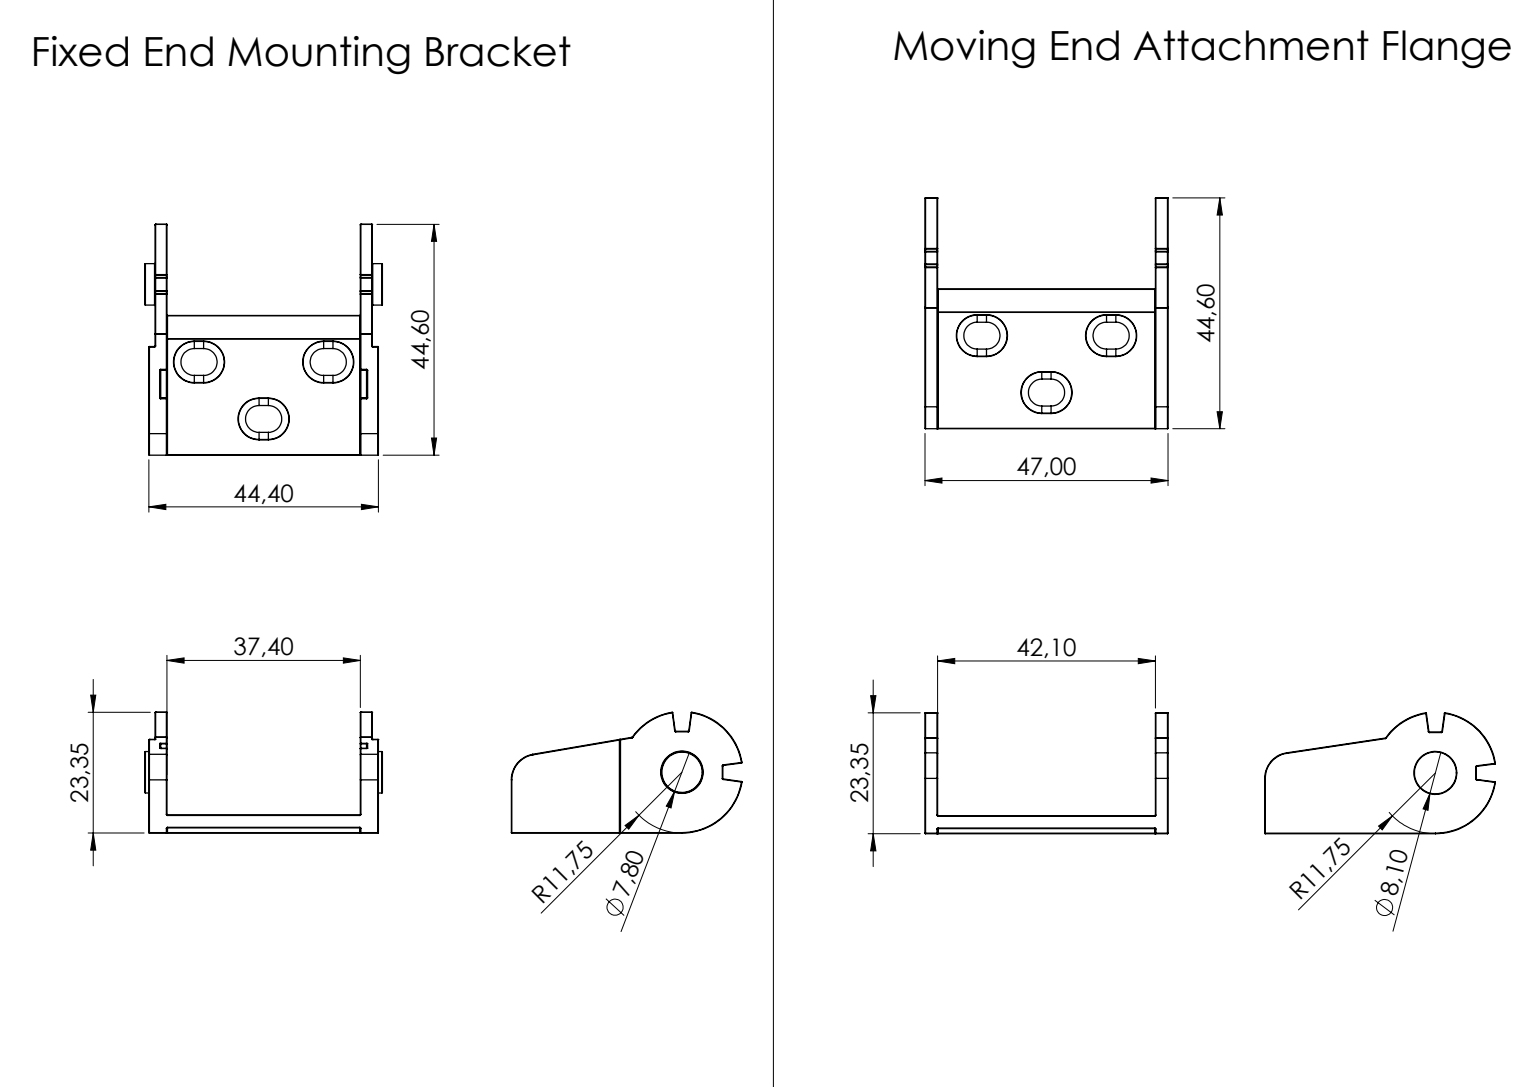
ISO-10303-21;
HEADER;
FILE_DESCRIPTION (('STEP AP214'),
    '1' );
FILE_NAME ('Moving End Attachment Flange.step',
    '2026-10-08T22:59:04',
    ( '' ),
    ( '' ),
    'SwSTEP 2.0',
    'SolidWorks 2020',
    '' );
FILE_SCHEMA (( 'AUTOMOTIVE_DESIGN' ));
ENDSEC;

DATA;
#58=DIRECTION ( 'NONE',  ( 1.000000000000000000, 0.000000000000000000, 0.000000000000000000 ) ) ;
#65=DIRECTION ( 'NONE',  ( -1.000000000000000000, 0.000000000000000000, 0.000000000000000000 ) ) ;
#86=AXIS2_PLACEMENT_3D ( 'NONE', #170578, #248783, #191400 ) ;
#130=ORIENTED_EDGE ( 'NONE', *, *, #78727, .F. ) ;
#161=CARTESIAN_POINT ( 'NONE',  ( 21.15000000000003055, 74.83745509109094485, -44.02310748452479316 ) ) ;
#188=FACE_OUTER_BOUND ( 'NONE', #64548, .T. ) ;
#229=AXIS2_PLACEMENT_3D ( 'NONE', #181398, #200936, #217905 ) ;
#283=DIRECTION ( 'NONE',  ( 1.000000000000000000, -0.000000000000000000, -0.000000000000000000 ) ) ;
#297=VERTEX_POINT ( 'NONE', #114542 ) ;
#298=DIRECTION ( 'NONE',  ( 0.000000000000000000, -0.9910827722268049644, -0.1332476588733589040 ) ) ;
#305=AXIS2_PLACEMENT_3D ( 'NONE', #200096, #237928, #219641 ) ;
#313=LINE ( 'NONE', #160718, #74675 ) ;
#317=ORIENTED_EDGE ( 'NONE', *, *, #114958, .T. ) ;
#423=CARTESIAN_POINT ( 'NONE',  ( 23.50000000000005684, 64.35000000001120668, -36.02310748452479316 ) ) ;
#432=ORIENTED_EDGE ( 'NONE', *, *, #190307, .F. ) ;
#508=AXIS2_PLACEMENT_3D ( 'NONE', #214942, #57126, #117135 ) ;
#514=VERTEX_POINT ( 'NONE', #110365 ) ;
#591=DIRECTION ( 'NONE',  ( 0.000000000000000000, -0.000000000000000000, 1.000000000000000000 ) ) ;
#608=DIRECTION ( 'NONE',  ( -1.000000000000000000, 0.000000000000000000, 0.000000000000000000 ) ) ;
#681=DIRECTION ( 'NONE',  ( 1.000000000000000000, -0.000000000000000000, -0.000000000000000000 ) ) ;
#684=DIRECTION ( 'NONE',  ( -1.000000000000000000, 0.000000000000000000, 0.000000000000000000 ) ) ;
#692=VECTOR ( 'NONE', #235400, 1000.000000000000114 ) ;
#719=EDGE_CURVE ( 'NONE', #17064, #33613, #92090, .T. ) ;
#745=FACE_OUTER_BOUND ( 'NONE', #98219, .T. ) ;
#767=ORIENTED_EDGE ( 'NONE', *, *, #253164, .T. ) ;
#781=CARTESIAN_POINT ( 'NONE',  ( 21.05000000000003979, 77.26165318615413469, -44.00978271863746016 ) ) ;
#784=CARTESIAN_POINT ( 'NONE',  ( 21.15000000000005187, 82.72707916847673459, -26.51159310135756897 ) ) ;
#789=CIRCLE ( 'NONE', #92397, 0.09999999999999939493 ) ;
#846=DIRECTION ( 'NONE',  ( 0.000000000000000000, 0.000000000000000000, 1.000000000000000000 ) ) ;
#874=DIRECTION ( 'NONE',  ( 0.000000000000000000, -1.000000000000000000, 0.000000000000000000 ) ) ;
#877=FACE_OUTER_BOUND ( 'NONE', #241147, .T. ) ;
#885=AXIS2_PLACEMENT_3D ( 'NONE', #13789, #95876, #252376 ) ;
#899=CARTESIAN_POINT ( 'NONE',  ( -23.49999999999994316, 74.83745509109094485, -44.02310748452479316 ) ) ;
#911=CARTESIAN_POINT ( 'NONE',  ( -23.39999999999994529, 84.00000000001119815, -37.18565239344504647 ) ) ;
#1008=AXIS2_PLACEMENT_3D ( 'NONE', #183384, #165097, #242056 ) ;
#1064=CARTESIAN_POINT ( 'NONE',  ( -23.49999999999994316, 83.80000000001119531, -34.86056257560453986 ) ) ;
#1099=DIRECTION ( 'NONE',  ( 0.000000000000000000, 0.000000000000000000, -1.000000000000000000 ) ) ;
#1101=DIRECTION ( 'NONE',  ( 0.000000000000000000, -0.9910827722268055195, 0.1332476588733540468 ) ) ;
#1121=EDGE_LOOP ( 'NONE', ( #113054, #182674, #33801, #198627 ) ) ;
#1192=CARTESIAN_POINT ( 'NONE',  ( 13.40000000000005898, 67.72071067812984779, -17.05239680640613997 ) ) ;
#1199=CARTESIAN_POINT ( 'NONE',  ( -20.94999999999994600, 65.25000000001119815, -51.02310748452479316 ) ) ;
#1262=EDGE_CURVE ( 'NONE', #252143, #114575, #242463, .T. ) ;
#1303=EDGE_LOOP ( 'NONE', ( #252309, #196137, #144068, #151074 ) ) ;
#1338=EDGE_CURVE ( 'NONE', #144177, #154033, #211118, .T. ) ;
#1363=CARTESIAN_POINT ( 'NONE',  ( 21.05000000000005400, 76.00000000001119815, -36.02310748452479316 ) ) ;
#1390=DIRECTION ( 'NONE',  ( -1.070660780358590712E-14, 0.9875102702516478370, -0.1575546449569727447 ) ) ;
#1441=EDGE_LOOP ( 'NONE', ( #100065, #27139, #58016, #75040 ) ) ;
#1472=LINE ( 'NONE', #118882, #221495 ) ;
#1480=DIRECTION ( 'NONE',  ( 1.000000000000000000, 0.000000000000000000, 0.000000000000000000 ) ) ;
#1489=ORIENTED_EDGE ( 'NONE', *, *, #175669, .F. ) ;
#1495=CARTESIAN_POINT ( 'NONE',  ( -20.94999999999994600, 66.25000000001114131, -51.02310748452476474 ) ) ;
#1569=VERTEX_POINT ( 'NONE', #161428 ) ;
#1588=LINE ( 'NONE', #141126, #111848 ) ;
#1647=DIRECTION ( 'NONE',  ( -0.000000000000000000, 1.000000000000000000, -0.000000000000000000 ) ) ;
#1657=VERTEX_POINT ( 'NONE', #70031 ) ;
#1673=EDGE_CURVE ( 'NONE', #28383, #222419, #249930, .T. ) ;
#1721=ORIENTED_EDGE ( 'NONE', *, *, #167214, .T. ) ;
#1726=AXIS2_PLACEMENT_3D ( 'NONE', #171029, #167159, #68024 ) ;
#1753=EDGE_CURVE ( 'NONE', #216962, #117682, #84575, .T. ) ;
#1769=EDGE_CURVE ( 'NONE', #179303, #61312, #15179, .T. ) ;
#1838=FACE_OUTER_BOUND ( 'NONE', #225196, .T. ) ;
#1881=CIRCLE ( 'NONE', #139248, 11.74999999999999645 ) ;
#1900=CYLINDRICAL_SURFACE ( 'NONE', #133191, 0.1000000000000028644 ) ;
#1940=ADVANCED_FACE ( 'NONE', ( #127099 ), #187100, .F. ) ;
#1952=ORIENTED_EDGE ( 'NONE', *, *, #205499, .F. ) ;
#2003=CARTESIAN_POINT ( 'NONE',  ( -23.49999999999994316, 64.35000000001120668, -29.92310748452479174 ) ) ;
#2010=ORIENTED_EDGE ( 'NONE', *, *, #13983, .T. ) ;
#2069=ORIENTED_EDGE ( 'NONE', *, *, #253484, .F. ) ;
#2123=DIRECTION ( 'NONE',  ( 0.000000000000000000, 0.000000000000000000, 1.000000000000000000 ) ) ;
#2254=EDGE_LOOP ( 'NONE', ( #136794, #52446, #245311, #24312 ) ) ;
#2289=EDGE_CURVE ( 'NONE', #178217, #49193, #223313, .T. ) ;
#2316=ORIENTED_EDGE ( 'NONE', *, *, #26990, .T. ) ;
#2337=ORIENTED_EDGE ( 'NONE', *, *, #212153, .F. ) ;
#2346=ORIENTED_EDGE ( 'NONE', *, *, #179917, .F. ) ;
#2425=AXIS2_PLACEMENT_3D ( 'NONE', #153513, #135160, #16531 ) ;
#2429=AXIS2_PLACEMENT_3D ( 'NONE', #151127, #230663, #191554 ) ;
#2432=CARTESIAN_POINT ( 'NONE',  ( -20.94999999999994600, 64.35000000001120668, -30.12310748452479103 ) ) ;
#2437=EDGE_CURVE ( 'NONE', #105984, #249805, #159645, .T. ) ;
#2510=CARTESIAN_POINT ( 'NONE',  ( -21.04999999999994387, 67.75000000001118394, -51.02310748452479316 ) ) ;
#2533=ORIENTED_EDGE ( 'NONE', *, *, #140585, .F. ) ;
#2552=DIRECTION ( 'NONE',  ( -1.000000000000000000, 0.000000000000000000, 0.000000000000000000 ) ) ;
#2571=DIRECTION ( 'NONE',  ( 0.000000000000000000, -1.000000000000000000, 0.000000000000000000 ) ) ;
#2592=ORIENTED_EDGE ( 'NONE', *, *, #199882, .F. ) ;
#2628=ADVANCED_FACE ( 'NONE', ( #243589 ), #18362, .F. ) ;
#2667=ORIENTED_EDGE ( 'NONE', *, *, #152205, .F. ) ;
#2698=ORIENTED_EDGE ( 'NONE', *, *, #100935, .F. ) ;
#2707=ORIENTED_EDGE ( 'NONE', *, *, #230430, .F. ) ;
#2770=ADVANCED_FACE ( 'NONE', ( #12709, #51783 ), #92205, .T. ) ;
#2806=PLANE ( 'NONE',  #25318 ) ;
#2812=EDGE_CURVE ( 'NONE', #113855, #9346, #20397, .T. ) ;
#2871=CARTESIAN_POINT ( 'NONE',  ( 21.05000000000005400, 74.16448838626246243, -47.52760213295649550 ) ) ;
#2911=AXIS2_PLACEMENT_3D ( 'NONE', #169962, #13421, #155523 ) ;
#2954=AXIS2_PLACEMENT_3D ( 'NONE', #224651, #164695, #167289 ) ;
#2988=AXIS2_PLACEMENT_3D ( 'NONE', #69678, #65800, #146600 ) ;
#3026=FACE_OUTER_BOUND ( 'NONE', #56842, .T. ) ;
#3089=EDGE_CURVE ( 'NONE', #24547, #60636, #101713, .T. ) ;
#3099=ORIENTED_EDGE ( 'NONE', *, *, #152190, .T. ) ;
#3110=LINE ( 'NONE', #183067, #153785 ) ;
#3143=DIRECTION ( 'NONE',  ( 0.000000000000000000, 0.000000000000000000, 1.000000000000000000 ) ) ;
#3193=CARTESIAN_POINT ( 'NONE',  ( -23.49999999999994316, 64.25000000001119815, -21.92310748452479174 ) ) ;
#3251=AXIS2_PLACEMENT_3D ( 'NONE', #102544, #214215, #195948 ) ;
#3256=DIRECTION ( 'NONE',  ( 1.000000000000000000, -0.000000000000000000, 0.000000000000000000 ) ) ;
#3259=VERTEX_POINT ( 'NONE', #80009 ) ;
#3263=CARTESIAN_POINT ( 'NONE',  ( -23.49999999999994316, 77.16254490893143725, -44.02310748452479316 ) ) ;
#3291=EDGE_LOOP ( 'NONE', ( #132921, #218359, #207662, #185863 ) ) ;
#3403=CARTESIAN_POINT ( 'NONE',  ( 21.15000000000005187, 83.90000000001120384, -37.27310748452479316 ) ) ;
#3418=ORIENTED_EDGE ( 'NONE', *, *, #5501, .T. ) ;
#3438=CARTESIAN_POINT ( 'NONE',  ( 6.000000000000061284, 64.65000000001120384, -22.12310748452479103 ) ) ;
#3443=EDGE_CURVE ( 'NONE', #226270, #123360, #243570, .T. ) ;
#3454=DIRECTION ( 'NONE',  ( 0.000000000000000000, 0.1332476588733589318, 0.9910827722268049644 ) ) ;
#3486=CIRCLE ( 'NONE', #149273, 0.1000000000000045852 ) ;
#3565=ORIENTED_EDGE ( 'NONE', *, *, #6376, .T. ) ;
#3574=EDGE_CURVE ( 'NONE', #35839, #131459, #32963, .T. ) ;
#3588=CARTESIAN_POINT ( 'NONE',  ( -23.49999999999994316, 82.84256550613280012, -26.34830530078816935 ) ) ;
#3592=VERTEX_POINT ( 'NONE', #115024 ) ;
#3598=CARTESIAN_POINT ( 'NONE',  ( 20.95000000000005258, 65.15000000001120384, -51.02310748452479316 ) ) ;
#3668=CARTESIAN_POINT ( 'NONE',  ( 5.551115123125782702E-14, 64.75000000001119815, -36.02310748452479316 ) ) ;
#3706=DIRECTION ( 'NONE',  ( 0.000000000000000000, -0.9910827722268055195, -0.1332476588733540468 ) ) ;
#3757=CARTESIAN_POINT ( 'NONE',  ( -20.94999999999994600, 65.15000000001120384, -3.123107484524795474 ) ) ;
#3786=CARTESIAN_POINT ( 'NONE',  ( 21.05000000000005400, 64.25000000001119815, -29.92310748452479174 ) ) ;
#3817=ORIENTED_EDGE ( 'NONE', *, *, #192515, .F. ) ;
#3832=CIRCLE ( 'NONE', #182907, 4.041421356237310469 ) ;
#3842=CIRCLE ( 'NONE', #241184, 0.09999999999999982514 ) ;
#3861=DIRECTION ( 'NONE',  ( 0.000000000000000000, 0.000000000000000000, -1.000000000000000000 ) ) ;
#3897=AXIS2_PLACEMENT_3D ( 'NONE', #95566, #57713, #237656 ) ;
#3941=ORIENTED_EDGE ( 'NONE', *, *, #226784, .F. ) ;
#4014=ADVANCED_FACE ( 'NONE', ( #179523 ), #139050, .T. ) ;
#4017=ORIENTED_EDGE ( 'NONE', *, *, #162333, .F. ) ;
#4045=CYLINDRICAL_SURFACE ( 'NONE', #163268, 0.09999999999999939493 ) ;
#4077=AXIS2_PLACEMENT_3D ( 'NONE', #31474, #53573, #110979 ) ;
#4093=DIRECTION ( 'NONE',  ( 0.000000000000000000, 0.000000000000000000, -1.000000000000000000 ) ) ;
#4096=AXIS2_PLACEMENT_3D ( 'NONE', #226436, #206904, #28301 ) ;
#4129=ORIENTED_EDGE ( 'NONE', *, *, #11231, .F. ) ;
#4148=CIRCLE ( 'NONE', #145598, 0.09999999999999939493 ) ;
#4156=CARTESIAN_POINT ( 'NONE',  ( 20.95000000000005613, 66.15000000001120384, -5.923107484524795296 ) ) ;
#4160=DIRECTION ( 'NONE',  ( 1.000000000000000000, 0.000000000000000000, 0.000000000000000000 ) ) ;
#4165=AXIS2_PLACEMENT_3D ( 'NONE', #175488, #100708, #155931 ) ;
#4169=DIRECTION ( 'NONE',  ( 0.000000000000000000, 0.000000000000000000, 1.000000000000000000 ) ) ;
#4170=DIRECTION ( 'NONE',  ( 0.000000000000000000, 0.000000000000000000, 1.000000000000000000 ) ) ;
#4173=ORIENTED_EDGE ( 'NONE', *, *, #60970, .F. ) ;
#4191=CIRCLE ( 'NONE', #204094, 0.09999999999999635569 ) ;
#4262=AXIS2_PLACEMENT_3D ( 'NONE', #181726, #124322, #42219 ) ;
#4289=CARTESIAN_POINT ( 'NONE',  ( -23.39999999999994529, 82.64476912853859858, -26.37791261425322986 ) ) ;
#4299=ORIENTED_EDGE ( 'NONE', *, *, #222834, .F. ) ;
#4303=EDGE_LOOP ( 'NONE', ( #202943, #2316, #5119, #203165, #34482, #231347, #128376, #168284, #195736, #122157, #112154, #131721, #69827, #42740, #256729, #184778, #204213, #171842 ) ) ;
#4333=DIRECTION ( 'NONE',  ( 0.000000000000000000, -0.1480365673253065117, 0.9889818879709274535 ) ) ;
#4335=CIRCLE ( 'NONE', #125175, 0.1999999999999987899 ) ;
#4427=LINE ( 'NONE', #245626, #204503 ) ;
#4449=EDGE_CURVE ( 'NONE', #168532, #177623, #63085, .T. ) ;
#4530=DIRECTION ( 'NONE',  ( 1.000000000000000000, 0.000000000000000000, 0.000000000000000000 ) ) ;
#4591=CARTESIAN_POINT ( 'NONE',  ( -21.14999999999994174, 76.00000000001119815, -36.02310748452479316 ) ) ;
#4593=DIRECTION ( 'NONE',  ( -1.000000000000000000, 0.000000000000000000, 0.000000000000000000 ) ) ;
#4675=AXIS2_PLACEMENT_3D ( 'NONE', #54422, #132692, #33632 ) ;
#4691=DIRECTION ( 'NONE',  ( -0.000000000000000000, -1.000000000000000000, 0.000000000000000000 ) ) ;
#4782=CIRCLE ( 'NONE', #221456, 0.09999999999999635569 ) ;
#4787=CARTESIAN_POINT ( 'NONE',  ( -21.14999999999994174, 83.90000000001120384, -34.77310748452479316 ) ) ;
#4835=CIRCLE ( 'NONE', #79679, 0.1000000000000021844 ) ;
#4914=CARTESIAN_POINT ( 'NONE',  ( -23.39999999999994529, 77.16254490893143725, -43.82310748452479743 ) ) ;
#5000=DIRECTION ( 'NONE',  ( 0.000000000000000000, 0.1480365673253065117, -0.9889818879709273425 ) ) ;
#5019=CARTESIAN_POINT ( 'NONE',  ( -21.14999999999994174, 87.51781941433023349, -37.75951082105083145 ) ) ;
#5026=DIRECTION ( 'NONE',  ( -0.000000000000000000, 0.000000000000000000, 1.000000000000000000 ) ) ;
#5035=DIRECTION ( 'NONE',  ( -1.284434275755705296E-16, 0.7071067811865471286, -0.7071067811865479058 ) ) ;
#5048=DIRECTION ( 'NONE',  ( 1.000000000000000000, 0.000000000000000000, 0.000000000000000000 ) ) ;
#5067=LINE ( 'NONE', #45514, #195066 ) ;
#5119=ORIENTED_EDGE ( 'NONE', *, *, #1753, .F. ) ;
#5137=DIRECTION ( 'NONE',  ( 1.000000000000000000, 0.000000000000000000, 0.000000000000000000 ) ) ;
#5177=DIRECTION ( 'NONE',  ( 0.000000000000000000, 0.000000000000000000, 1.000000000000000000 ) ) ;
#5205=AXIS2_PLACEMENT_3D ( 'NONE', #2510, #202017, #20831 ) ;
#5207=VERTEX_POINT ( 'NONE', #162901 ) ;
#5251=DIRECTION ( 'NONE',  ( 1.000000000000000000, 0.000000000000000000, 0.000000000000000000 ) ) ;
#5309=CARTESIAN_POINT ( 'NONE',  ( -13.39999999999994529, 64.35000000001120668, -18.32310748452479388 ) ) ;
#5311=DIRECTION ( 'NONE',  ( 0.000000000000000000, 1.000000000000000000, 0.000000000000000000 ) ) ;
#5356=ORIENTED_EDGE ( 'NONE', *, *, #92045, .T. ) ;
#5376=ORIENTED_EDGE ( 'NONE', *, *, #101397, .F. ) ;
#5436=ORIENTED_EDGE ( 'NONE', *, *, #13960, .T. ) ;
#5487=VECTOR ( 'NONE', #95802, 1000.000000000000000 ) ;
#5491=ORIENTED_EDGE ( 'NONE', *, *, #140323, .T. ) ;
#5501=EDGE_CURVE ( 'NONE', #118363, #143932, #44230, .T. ) ;
#5523=ORIENTED_EDGE ( 'NONE', *, *, #39101, .F. ) ;
#5527=ORIENTED_EDGE ( 'NONE', *, *, #208102, .F. ) ;
#5534=EDGE_CURVE ( 'NONE', #81245, #109039, #143949, .T. ) ;
#5588=AXIS2_PLACEMENT_3D ( 'NONE', #65713, #188233, #109969 ) ;
#5596=DIRECTION ( 'NONE',  ( 0.000000000000000000, 0.000000000000000000, 1.000000000000000000 ) ) ;
#5681=ORIENTED_EDGE ( 'NONE', *, *, #75557, .T. ) ;
#5698=ORIENTED_EDGE ( 'NONE', *, *, #205981, .F. ) ;
#5797=EDGE_LOOP ( 'NONE', ( #16794, #21298, #95358, #113360 ) ) ;
#5858=CIRCLE ( 'NONE', #30852, 0.09999999999999939493 ) ;
#5874=CARTESIAN_POINT ( 'NONE',  ( -5.899999999999938183, 64.65000000001120384, -22.12310748452479103 ) ) ;
#5887=VECTOR ( 'NONE', #138797, 1000.000000000000000 ) ;
#5945=ORIENTED_EDGE ( 'NONE', *, *, #220027, .F. ) ;
#5948=CARTESIAN_POINT ( 'NONE',  ( 11.60000000000006182, 66.35000000001119247, -18.42310748452479530 ) ) ;
#6019=ORIENTED_EDGE ( 'NONE', *, *, #64587, .T. ) ;
#6034=DIRECTION ( 'NONE',  ( 1.000000000000000000, 0.000000000000000000, 0.000000000000000000 ) ) ;
#6060=DIRECTION ( 'NONE',  ( 3.469446951953515108E-14, 0.000000000000000000, 1.000000000000000000 ) ) ;
#6077=AXIS2_PLACEMENT_3D ( 'NONE', #129564, #249515, #126983 ) ;
#6102=CARTESIAN_POINT ( 'NONE',  ( 20.95000000000005969, 61.72892516158560028, -36.56695479651062897 ) ) ;
#6134=EDGE_CURVE ( 'NONE', #166555, #204034, #173245, .T. ) ;
#6163=LINE ( 'NONE', #129650, #109600 ) ;
#6179=ORIENTED_EDGE ( 'NONE', *, *, #223678, .F. ) ;
#6253=EDGE_CURVE ( 'NONE', #109234, #200341, #151252, .T. ) ;
#6254=ORIENTED_EDGE ( 'NONE', *, *, #244093, .T. ) ;
#6284=CARTESIAN_POINT ( 'NONE',  ( -21.04999999999994387, 67.75000000001118394, -3.123107484524795474 ) ) ;
#6318=CARTESIAN_POINT ( 'NONE',  ( -23.49999999999994316, 83.90000000001120384, -34.77310748452479316 ) ) ;
#6339=CARTESIAN_POINT ( 'NONE',  ( -23.49999999999994316, 77.83551161375991967, -47.52760213295649550 ) ) ;
#6376=EDGE_CURVE ( 'NONE', #131459, #210784, #186243, .T. ) ;
#6397=FACE_OUTER_BOUND ( 'NONE', #98533, .T. ) ;
#6464=FACE_OUTER_BOUND ( 'NONE', #103057, .T. ) ;
#6487=VERTEX_POINT ( 'NONE', #119836 ) ;
#6491=EDGE_CURVE ( 'NONE', #88642, #28434, #23384, .T. ) ;
#6566=CIRCLE ( 'NONE', #102390, 0.1000000000000028644 ) ;
#6567=CARTESIAN_POINT ( 'NONE',  ( -23.49999999999994316, 87.50449464844290048, -37.85861909827351468 ) ) ;
#6577=ORIENTED_EDGE ( 'NONE', *, *, #18649, .T. ) ;
#6652=SPHERICAL_SURFACE ( 'NONE', #72367, 0.1000000000000000056 ) ;
#6663=CARTESIAN_POINT ( 'NONE',  ( -23.49999999999994316, 77.73640333653723644, -47.54092689884382850 ) ) ;
#6726=AXIS2_PLACEMENT_3D ( 'NONE', #63550, #141802, #183513 ) ;
#6800=VECTOR ( 'NONE', #177965, 1000.000000000000000 ) ;
#6839=ORIENTED_EDGE ( 'NONE', *, *, #254228, .F. ) ;
#6859=CARTESIAN_POINT ( 'NONE',  ( -13.39999999999994351, 64.25000000001119815, -23.72310748452479245 ) ) ;
#6881=LINE ( 'NONE', #186825, #76412 ) ;
#6904=CARTESIAN_POINT ( 'NONE',  ( 21.15000000000005187, 64.25000000001119815, -36.02310748452479316 ) ) ;
#6932=ORIENTED_EDGE ( 'NONE', *, *, #243618, .F. ) ;
#6944=ORIENTED_EDGE ( 'NONE', *, *, #59147, .T. ) ;
#6947=ORIENTED_EDGE ( 'NONE', *, *, #242302, .T. ) ;
#6953=VERTEX_POINT ( 'NONE', #104705 ) ;
#6987=DIRECTION ( 'NONE',  ( 0.000000000000000000, 1.000000000000000000, -1.224646799147352961E-16 ) ) ;
#7009=DIRECTION ( 'NONE',  ( 0.000000000000000000, 0.000000000000000000, 1.000000000000000000 ) ) ;
#7097=CARTESIAN_POINT ( 'NONE',  ( -23.49999999999994316, 89.48413628383013929, -38.12477508515532065 ) ) ;
#7122=AXIS2_PLACEMENT_3D ( 'NONE', #137369, #257277, #96934 ) ;
#7186=ADVANCED_FACE ( 'NONE', ( #238827 ), #58872, .T. ) ;
#7195=ADVANCED_FACE ( 'NONE', ( #120200 ), #15957, .T. ) ;
#7211=FACE_OUTER_BOUND ( 'NONE', #182132, .T. ) ;
#7234=CARTESIAN_POINT ( 'NONE',  ( 23.40000000000005542, 64.25000000001119815, -43.82310748452479743 ) ) ;
#7255=ORIENTED_EDGE ( 'NONE', *, *, #152151, .F. ) ;
#7370=LINE ( 'NONE', #204278, #172996 ) ;
#7377=ORIENTED_EDGE ( 'NONE', *, *, #142662, .F. ) ;
#7384=CIRCLE ( 'NONE', #153185, 0.09999999999999939493 ) ;
#7407=CARTESIAN_POINT ( 'NONE',  ( 21.05000000000005400, 79.78873604695631627, -7.297728304630792806 ) ) ;
#7463=ORIENTED_EDGE ( 'NONE', *, *, #65270, .T. ) ;
#7555=FACE_OUTER_BOUND ( 'NONE', #97491, .T. ) ;
#7567=ORIENTED_EDGE ( 'NONE', *, *, #44290, .T. ) ;
#7576=AXIS2_PLACEMENT_3D ( 'NONE', #228645, #26588, #203917 ) ;
#7626=DIRECTION ( 'NONE',  ( 0.000000000000000000, 0.1332476588733448597, 0.9910827722268067408 ) ) ;
#7661=AXIS2_PLACEMENT_3D ( 'NONE', #125665, #87803, #167395 ) ;
#7714=TOROIDAL_SURFACE ( 'NONE', #20182, 4.150000000000000355, 0.1000000000000000056 ) ;
#7804=CARTESIAN_POINT ( 'NONE',  ( -21.14999999999994174, 76.00000000001119815, -36.02310748452479316 ) ) ;
#7807=DIRECTION ( 'NONE',  ( -1.000000000000000000, 0.000000000000000000, 0.000000000000000000 ) ) ;
#7832=ORIENTED_EDGE ( 'NONE', *, *, #196051, .F. ) ;
#7836=ADVANCED_FACE ( 'NONE', ( #182412 ), #132225, .T. ) ;
#7879=ORIENTED_EDGE ( 'NONE', *, *, #155408, .F. ) ;
#7893=DIRECTION ( 'NONE',  ( -1.000000000000000000, -0.000000000000000000, -0.000000000000000000 ) ) ;
#7939=CARTESIAN_POINT ( 'NONE',  ( 5.900000000000059863, 64.65000000001120384, -25.92310748452479174 ) ) ;
#7988=VECTOR ( 'NONE', #37090, 1000.000000000000114 ) ;
#7990=ADVANCED_FACE ( 'NONE', ( #176985 ), #53150, .F. ) ;
#8064=CARTESIAN_POINT ( 'NONE',  ( 6.000000000000060396, 64.25000000001119815, -25.92310748452479174 ) ) ;
#8187=DIRECTION ( 'NONE',  ( 0.000000000000000000, 0.000000000000000000, -1.000000000000000000 ) ) ;
#8191=DIRECTION ( 'NONE',  ( 1.000000000000000000, -0.000000000000000000, -0.000000000000000000 ) ) ;
#8217=VERTEX_POINT ( 'NONE', #48989 ) ;
#8218=SHAPE_REPRESENTATION_RELATIONSHIP ( 'NONE' , 'NONE' ,  #133560, #200717 ) ;
#8249=ORIENTED_EDGE ( 'NONE', *, *, #204291, .F. ) ;
#8251=ORIENTED_EDGE ( 'NONE', *, *, #19825, .F. ) ;
#8336=CIRCLE ( 'NONE', #154110, 4.041421356237310469 ) ;
#8399=FACE_OUTER_BOUND ( 'NONE', #57955, .T. ) ;
#8423=ORIENTED_EDGE ( 'NONE', *, *, #165404, .T. ) ;
#8429=FACE_OUTER_BOUND ( 'NONE', #91879, .T. ) ;
#8441=ORIENTED_EDGE ( 'NONE', *, *, #6376, .F. ) ;
#8457=AXIS2_PLACEMENT_3D ( 'NONE', #82873, #102439, #24248 ) ;
#8462=EDGE_LOOP ( 'NONE', ( #194088, #90251, #198660, #143089 ) ) ;
#8469=ORIENTED_EDGE ( 'NONE', *, *, #62876, .F. ) ;
#8539=DIRECTION ( 'NONE',  ( 0.000000000000000000, 2.775557561562812086E-13, 1.000000000000000000 ) ) ;
#8561=CIRCLE ( 'NONE', #16952, 0.1000000000000021844 ) ;
#8569=DIRECTION ( 'NONE',  ( 0.000000000000000000, 0.000000000000000000, 1.000000000000000000 ) ) ;
#8584=CARTESIAN_POINT ( 'NONE',  ( 21.05000000000005400, 82.72707916847673459, -26.51159310135756897 ) ) ;
#8596=CARTESIAN_POINT ( 'NONE',  ( -23.49999999999994316, 77.85126707825561709, -47.62635315998165453 ) ) ;
#8652=CARTESIAN_POINT ( 'NONE',  ( -13.39999999999994529, 67.65000000001118963, -16.98168612828748181 ) ) ;
#8670=CARTESIAN_POINT ( 'NONE',  ( -21.04999999999994387, 87.50449464844290048, -34.18759587077607165 ) ) ;
#8675=DIRECTION ( 'NONE',  ( -1.000000000000000000, 0.000000000000000000, 0.000000000000000000 ) ) ;
#8676=ORIENTED_EDGE ( 'NONE', *, *, #190134, .F. ) ;
#8683=FACE_OUTER_BOUND ( 'NONE', #14893, .T. ) ;
#8784=ORIENTED_EDGE ( 'NONE', *, *, #137079, .T. ) ;
#8835=ORIENTED_EDGE ( 'NONE', *, *, #46738, .T. ) ;
#8920=AXIS2_PLACEMENT_3D ( 'NONE', #232601, #90481, #248284 ) ;
#8939=LINE ( 'NONE', #164169, #155031 ) ;
#8971=CARTESIAN_POINT ( 'NONE',  ( 21.05000000000005400, 67.65000000001118963, -25.06452884076209742 ) ) ;
#8988=ORIENTED_EDGE ( 'NONE', *, *, #141241, .T. ) ;
#9117=EDGE_LOOP ( 'NONE', ( #16086, #23583, #36112, #191588 ) ) ;
#9165=CARTESIAN_POINT ( 'NONE',  ( -5.999999999999938716, 64.75000000001119815, -25.92310748452479174 ) ) ;
#9189=CIRCLE ( 'NONE', #217443, 0.1000000000000028644 ) ;
#9211=AXIS2_PLACEMENT_3D ( 'NONE', #172868, #77537, #257425 ) ;
#9233=ORIENTED_EDGE ( 'NONE', *, *, #179815, .T. ) ;
#9244=SPHERICAL_SURFACE ( 'NONE', #225558, 0.1000000000000000056 ) ;
#9290=ORIENTED_EDGE ( 'NONE', *, *, #13159, .T. ) ;
#9297=FACE_OUTER_BOUND ( 'NONE', #214035, .T. ) ;
#9304=DIRECTION ( 'NONE',  ( -0.000000000000000000, 0.9910827722268037432, 0.1332476588733682299 ) ) ;
#9319=CYLINDRICAL_SURFACE ( 'NONE', #147477, 0.09999999999999982514 ) ;
#9334=ADVANCED_FACE ( 'NONE', ( #163857, #162586 ), #99990, .T. ) ;
#9346=VERTEX_POINT ( 'NONE', #183421 ) ;
#9371=CARTESIAN_POINT ( 'NONE',  ( -23.39999999999994529, 64.25000000001119815, -36.02310748452479316 ) ) ;
#9389=VERTEX_POINT ( 'NONE', #127292 ) ;
#9410=ORIENTED_EDGE ( 'NONE', *, *, #246327, .F. ) ;
#9439=DIRECTION ( 'NONE',  ( 0.000000000000000000, 0.9910827722268042983, 0.1332476588733650935 ) ) ;
#9468=AXIS2_PLACEMENT_3D ( 'NONE', #110669, #72861, #148520 ) ;
#9479=ORIENTED_EDGE ( 'NONE', *, *, #226367, .T. ) ;
#9491=DIRECTION ( 'NONE',  ( 1.000000000000000000, 0.000000000000000000, 0.000000000000000000 ) ) ;
#9494=CARTESIAN_POINT ( 'NONE',  ( -40.23850191057533010, 61.64150943397345372, -36.51839050339276582 ) ) ;
#9533=ORIENTED_EDGE ( 'NONE', *, *, #49799, .T. ) ;
#9552=CARTESIAN_POINT ( 'NONE',  ( 23.50000000000005684, 84.00000000001119815, -34.86056257560453986 ) ) ;
#9575=CARTESIAN_POINT ( 'NONE',  ( -23.49999999999994316, 76.00000000001119815, -36.02310748452479316 ) ) ;
#9586=ORIENTED_EDGE ( 'NONE', *, *, #186080, .F. ) ;
#9589=DIRECTION ( 'NONE',  ( 0.000000000000000000, 0.9875102702516471709, 0.1575546449569757979 ) ) ;
#9621=CARTESIAN_POINT ( 'NONE',  ( 21.05000000000005400, 84.00000000001119815, -34.86056257560453986 ) ) ;
#9633=ORIENTED_EDGE ( 'NONE', *, *, #3443, .T. ) ;
#9637=EDGE_CURVE ( 'NONE', #143490, #186471, #124962, .T. ) ;
#9798=ORIENTED_EDGE ( 'NONE', *, *, #74787, .T. ) ;
#9836=TOROIDAL_SURFACE ( 'NONE', #147213, 0.2000000000000000111, 0.1000000000000000056 ) ;
#9838=ORIENTED_EDGE ( 'NONE', *, *, #147461, .F. ) ;
#9898=ORIENTED_EDGE ( 'NONE', *, *, #85489, .T. ) ;
#9937=CARTESIAN_POINT ( 'NONE',  ( -21.14999999999994174, 74.63923853664559260, -43.99645795275012006 ) ) ;
#10006=DIRECTION ( 'NONE',  ( 0.000000000000000000, 0.000000000000000000, -1.000000000000000000 ) ) ;
#10047=VERTEX_POINT ( 'NONE', #118902 ) ;
#10142=FACE_OUTER_BOUND ( 'NONE', #252352, .T. ) ;
#10157=VECTOR ( 'NONE', #85979, 1000.000000000000000 ) ;
#10224=CARTESIAN_POINT ( 'NONE',  ( -5.999999999999938716, 64.65000000001120384, -25.92310748452479174 ) ) ;
#10230=ORIENTED_EDGE ( 'NONE', *, *, #225434, .T. ) ;
#10234=CIRCLE ( 'NONE', #218863, 0.1000000000000032391 ) ;
#10258=CARTESIAN_POINT ( 'NONE',  ( 21.15000000000005542, 64.35000000001120668, -3.023107484524792277 ) ) ;
#10259=CARTESIAN_POINT ( 'NONE',  ( -21.14999999999994174, 77.25000000001119815, -43.92310748452479885 ) ) ;
#10282=VECTOR ( 'NONE', #105529, 1000.000000000000000 ) ;
#10351=CARTESIAN_POINT ( 'NONE',  ( -23.39999999999994529, 79.78873604695631627, -7.297728304630792806 ) ) ;
#10391=FACE_OUTER_BOUND ( 'NONE', #232579, .T. ) ;
#10448=ORIENTED_EDGE ( 'NONE', *, *, #61513, .F. ) ;
#10581=EDGE_CURVE ( 'NONE', #216036, #53024, #100773, .T. ) ;
#10605=VERTEX_POINT ( 'NONE', #5019 ) ;
#10610=EDGE_LOOP ( 'NONE', ( #69076, #190839, #236443, #253146 ) ) ;
#10848=DIRECTION ( 'NONE',  ( 0.000000000000000000, 0.000000000000000000, 1.000000000000000000 ) ) ;
#10888=PLANE ( 'NONE',  #186697 ) ;
#10915=CARTESIAN_POINT ( 'NONE',  ( -23.39999999999994529, 76.00000000001119815, -36.02310748452479316 ) ) ;
#10936=CARTESIAN_POINT ( 'NONE',  ( 21.15000000000005542, 83.97335046823651794, -37.38386894789040582 ) ) ;
#10948=DIRECTION ( 'NONE',  ( 0.000000000000000000, 0.000000000000000000, -1.000000000000000000 ) ) ;
#10959=ORIENTED_EDGE ( 'NONE', *, *, #249561, .F. ) ;
#10977=VECTOR ( 'NONE', #23732, 999.9999999999998863 ) ;
#11001=ADVANCED_FACE ( 'NONE', ( #85519 ), #245924, .T. ) ;
#11052=DIRECTION ( 'NONE',  ( 1.734723475976817823E-14, 1.000000000000000000, -0.000000000000000000 ) ) ;
#11068=ADVANCED_FACE ( 'NONE', ( #202934 ), #127255, .T. ) ;
#11093=ORIENTED_EDGE ( 'NONE', *, *, #257916, .T. ) ;
#11100=CYLINDRICAL_SURFACE ( 'NONE', #203103, 0.09999999999999939493 ) ;
#11109=VECTOR ( 'NONE', #240581, 1000.000000000000114 ) ;
#11165=DIRECTION ( 'NONE',  ( -3.469446951953515108E-14, 0.000000000000000000, -1.000000000000000000 ) ) ;
#11178=LINE ( 'NONE', #69885, #101275 ) ;
#11227=CARTESIAN_POINT ( 'NONE',  ( 21.05000000000005400, 76.00000000001119815, -36.02310748452479316 ) ) ;
#11231=EDGE_CURVE ( 'NONE', #49193, #147247, #254837, .T. ) ;
#11253=DIRECTION ( 'NONE',  ( -1.000000000000000000, 0.000000000000000000, -0.000000000000000000 ) ) ;
#11296=CARTESIAN_POINT ( 'NONE',  ( -40.23850191057533010, 67.65000000001118963, -25.49719488170504533 ) ) ;
#11488=CARTESIAN_POINT ( 'NONE',  ( 23.40000000000005542, 87.50449464844290048, -37.85861909827351468 ) ) ;
#11531=ORIENTED_EDGE ( 'NONE', *, *, #94855, .T. ) ;
#11539=DIRECTION ( 'NONE',  ( -0.000000000000000000, 0.1480365673253065117, -0.9889818879709273425 ) ) ;
#11638=CARTESIAN_POINT ( 'NONE',  ( -5.899999999999938183, 64.65000000001120384, -26.02310748452479316 ) ) ;
#11704=ORIENTED_EDGE ( 'NONE', *, *, #140585, .T. ) ;
#11710=DIRECTION ( 'NONE',  ( 0.000000000000000000, 1.000000000000000000, 0.000000000000000000 ) ) ;
#11717=ORIENTED_EDGE ( 'NONE', *, *, #152190, .F. ) ;
#11762=ADVANCED_FACE ( 'NONE', ( #45498 ), #46767, .T. ) ;
#11779=CIRCLE ( 'NONE', #174110, 2.699999999999999289 ) ;
#11786=ORIENTED_EDGE ( 'NONE', *, *, #250558, .T. ) ;
#11792=AXIS2_PLACEMENT_3D ( 'NONE', #47207, #146317, #126764 ) ;
#11824=AXIS2_PLACEMENT_3D ( 'NONE', #82317, #241436, #4093 ) ;
#11841=ORIENTED_EDGE ( 'NONE', *, *, #33972, .F. ) ;
#11846=DIRECTION ( 'NONE',  ( 0.000000000000000000, 2.775557561562812086E-13, 1.000000000000000000 ) ) ;
#11891=CIRCLE ( 'NONE', #207517, 0.09999999999999939493 ) ;
#11916=LINE ( 'NONE', #169724, #118260 ) ;
#11972=VERTEX_POINT ( 'NONE', #174491 ) ;
#11987=EDGE_LOOP ( 'NONE', ( #236841, #230235, #218852, #15222 ) ) ;
#11995=AXIS2_PLACEMENT_3D ( 'NONE', #94146, #254481, #172453 ) ;
#12025=EDGE_LOOP ( 'NONE', ( #138536, #106594, #133117, #116553 ) ) ;
#12036=ORIENTED_EDGE ( 'NONE', *, *, #42241, .F. ) ;
#12057=CARTESIAN_POINT ( 'NONE',  ( 21.05000000000005400, 87.75000000001119815, -43.82310748452479743 ) ) ;
#12090=CIRCLE ( 'NONE', #150118, 0.1000000000000028644 ) ;
#12117=CIRCLE ( 'NONE', #45402, 4.049999999999998046 ) ;
#12135=DIRECTION ( 'NONE',  ( 0.000000000000000000, 0.000000000000000000, -1.000000000000000000 ) ) ;
#12138=DIRECTION ( 'NONE',  ( 0.000000000000000000, 0.000000000000000000, 1.000000000000000000 ) ) ;
#12172=CARTESIAN_POINT ( 'NONE',  ( -23.49999999999994316, 76.00000000001119815, -31.87310748452479459 ) ) ;
#12178=DIRECTION ( 'NONE',  ( 1.000000000000000000, -0.000000000000000000, -0.000000000000000000 ) ) ;
#12197=VERTEX_POINT ( 'NONE', #88129 ) ;
#12214=VERTEX_POINT ( 'NONE', #105117 ) ;
#12239=EDGE_CURVE ( 'NONE', #35839, #74847, #89074, .T. ) ;
#12240=AXIS2_PLACEMENT_3D ( 'NONE', #105737, #223138, #44522 ) ;
#12281=PLANE ( 'NONE',  #68683 ) ;
#12282=DIRECTION ( 'NONE',  ( 0.000000000000000000, 0.000000000000000000, -1.000000000000000000 ) ) ;
#12360=EDGE_LOOP ( 'NONE', ( #119536, #155518, #179823 ) ) ;
#12388=DIRECTION ( 'NONE',  ( -1.000000000000000000, 0.000000000000000000, 0.000000000000000000 ) ) ;
#12524=CIRCLE ( 'NONE', #245736, 0.09999999999999939493 ) ;
#12539=VERTEX_POINT ( 'NONE', #87836 ) ;
#12634=ORIENTED_EDGE ( 'NONE', *, *, #33176, .T. ) ;
#12659=EDGE_CURVE ( 'NONE', #17064, #88829, #105988, .T. ) ;
#12665=ORIENTED_EDGE ( 'NONE', *, *, #236566, .F. ) ;
#12679=ORIENTED_EDGE ( 'NONE', *, *, #224280, .T. ) ;
#12682=ORIENTED_EDGE ( 'NONE', *, *, #24841, .T. ) ;
#12695=ADVANCED_FACE ( 'NONE', ( #248225 ), #229940, .T. ) ;
#12709=FACE_BOUND ( 'NONE', #159419, .T. ) ;
#12741=CARTESIAN_POINT ( 'NONE',  ( -20.94999999999994600, 64.35000000001120668, -30.02310748452479316 ) ) ;
#12755=LINE ( 'NONE', #210930, #212322 ) ;
#12764=CIRCLE ( 'NONE', #183430, 0.1000000000000028644 ) ;
#12771=CARTESIAN_POINT ( 'NONE',  ( 5.900000000000060751, 64.35000000001120668, -22.02310748452479316 ) ) ;
#12772=ORIENTED_EDGE ( 'NONE', *, *, #257916, .F. ) ;
#12805=DIRECTION ( 'NONE',  ( 0.000000000000000000, 1.000000000000000000, 0.000000000000000000 ) ) ;
#12851=AXIS2_PLACEMENT_3D ( 'NONE', #70539, #127920, #228307 ) ;
#12912=DIRECTION ( 'NONE',  ( 4.336808689942017736E-16, -0.000000000000000000, 1.000000000000000000 ) ) ;
#12936=AXIS2_PLACEMENT_3D ( 'NONE', #190065, #90955, #170556 ) ;
#12981=CARTESIAN_POINT ( 'NONE',  ( -20.94999999999994245, 67.85000000001119247, -51.02310748452479316 ) ) ;
#13015=DIRECTION ( 'NONE',  ( 0.000000000000000000, -0.1332476588733448597, -0.9910827722268067408 ) ) ;
#13048=DIRECTION ( 'NONE',  ( -0.000000000000000000, 1.000000000000000000, -0.000000000000000000 ) ) ;
#13087=DIRECTION ( 'NONE',  ( -1.000000000000000000, 0.000000000000000000, 0.000000000000000000 ) ) ;
#13122=ADVANCED_FACE ( 'NONE', ( #9297 ), #50966, .T. ) ;
#13148=CYLINDRICAL_SURFACE ( 'NONE', #232670, 0.09999999999999939493 ) ;
#13159=EDGE_CURVE ( 'NONE', #205114, #30110, #88858, .T. ) ;
#13224=CARTESIAN_POINT ( 'NONE',  ( -13.39999999999994351, 66.35000000001119247, -23.62310748452479103 ) ) ;
#13230=DIRECTION ( 'NONE',  ( -1.000000000000000000, 0.000000000000000000, 0.000000000000000000 ) ) ;
#13239=CARTESIAN_POINT ( 'NONE',  ( 21.15000000000005187, 82.84256550613280012, -26.34830530078816935 ) ) ;
#13264=ORIENTED_EDGE ( 'NONE', *, *, #147746, .F. ) ;
#13355=ORIENTED_EDGE ( 'NONE', *, *, #50686, .F. ) ;
#13376=CARTESIAN_POINT ( 'NONE',  ( -21.14999999999994174, 83.97335046823651794, -37.38386894789040582 ) ) ;
#13421=DIRECTION ( 'NONE',  ( 1.000000000000000000, -0.000000000000000000, -0.000000000000000000 ) ) ;
#13543=AXIS2_PLACEMENT_3D ( 'NONE', #96349, #152532, #175939 ) ;
#13662=DIRECTION ( 'NONE',  ( 0.000000000000000000, 0.000000000000000000, 1.000000000000000000 ) ) ;
#13672=CARTESIAN_POINT ( 'NONE',  ( 13.40000000000005898, 64.35000000001120668, -21.02310748452479316 ) ) ;
#13705=ORIENTED_EDGE ( 'NONE', *, *, #155750, .T. ) ;
#13752=DIRECTION ( 'NONE',  ( 1.000000000000000000, 0.000000000000000000, 0.000000000000000000 ) ) ;
#13756=VECTOR ( 'NONE', #184747, 1000.000000000000000 ) ;
#13774=CARTESIAN_POINT ( 'NONE',  ( 13.40000000000005720, 64.25000000001119815, -18.32310748452480098 ) ) ;
#13789=CARTESIAN_POINT ( 'NONE',  ( 13.40000000000005898, 64.35000000001120668, -21.02310748452479316 ) ) ;
#13796=ORIENTED_EDGE ( 'NONE', *, *, #138506, .T. ) ;
#13811=CIRCLE ( 'NONE', #109841, 0.09999999999999939493 ) ;
#13830=DIRECTION ( 'NONE',  ( 0.000000000000000000, 0.9910827722268055195, 0.1332476588733540468 ) ) ;
#13870=AXIS2_PLACEMENT_3D ( 'NONE', #130521, #117070, #90100 ) ;
#13905=AXIS2_PLACEMENT_3D ( 'NONE', #122932, #88592, #202463 ) ;
#13909=DIRECTION ( 'NONE',  ( 0.000000000000000000, 0.000000000000000000, -1.000000000000000000 ) ) ;
#13960=EDGE_CURVE ( 'NONE', #224235, #92271, #196928, .T. ) ;
#13983=EDGE_CURVE ( 'NONE', #248236, #192885, #135201, .T. ) ;
#14023=CARTESIAN_POINT ( 'NONE',  ( -21.14999999999994174, 74.94272479589878344, -3.023107484524792277 ) ) ;
#14046=ORIENTED_EDGE ( 'NONE', *, *, #174401, .F. ) ;
#14054=ORIENTED_EDGE ( 'NONE', *, *, #75636, .F. ) ;
#14055=AXIS2_PLACEMENT_3D ( 'NONE', #134334, #135623, #211329 ) ;
#14081=CARTESIAN_POINT ( 'NONE',  ( -13.39999999999994529, 67.75000000001118394, -16.98168612828748181 ) ) ;
#14126=DIRECTION ( 'NONE',  ( 0.000000000000000000, -0.9910827722268055195, -0.1332476588733540468 ) ) ;
#14135=ORIENTED_EDGE ( 'NONE', *, *, #253187, .T. ) ;
#14155=LINE ( 'NONE', #254007, #53938 ) ;
#14257=ORIENTED_EDGE ( 'NONE', *, *, #42522, .T. ) ;
#14293=CYLINDRICAL_SURFACE ( 'NONE', #69639, 0.09999999999999982514 ) ;
#14315=CYLINDRICAL_SURFACE ( 'NONE', #2954, 0.09999999999999939493 ) ;
#14340=ORIENTED_EDGE ( 'NONE', *, *, #213756, .T. ) ;
#14416=AXIS2_PLACEMENT_3D ( 'NONE', #205276, #127041, #103597 ) ;
#14472=CARTESIAN_POINT ( 'NONE',  ( -23.39999999999994529, 74.83745509109094485, -43.92310748452479885 ) ) ;
#14536=ORIENTED_EDGE ( 'NONE', *, *, #142536, .T. ) ;
#14572=ORIENTED_EDGE ( 'NONE', *, *, #71480, .F. ) ;
#14593=EDGE_LOOP ( 'NONE', ( #37242, #15404, #132835, #91312 ) ) ;
#14601=EDGE_LOOP ( 'NONE', ( #47038, #174680, #215860, #23375 ) ) ;
#14679=EDGE_CURVE ( 'NONE', #45216, #17064, #85007, .T. ) ;
#14693=DIRECTION ( 'NONE',  ( 1.000000000000000000, 0.000000000000000000, -0.000000000000000000 ) ) ;
#14715=CARTESIAN_POINT ( 'NONE',  ( 0.9000000000000547562, 64.35000000001120668, -10.02310748452479139 ) ) ;
#14764=CARTESIAN_POINT ( 'NONE',  ( -21.04999999999994387, 64.35000000001120668, -30.12310748452479103 ) ) ;
#14802=FACE_OUTER_BOUND ( 'NONE', #142238, .T. ) ;
#14806=DIRECTION ( 'NONE',  ( -1.000000000000000000, -0.000000000000000000, 0.000000000000000000 ) ) ;
#14829=VERTEX_POINT ( 'NONE', #30214 ) ;
#14843=DIRECTION ( 'NONE',  ( 0.000000000000000000, 0.000000000000000000, 1.000000000000000000 ) ) ;
#14876=LINE ( 'NONE', #249622, #248009 ) ;
#14882=DIRECTION ( 'NONE',  ( -0.000000000000000000, 0.9910827722268049644, -0.1332476588733589318 ) ) ;
#14893=EDGE_LOOP ( 'NONE', ( #61675, #142377, #175182, #100694 ) ) ;
#14962=FACE_OUTER_BOUND ( 'NONE', #146804, .T. ) ;
#15078=ORIENTED_EDGE ( 'NONE', *, *, #206989, .T. ) ;
#15110=DIRECTION ( 'NONE',  ( 0.000000000000000000, 1.000000000000000000, -0.000000000000000000 ) ) ;
#15130=CIRCLE ( 'NONE', #194209, 0.09999999999999939493 ) ;
#15171=VERTEX_POINT ( 'NONE', #65159 ) ;
#15179=LINE ( 'NONE', #94692, #34577 ) ;
#15198=AXIS2_PLACEMENT_3D ( 'NONE', #103703, #47593, #163713 ) ;
#15219=EDGE_CURVE ( 'NONE', #144016, #202492, #144115, .T. ) ;
#15222=ORIENTED_EDGE ( 'NONE', *, *, #146087, .F. ) ;
#15224=CARTESIAN_POINT ( 'NONE',  ( 6.100000000000060929, 64.35000000001120668, -25.92310748452479174 ) ) ;
#15261=VERTEX_POINT ( 'NONE', #11638 ) ;
#15297=ORIENTED_EDGE ( 'NONE', *, *, #18649, .F. ) ;
#15387=ORIENTED_EDGE ( 'NONE', *, *, #11231, .T. ) ;
#15404=ORIENTED_EDGE ( 'NONE', *, *, #36383, .T. ) ;
#15434=CARTESIAN_POINT ( 'NONE',  ( 21.05000000000005400, 65.19115966511134275, -30.12310748452479103 ) ) ;
#15464=VECTOR ( 'NONE', #82545, 1000.000000000000000 ) ;
#15498=CARTESIAN_POINT ( 'NONE',  ( -23.39999999999994529, 77.36076146337680370, -43.99645795275012006 ) ) ;
#15540=EDGE_CURVE ( 'NONE', #6487, #209133, #150809, .T. ) ;
#15549=FACE_OUTER_BOUND ( 'NONE', #231038, .T. ) ;
#15572=DIRECTION ( 'NONE',  ( -1.000000000000000000, 0.000000000000000000, -0.000000000000000000 ) ) ;
#15581=ORIENTED_EDGE ( 'NONE', *, *, #5501, .F. ) ;
#15633=CYLINDRICAL_SURFACE ( 'NONE', #29487, 2.599999999999998312 ) ;
#15639=ADVANCED_FACE ( 'NONE', ( #16463 ), #231834, .T. ) ;
#15649=DIRECTION ( 'NONE',  ( 0.000000000000000000, 0.000000000000000000, 1.000000000000000000 ) ) ;
#15695=DIRECTION ( 'NONE',  ( 1.000000000000000000, 0.000000000000000000, 0.000000000000000000 ) ) ;
#15726=DIRECTION ( 'NONE',  ( 0.000000000000000000, 0.000000000000000000, -1.000000000000000000 ) ) ;
#15731=FACE_OUTER_BOUND ( 'NONE', #128574, .T. ) ;
#15765=LINE ( 'NONE', #31475, #32410 ) ;
#15809=DIRECTION ( 'NONE',  ( 0.000000000000000000, 0.000000000000000000, -1.000000000000000000 ) ) ;
#15825=DIRECTION ( 'NONE',  ( 1.000000000000000000, -0.000000000000000000, -0.000000000000000000 ) ) ;
#15865=TOROIDAL_SURFACE ( 'NONE', #157325, 11.65000000000000036, 0.1000000000000000056 ) ;
#15890=CARTESIAN_POINT ( 'NONE',  ( -40.23850191057533010, 65.25000000001119815, -4.423107484524790856 ) ) ;
#15908=VERTEX_POINT ( 'NONE', #128383 ) ;
#15912=ORIENTED_EDGE ( 'NONE', *, *, #64587, .F. ) ;
#15945=CARTESIAN_POINT ( 'NONE',  ( -21.04999999999994387, 83.90000000001120384, -34.86056257560453986 ) ) ;
#15957=CYLINDRICAL_SURFACE ( 'NONE', #156846, 0.09999999999999939493 ) ;
#16042=FACE_OUTER_BOUND ( 'NONE', #47930, .T. ) ;
#16063=ORIENTED_EDGE ( 'NONE', *, *, #117310, .F. ) ;
#16086=ORIENTED_EDGE ( 'NONE', *, *, #242478, .F. ) ;
#16113=EDGE_LOOP ( 'NONE', ( #98849, #63173, #1952, #28126 ) ) ;
#16268=FACE_OUTER_BOUND ( 'NONE', #93488, .T. ) ;
#16389=CARTESIAN_POINT ( 'NONE',  ( 13.40000000000005898, 67.65000000001118963, -21.02310748452479316 ) ) ;
#16409=EDGE_CURVE ( 'NONE', #90507, #19078, #153113, .T. ) ;
#16410=DIRECTION ( 'NONE',  ( 0.000000000000000000, 0.1575546449569621699, -0.9875102702516493913 ) ) ;
#16419=ORIENTED_EDGE ( 'NONE', *, *, #200332, .F. ) ;
#16426=CIRCLE ( 'NONE', #116375, 11.65000000000000036 ) ;
#16463=FACE_OUTER_BOUND ( 'NONE', #53296, .T. ) ;
#16475=CARTESIAN_POINT ( 'NONE',  ( 21.05000000000005400, 66.15000000001120384, -5.923107484524795296 ) ) ;
#16528=ORIENTED_EDGE ( 'NONE', *, *, #197824, .F. ) ;
#16530=ORIENTED_EDGE ( 'NONE', *, *, #155408, .T. ) ;
#16531=DIRECTION ( 'NONE',  ( 1.000000000000000000, 0.000000000000000000, 0.000000000000000000 ) ) ;
#16560=VECTOR ( 'NONE', #235069, 1000.000000000000000 ) ;
#16574=DIRECTION ( 'NONE',  ( 0.000000000000000000, -0.7071067811865477948, -0.7071067811865473507 ) ) ;
#16645=FACE_OUTER_BOUND ( 'NONE', #105945, .T. ) ;
#16704=CARTESIAN_POINT ( 'NONE',  ( 21.15000000000005187, 74.94272479589878344, -8.023107484524793165 ) ) ;
#16794=ORIENTED_EDGE ( 'NONE', *, *, #193020, .T. ) ;
#16826=VECTOR ( 'NONE', #73349, 1000.000000000000000 ) ;
#16834=FACE_OUTER_BOUND ( 'NONE', #48777, .T. ) ;
#16843=AXIS2_PLACEMENT_3D ( 'NONE', #145443, #144149, #67203 ) ;
#16872=CARTESIAN_POINT ( 'NONE',  ( 23.50000000000005684, 77.16254490893143725, -44.02310748452479316 ) ) ;
#16873=AXIS2_PLACEMENT_3D ( 'NONE', #123439, #81698, #80414 ) ;
#16881=DIRECTION ( 'NONE',  ( 0.000000000000000000, -0.7071067811865472397, -0.7071067811865479058 ) ) ;
#16931=CARTESIAN_POINT ( 'NONE',  ( 23.50000000000005684, 79.78873604695631627, -7.297728304630792806 ) ) ;
#16937=AXIS2_PLACEMENT_3D ( 'NONE', #184020, #142322, #22409 ) ;
#16942=LINE ( 'NONE', #1192, #182692 ) ;
#16952=AXIS2_PLACEMENT_3D ( 'NONE', #11488, #230533, #7626 ) ;
#17048=ADVANCED_FACE ( 'NONE', ( #144955 ), #27633, .T. ) ;
#17064=VERTEX_POINT ( 'NONE', #142400 ) ;
#17074=FACE_OUTER_BOUND ( 'NONE', #125058, .T. ) ;
#17084=ORIENTED_EDGE ( 'NONE', *, *, #248568, .F. ) ;
#17117=VECTOR ( 'NONE', #115455, 1000.000000000000114 ) ;
#17164=LINE ( 'NONE', #15890, #244964 ) ;
#17175=FACE_OUTER_BOUND ( 'NONE', #219417, .T. ) ;
#17202=AXIS2_PLACEMENT_3D ( 'NONE', #156318, #255324, #139256 ) ;
#17306=ADVANCED_FACE ( 'NONE', ( #30345, #105986 ), #186852, .T. ) ;
#17333=DIRECTION ( 'NONE',  ( 0.000000000000000000, 0.000000000000000000, 1.000000000000000000 ) ) ;
#17336=CARTESIAN_POINT ( 'NONE',  ( 20.95000000000005613, 67.82483145523551116, -25.59432346794077162 ) ) ;
#17341=DIRECTION ( 'NONE',  ( -0.000000000000000000, 0.9910827722268049644, 0.1332476588733589318 ) ) ;
#17344=DIRECTION ( 'NONE',  ( 0.000000000000000000, 1.000000000000000000, 0.000000000000000000 ) ) ;
#17355=EDGE_CURVE ( 'NONE', #103163, #211446, #27797, .T. ) ;
#17368=EDGE_CURVE ( 'NONE', #179805, #116279, #148787, .T. ) ;
#17380=DIRECTION ( 'NONE',  ( 1.000000000000000000, -0.000000000000000000, -0.000000000000000000 ) ) ;
#17389=EDGE_CURVE ( 'NONE', #15908, #137320, #95437, .T. ) ;
#17466=EDGE_CURVE ( 'NONE', #243985, #248236, #228468, .T. ) ;
#17470=CARTESIAN_POINT ( 'NONE',  ( -23.39999999999994529, 83.80000000001119531, -34.86056257560453986 ) ) ;
#17509=CARTESIAN_POINT ( 'NONE',  ( -21.04999999999994387, 76.00000000001119815, -36.02310748452479316 ) ) ;
#17543=AXIS2_PLACEMENT_3D ( 'NONE', #4914, #84432, #127463 ) ;
#17614=CARTESIAN_POINT ( 'NONE',  ( -23.49999999999994316, 87.60324567546805952, -34.17184040628037422 ) ) ;
#17702=DIRECTION ( 'NONE',  ( 1.000000000000000000, 0.000000000000000000, 0.000000000000000000 ) ) ;
#17728=DIRECTION ( 'NONE',  ( 1.000000000000000000, 0.000000000000000000, 0.000000000000000000 ) ) ;
#17729=EDGE_LOOP ( 'NONE', ( #60761, #191038, #130573, #103437 ) ) ;
#17759=AXIS2_PLACEMENT_3D ( 'NONE', #120350, #21243, #218103 ) ;
#17787=DIRECTION ( 'NONE',  ( 0.000000000000000000, 0.000000000000000000, -1.000000000000000000 ) ) ;
#17795=CARTESIAN_POINT ( 'NONE',  ( -21.04999999999994387, 67.75000000001118394, -51.02310748452479316 ) ) ;
#17812=DIRECTION ( 'NONE',  ( 0.000000000000000000, 1.000000000000000000, 0.000000000000000000 ) ) ;
#17858=ADVANCED_FACE ( 'NONE', ( #59830 ), #90683, .T. ) ;
#17859=CARTESIAN_POINT ( 'NONE',  ( -23.49999999999994316, 74.94272479589878344, -8.023107484524793165 ) ) ;
#17871=EDGE_CURVE ( 'NONE', #221278, #135540, #122405, .T. ) ;
#17899=VECTOR ( 'NONE', #107798, 1000.000000000000000 ) ;
#17919=EDGE_LOOP ( 'NONE', ( #151768, #99821, #143837, #92593 ) ) ;
#17923=ORIENTED_EDGE ( 'NONE', *, *, #227971, .T. ) ;
#17931=CIRCLE ( 'NONE', #34717, 4.150000000000001243 ) ;
#18034=CIRCLE ( 'NONE', #172213, 2.599999999999998312 ) ;
#18052=CYLINDRICAL_SURFACE ( 'NONE', #123069, 0.1000000000000002554 ) ;
#18072=ADVANCED_FACE ( 'NONE', ( #127535 ), #94783, .T. ) ;
#18076=EDGE_CURVE ( 'NONE', #177623, #116279, #107974, .T. ) ;
#18100=VERTEX_POINT ( 'NONE', #36151 ) ;
#18131=ORIENTED_EDGE ( 'NONE', *, *, #73558, .T. ) ;
#18162=DIRECTION ( 'NONE',  ( 0.000000000000000000, 0.000000000000000000, 1.000000000000000000 ) ) ;
#18170=DIRECTION ( 'NONE',  ( 0.000000000000000000, -0.7071067811865477948, 0.7071067811865473507 ) ) ;
#18179=DIRECTION ( 'NONE',  ( 0.000000000000000000, 0.000000000000000000, 1.000000000000000000 ) ) ;
#18223=VECTOR ( 'NONE', #52357, 999.9999999999998863 ) ;
#18243=ORIENTED_EDGE ( 'NONE', *, *, #174401, .T. ) ;
#18304=LINE ( 'NONE', #241222, #253231 ) ;
#18351=DIRECTION ( 'NONE',  ( -1.000000000000000000, 0.000000000000000000, 0.000000000000000000 ) ) ;
#18358=CARTESIAN_POINT ( 'NONE',  ( 23.50000000000005684, 76.00000000001119815, -36.02310748452479316 ) ) ;
#18362=CONICAL_SURFACE ( 'NONE', #168242, 4.000000000000000000, 0.7853981633974489451 ) ;
#18365=AXIS2_PLACEMENT_3D ( 'NONE', #113308, #57159, #74224 ) ;
#18448=DIRECTION ( 'NONE',  ( 0.000000000000000000, 0.000000000000000000, 1.000000000000000000 ) ) ;
#18464=DIRECTION ( 'NONE',  ( -1.000000000000000000, 0.000000000000000000, 0.000000000000000000 ) ) ;
#18526=EDGE_LOOP ( 'NONE', ( #317, #193214, #126025 ) ) ;
#18533=DIRECTION ( 'NONE',  ( -0.000000000000000000, 1.000000000000000000, 0.000000000000000000 ) ) ;
#18578=DIRECTION ( 'NONE',  ( 1.661467591126378393E-14, -0.9910827722268042983, -0.1332476588733650935 ) ) ;
#18622=DIRECTION ( 'NONE',  ( -1.000000000000000000, 0.000000000000000000, 0.000000000000000000 ) ) ;
#18649=EDGE_CURVE ( 'NONE', #85681, #169497, #44813, .T. ) ;
#18655=ORIENTED_EDGE ( 'NONE', *, *, #253164, .F. ) ;
#18690=EDGE_LOOP ( 'NONE', ( #210591, #80799, #13796, #153418 ) ) ;
#18701=ADVANCED_FACE ( 'NONE', ( #91339 ), #249297, .T. ) ;
#18753=DIRECTION ( 'NONE',  ( 0.000000000000000000, -0.000000000000000000, 1.000000000000000000 ) ) ;
#18837=ORIENTED_EDGE ( 'NONE', *, *, #146318, .T. ) ;
#18983=EDGE_LOOP ( 'NONE', ( #71893, #80288, #157638, #182612 ) ) ;
#19055=CARTESIAN_POINT ( 'NONE',  ( 21.15000000000005187, 74.16448838626247664, -47.52760213295649550 ) ) ;
#19078=VERTEX_POINT ( 'NONE', #56988 ) ;
#19190=DIRECTION ( 'NONE',  ( -1.000000000000000000, 0.000000000000000000, 0.000000000000000000 ) ) ;
#19213=SPHERICAL_SURFACE ( 'NONE', #199670, 0.1000000000000000056 ) ;
#19235=DIRECTION ( 'NONE',  ( -1.000000000000000000, 0.000000000000000000, 0.000000000000000000 ) ) ;
#19237=LINE ( 'NONE', #180889, #148011 ) ;
#19238=DIRECTION ( 'NONE',  ( 0.000000000000000000, 1.000000000000000000, 0.000000000000000000 ) ) ;
#19244=EDGE_CURVE ( 'NONE', #39283, #104351, #242066, .T. ) ;
#19257=ORIENTED_EDGE ( 'NONE', *, *, #61404, .F. ) ;
#19307=ADVANCED_FACE ( 'NONE', ( #236943 ), #58284, .T. ) ;
#19328=EDGE_CURVE ( 'NONE', #63115, #100189, #62164, .T. ) ;
#19367=CARTESIAN_POINT ( 'NONE',  ( -5.999999999999938716, 64.65000000001120384, -26.02310748452479316 ) ) ;
#19424=CARTESIAN_POINT ( 'NONE',  ( 21.05000000000005400, 67.75000000001118394, -51.02310748452479316 ) ) ;
#19438=DIRECTION ( 'NONE',  ( 0.000000000000000000, -0.7071067811865479058, 0.7071067811865472397 ) ) ;
#19470=CARTESIAN_POINT ( 'NONE',  ( -21.14999999999994174, 64.25000000001119815, -30.12310748452479103 ) ) ;
#19480=ORIENTED_EDGE ( 'NONE', *, *, #214676, .T. ) ;
#19487=DIRECTION ( 'NONE',  ( 0.000000000000000000, 1.000000000000000000, 0.000000000000000000 ) ) ;
#19504=EDGE_LOOP ( 'NONE', ( #5356, #154089, #3817, #31451 ) ) ;
#19646=DIRECTION ( 'NONE',  ( 0.000000000000000000, 0.000000000000000000, -1.000000000000000000 ) ) ;
#19654=ADVANCED_FACE ( 'NONE', ( #157116 ), #138772, .T. ) ;
#19676=DIRECTION ( 'NONE',  ( 0.000000000000000000, -1.000000000000000000, 0.000000000000000000 ) ) ;
#19740=ORIENTED_EDGE ( 'NONE', *, *, #217306, .F. ) ;
#19822=AXIS2_PLACEMENT_3D ( 'NONE', #3757, #183691, #84527 ) ;
#19825=EDGE_CURVE ( 'NONE', #186900, #60596, #4427, .T. ) ;
#19854=ORIENTED_EDGE ( 'NONE', *, *, #226448, .T. ) ;
#19869=ADVANCED_FACE ( 'NONE', ( #94244 ), #242097, .T. ) ;
#19891=ORIENTED_EDGE ( 'NONE', *, *, #214755, .T. ) ;
#19913=ORIENTED_EDGE ( 'NONE', *, *, #249561, .T. ) ;
#19937=VECTOR ( 'NONE', #186848, 1000.000000000000000 ) ;
#19951=AXIS2_PLACEMENT_3D ( 'NONE', #192834, #71613, #136683 ) ;
#19958=CARTESIAN_POINT ( 'NONE',  ( 5.900000000000059863, 64.75000000001119815, -26.02310748452479316 ) ) ;
#19985=FACE_OUTER_BOUND ( 'NONE', #153828, .T. ) ;
#20003=ORIENTED_EDGE ( 'NONE', *, *, #96953, .T. ) ;
#20012=AXIS2_PLACEMENT_3D ( 'NONE', #140289, #22963, #144140 ) ;
#20063=CARTESIAN_POINT ( 'NONE',  ( -40.23850191057533010, 66.15000000001120384, -5.923107484524795296 ) ) ;
#20084=CARTESIAN_POINT ( 'NONE',  ( 20.95000000000005258, 65.25000000001119815, -3.123107484524795474 ) ) ;
#20182=AXIS2_PLACEMENT_3D ( 'NONE', #128209, #91646, #12135 ) ;
#20197=FACE_OUTER_BOUND ( 'NONE', #49165, .T. ) ;
#20203=FACE_OUTER_BOUND ( 'NONE', #121989, .T. ) ;
#20297=ORIENTED_EDGE ( 'NONE', *, *, #153269, .F. ) ;
#20346=CARTESIAN_POINT ( 'NONE',  ( -21.04999999999994387, 67.75000000001118394, -43.82310748452479743 ) ) ;
#20353=CARTESIAN_POINT ( 'NONE',  ( 13.40000000000005898, 64.25000000001119815, -23.72310748452479601 ) ) ;
#20383=ORIENTED_EDGE ( 'NONE', *, *, #13159, .F. ) ;
#20395=ORIENTED_EDGE ( 'NONE', *, *, #94412, .T. ) ;
#20397=LINE ( 'NONE', #22977, #51836 ) ;
#20423=ORIENTED_EDGE ( 'NONE', *, *, #157087, .T. ) ;
#20456=DIRECTION ( 'NONE',  ( 1.000000000000000000, -0.000000000000000000, 0.000000000000000000 ) ) ;
#20477=SPHERICAL_SURFACE ( 'NONE', #33287, 0.1000000000000000056 ) ;
#20495=FACE_OUTER_BOUND ( 'NONE', #60586, .T. ) ;
#20544=VERTEX_POINT ( 'NONE', #141197 ) ;
#20678=DIRECTION ( 'NONE',  ( -0.000000000000000000, 1.000000000000000000, -0.000000000000000000 ) ) ;
#20731=CARTESIAN_POINT ( 'NONE',  ( -21.14999999999994174, 77.36076146337680370, -43.99645795275012006 ) ) ;
#20749=EDGE_CURVE ( 'NONE', #3592, #189995, #111710, .T. ) ;
#20764=ORIENTED_EDGE ( 'NONE', *, *, #52047, .F. ) ;
#20775=EDGE_CURVE ( 'NONE', #161116, #137320, #195125, .T. ) ;
#20815=EDGE_LOOP ( 'NONE', ( #234589, #87668, #63025, #43144 ) ) ;
#20826=SHAPE_DEFINITION_REPRESENTATION ( #193165, #133560 ) ;
#20831=DIRECTION ( 'NONE',  ( 0.000000000000000000, 0.000000000000000000, -1.000000000000000000 ) ) ;
#20832=CONICAL_SURFACE ( 'NONE', #166577, 4.000000000000000000, 0.7853981633974489451 ) ;
#20843=DIRECTION ( 'NONE',  ( -0.000000000000000000, 0.000000000000000000, -1.000000000000000000 ) ) ;
#20937=VECTOR ( 'NONE', #176294, 1000.000000000000000 ) ;
#20951=CARTESIAN_POINT ( 'NONE',  ( 23.40000000000005187, 76.00000000001119815, -40.17310748452479174 ) ) ;
#20978=AXIS2_PLACEMENT_3D ( 'NONE', #39979, #236855, #180749 ) ;
#21018=VERTEX_POINT ( 'NONE', #33497 ) ;
#21048=DIRECTION ( 'NONE',  ( 1.000000000000000000, 0.000000000000000000, 0.000000000000000000 ) ) ;
#21166=ORIENTED_EDGE ( 'NONE', *, *, #205775, .F. ) ;
#21187=VERTEX_POINT ( 'NONE', #38590 ) ;
#21231=CIRCLE ( 'NONE', #83692, 0.09999999999999939493 ) ;
#21243=DIRECTION ( 'NONE',  ( -0.000000000000000000, 1.000000000000000000, -0.000000000000000000 ) ) ;
#21285=CIRCLE ( 'NONE', #162937, 0.1000000000000028644 ) ;
#21288=ORIENTED_EDGE ( 'NONE', *, *, #250244, .F. ) ;
#21298=ORIENTED_EDGE ( 'NONE', *, *, #188316, .T. ) ;
#21305=EDGE_LOOP ( 'NONE', ( #221693, #97604, #248495, #83671 ) ) ;
#21313=ORIENTED_EDGE ( 'NONE', *, *, #5534, .T. ) ;
#21325=ORIENTED_EDGE ( 'NONE', *, *, #125578, .T. ) ;
#21341=VECTOR ( 'NONE', #165771, 1000.000000000000000 ) ;
#21361=CYLINDRICAL_SURFACE ( 'NONE', #257189, 0.1000000000000002554 ) ;
#21419=CIRCLE ( 'NONE', #200461, 0.09999999999999635569 ) ;
#21451=ORIENTED_EDGE ( 'NONE', *, *, #72982, .T. ) ;
#21452=AXIS2_PLACEMENT_3D ( 'NONE', #5874, #46289, #4593 ) ;
#21481=AXIS2_PLACEMENT_3D ( 'NONE', #52757, #12388, #132304 ) ;
#21517=VECTOR ( 'NONE', #221217, 1000.000000000000000 ) ;
#21531=ORIENTED_EDGE ( 'NONE', *, *, #66157, .F. ) ;
#21627=ORIENTED_EDGE ( 'NONE', *, *, #196634, .T. ) ;
#21649=ORIENTED_EDGE ( 'NONE', *, *, #84168, .F. ) ;
#21755=CIRCLE ( 'NONE', #55037, 0.1999999999999987899 ) ;
#21815=AXIS2_PLACEMENT_3D ( 'NONE', #112857, #209385, #248511 ) ;
#21878=VERTEX_POINT ( 'NONE', #39290 ) ;
#21887=EDGE_CURVE ( 'NONE', #179805, #77787, #140942, .T. ) ;
#21965=CARTESIAN_POINT ( 'NONE',  ( 6.000000000000060396, 64.65000000001120384, -25.92310748452479174 ) ) ;
#21985=EDGE_CURVE ( 'NONE', #135971, #37851, #207579, .T. ) ;
#22102=ORIENTED_EDGE ( 'NONE', *, *, #239506, .F. ) ;
#22153=FACE_OUTER_BOUND ( 'NONE', #67532, .T. ) ;
#22195=ORIENTED_EDGE ( 'NONE', *, *, #186650, .T. ) ;
#22228=CARTESIAN_POINT ( 'NONE',  ( -23.49999999999994316, 77.16254490893143725, -44.02310748452479316 ) ) ;
#22275=DIRECTION ( 'NONE',  ( 0.000000000000000000, 0.1575546449569757979, 0.9875102702516471709 ) ) ;
#22285=DIRECTION ( 'NONE',  ( -0.000000000000000000, 1.000000000000000000, 0.000000000000000000 ) ) ;
#22296=ADVANCED_FACE ( 'NONE', ( #167097 ), #83628, .T. ) ;
#22308=CYLINDRICAL_SURFACE ( 'NONE', #135538, 0.09999999999999530098 ) ;
#22339=DIRECTION ( 'NONE',  ( -1.000000000000000000, 0.000000000000000000, 0.000000000000000000 ) ) ;
#22385=TOROIDAL_SURFACE ( 'NONE', #55631, 4.900000000000000355, 0.1000000000000000056 ) ;
#22403=DIRECTION ( 'NONE',  ( -0.000000000000000000, 0.000000000000000000, -1.000000000000000000 ) ) ;
#22409=DIRECTION ( 'NONE',  ( 0.000000000000000000, 0.000000000000000000, 1.000000000000000000 ) ) ;
#22425=EDGE_LOOP ( 'NONE', ( #100536, #82314, #126085, #42443 ) ) ;
#22429=VECTOR ( 'NONE', #24406, 1000.000000000000000 ) ;
#22441=DIRECTION ( 'NONE',  ( 1.000000000000000000, -0.000000000000000000, 0.000000000000000000 ) ) ;
#22448=CARTESIAN_POINT ( 'NONE',  ( -23.49999999999994316, 64.35000000001120668, -3.123107484524795474 ) ) ;
#22457=VERTEX_POINT ( 'NONE', #190501 ) ;
#22602=ORIENTED_EDGE ( 'NONE', *, *, #36412, .F. ) ;
#22615=ORIENTED_EDGE ( 'NONE', *, *, #224280, .F. ) ;
#22748=ORIENTED_EDGE ( 'NONE', *, *, #252772, .T. ) ;
#22750=CARTESIAN_POINT ( 'NONE',  ( 11.60000000000006004, 67.75000000001118394, -21.02310748452479316 ) ) ;
#22870=FACE_OUTER_BOUND ( 'NONE', #236129, .T. ) ;
#22926=AXIS2_PLACEMENT_3D ( 'NONE', #96248, #175822, #114549 ) ;
#22963=DIRECTION ( 'NONE',  ( 1.000000000000000000, 0.000000000000000000, 0.000000000000000000 ) ) ;
#22977=CARTESIAN_POINT ( 'NONE',  ( 11.60000000000006004, 67.75000000001118394, -18.42310748452479530 ) ) ;
#23019=DIRECTION ( 'NONE',  ( -1.000000000000000000, 0.000000000000000000, 0.000000000000000000 ) ) ;
#23050=DIRECTION ( 'NONE',  ( 1.000000000000000000, 0.000000000000000000, -0.000000000000000000 ) ) ;
#23060=FACE_OUTER_BOUND ( 'NONE', #23623, .T. ) ;
#23071=CARTESIAN_POINT ( 'NONE',  ( 20.95000000000005969, 65.27857539272349641, -29.97167177764265844 ) ) ;
#23074=CARTESIAN_POINT ( 'NONE',  ( -0.8999999999999437339, 66.35000000001119247, -7.423107484524793520 ) ) ;
#23080=VECTOR ( 'NONE', #51913, 1000.000000000000000 ) ;
#23100=DIRECTION ( 'NONE',  ( 0.000000000000000000, 1.000000000000000000, -0.000000000000000000 ) ) ;
#23129=CIRCLE ( 'NONE', #85603, 0.09999999999999939493 ) ;
#23140=DIRECTION ( 'NONE',  ( 0.000000000000000000, 0.000000000000000000, -1.000000000000000000 ) ) ;
#23158=CARTESIAN_POINT ( 'NONE',  ( 21.05000000000005400, 89.48413628383013929, -38.12477508515532065 ) ) ;
#23181=VERTEX_POINT ( 'NONE', #107745 ) ;
#23192=ORIENTED_EDGE ( 'NONE', *, *, #126282, .T. ) ;
#23235=AXIS2_PLACEMENT_3D ( 'NONE', #189486, #51218, #10848 ) ;
#23264=CARTESIAN_POINT ( 'NONE',  ( -21.04999999999994387, 74.83745509109094485, -43.82310748452479743 ) ) ;
#23265=AXIS2_PLACEMENT_3D ( 'NONE', #911, #178333, #120930 ) ;
#23302=FACE_OUTER_BOUND ( 'NONE', #81284, .T. ) ;
#23353=VERTEX_POINT ( 'NONE', #115445 ) ;
#23375=ORIENTED_EDGE ( 'NONE', *, *, #122302, .T. ) ;
#23384=CIRCLE ( 'NONE', #148239, 0.09999999999999530098 ) ;
#23405=CARTESIAN_POINT ( 'NONE',  ( -21.14999999999994174, 77.85126707825561709, -47.62635315998165453 ) ) ;
#23427=AXIS2_PLACEMENT_3D ( 'NONE', #103781, #120841, #165068 ) ;
#23439=DIRECTION ( 'NONE',  ( 0.000000000000000000, 1.000000000000000000, 0.000000000000000000 ) ) ;
#23531=FACE_OUTER_BOUND ( 'NONE', #188053, .T. ) ;
#23583=ORIENTED_EDGE ( 'NONE', *, *, #142070, .T. ) ;
#23590=ORIENTED_EDGE ( 'NONE', *, *, #40458, .T. ) ;
#23600=ORIENTED_EDGE ( 'NONE', *, *, #255632, .F. ) ;
#23604=CARTESIAN_POINT ( 'NONE',  ( -23.49999999999994316, 87.51781941433023349, -37.75951082105083145 ) ) ;
#23611=VERTEX_POINT ( 'NONE', #14472 ) ;
#23623=EDGE_LOOP ( 'NONE', ( #183859, #88486, #168353, #61897 ) ) ;
#23626=VERTEX_POINT ( 'NONE', #176112 ) ;
#23643=ORIENTED_EDGE ( 'NONE', *, *, #106886, .F. ) ;
#23717=CIRCLE ( 'NONE', #240175, 0.1000000000000028644 ) ;
#23722=EDGE_CURVE ( 'NONE', #204034, #146220, #150228, .T. ) ;
#23732=DIRECTION ( 'NONE',  ( -1.284434275755705789E-16, 0.7071067811865472397, -0.7071067811865479058 ) ) ;
#23747=CARTESIAN_POINT ( 'NONE',  ( 21.05000000000005400, 76.00000000001119815, -36.02310748452479316 ) ) ;
#23762=EDGE_LOOP ( 'NONE', ( #37477, #40612, #63650 ) ) ;
#23786=CARTESIAN_POINT ( 'NONE',  ( 21.05000000000005400, 67.85000000001119247, -3.023107484524792277 ) ) ;
#23803=DIRECTION ( 'NONE',  ( -0.000000000000000000, 1.000000000000000000, -0.000000000000000000 ) ) ;
#23866=ORIENTED_EDGE ( 'NONE', *, *, #30190, .F. ) ;
#23917=CYLINDRICAL_SURFACE ( 'NONE', #26188, 0.09999999999999939493 ) ;
#23924=DIRECTION ( 'NONE',  ( 0.000000000000000000, 0.000000000000000000, -1.000000000000000000 ) ) ;
#23932=ORIENTED_EDGE ( 'NONE', *, *, #106728, .T. ) ;
#23976=ORIENTED_EDGE ( 'NONE', *, *, #81123, .F. ) ;
#24002=CARTESIAN_POINT ( 'NONE',  ( -23.49999999999994316, 87.60324567546805952, -34.17184040628037422 ) ) ;
#24030=DIRECTION ( 'NONE',  ( 1.000000000000000000, 0.000000000000000000, 0.000000000000000000 ) ) ;
#24114=CYLINDRICAL_SURFACE ( 'NONE', #14416, 4.049999999999998046 ) ;
#24123=CARTESIAN_POINT ( 'NONE',  ( 21.05000000000005400, 65.15000000001120384, -3.123107484524795474 ) ) ;
#24132=CARTESIAN_POINT ( 'NONE',  ( 23.50000000000005684, 82.84256550613280012, -26.34830530078816935 ) ) ;
#24135=ORIENTED_EDGE ( 'NONE', *, *, #3089, .T. ) ;
#24145=CARTESIAN_POINT ( 'NONE',  ( 21.15000000000005187, 64.25000000001119815, -6.023107484524794941 ) ) ;
#24177=AXIS2_PLACEMENT_3D ( 'NONE', #156436, #58558, #39035 ) ;
#24188=DIRECTION ( 'NONE',  ( -1.000000000000000000, -0.000000000000000000, -0.000000000000000000 ) ) ;
#24207=ORIENTED_EDGE ( 'NONE', *, *, #161533, .F. ) ;
#24211=EDGE_CURVE ( 'NONE', #58156, #111921, #129559, .T. ) ;
#24218=DIRECTION ( 'NONE',  ( 1.000000000000000000, 0.000000000000000000, 0.000000000000000000 ) ) ;
#24248=DIRECTION ( 'NONE',  ( 0.000000000000000000, 0.000000000000000000, -1.000000000000000000 ) ) ;
#24311=DIRECTION ( 'NONE',  ( 0.000000000000000000, 0.000000000000000000, -1.000000000000000000 ) ) ;
#24312=ORIENTED_EDGE ( 'NONE', *, *, #118295, .F. ) ;
#24374=DIRECTION ( 'NONE',  ( -1.000000000000000000, 0.000000000000000000, 0.000000000000000000 ) ) ;
#24406=DIRECTION ( 'NONE',  ( -0.000000000000000000, 0.000000000000000000, -1.000000000000000000 ) ) ;
#24407=ORIENTED_EDGE ( 'NONE', *, *, #103123, .T. ) ;
#24489=DIRECTION ( 'NONE',  ( -0.000000000000000000, -0.1332476588733589318, -0.9910827722268049644 ) ) ;
#24505=EDGE_CURVE ( 'NONE', #33031, #213499, #21419, .T. ) ;
#24523=ORIENTED_EDGE ( 'NONE', *, *, #9637, .F. ) ;
#24543=ORIENTED_EDGE ( 'NONE', *, *, #55293, .F. ) ;
#24547=VERTEX_POINT ( 'NONE', #115856 ) ;
#24550=FACE_OUTER_BOUND ( 'NONE', #217626, .T. ) ;
#24570=ORIENTED_EDGE ( 'NONE', *, *, #33437, .F. ) ;
#24675=DIRECTION ( 'NONE',  ( -1.000000000000000000, 0.000000000000000000, 0.000000000000000000 ) ) ;
#24752=DIRECTION ( 'NONE',  ( 1.000000000000000000, 0.000000000000000000, 0.000000000000000000 ) ) ;
#24777=VECTOR ( 'NONE', #26316, 1000.000000000000000 ) ;
#24780=LINE ( 'NONE', #246366, #117588 ) ;
#24805=DIRECTION ( 'NONE',  ( 0.000000000000000000, -0.9889818879709272315, -0.1480365673253073999 ) ) ;
#24833=EDGE_LOOP ( 'NONE', ( #6944, #251897, #2346, #234155 ) ) ;
#24841=EDGE_CURVE ( 'NONE', #250992, #129355, #30526, .T. ) ;
#24842=ORIENTED_EDGE ( 'NONE', *, *, #161503, .T. ) ;
#24890=VERTEX_POINT ( 'NONE', #225192 ) ;
#24911=ORIENTED_EDGE ( 'NONE', *, *, #12659, .T. ) ;
#24929=CIRCLE ( 'NONE', #203780, 0.1000000000000028644 ) ;
#24991=EDGE_CURVE ( 'NONE', #216036, #44045, #55411, .T. ) ;
#25012=EDGE_CURVE ( 'NONE', #153832, #15171, #52987, .T. ) ;
#25030=LINE ( 'NONE', #122839, #226011 ) ;
#25049=FACE_OUTER_BOUND ( 'NONE', #170476, .T. ) ;
#25119=DIRECTION ( 'NONE',  ( 0.000000000000000000, 0.000000000000000000, -1.000000000000000000 ) ) ;
#25266=DIRECTION ( 'NONE',  ( 0.000000000000000000, -1.000000000000000000, 0.000000000000000000 ) ) ;
#25299=CARTESIAN_POINT ( 'NONE',  ( 21.15000000000005542, 74.16448838626246243, -47.52760213295649550 ) ) ;
#25303=AXIS2_PLACEMENT_3D ( 'NONE', #139157, #58338, #178342 ) ;
#25310=CIRCLE ( 'NONE', #129534, 0.1000000000000028644 ) ;
#25318=AXIS2_PLACEMENT_3D ( 'NONE', #124070, #104462, #26253 ) ;
#25411=DIRECTION ( 'NONE',  ( 0.000000000000000000, 0.000000000000000000, 1.000000000000000000 ) ) ;
#25457=EDGE_CURVE ( 'NONE', #14829, #153040, #66099, .T. ) ;
#25459=AXIS2_PLACEMENT_3D ( 'NONE', #137951, #217485, #42716 ) ;
#25467=FACE_OUTER_BOUND ( 'NONE', #116091, .T. ) ;
#25471=DIRECTION ( 'NONE',  ( 1.000000000000000000, 0.000000000000000000, 0.000000000000000000 ) ) ;
#25495=CARTESIAN_POINT ( 'NONE',  ( -21.14999999999994174, 77.75000000001119815, -47.64205752314703801 ) ) ;
#25532=ORIENTED_EDGE ( 'NONE', *, *, #200332, .T. ) ;
#25552=ORIENTED_EDGE ( 'NONE', *, *, #128540, .F. ) ;
#25598=ADVANCED_FACE ( 'NONE', ( #131202 ), #133772, .F. ) ;
#25627=CARTESIAN_POINT ( 'NONE',  ( -23.49999999999994316, 87.75000000001119815, -51.02310748452479316 ) ) ;
#25630=CARTESIAN_POINT ( 'NONE',  ( -23.49999999999994316, 74.16448838626247664, -47.52760213295649550 ) ) ;
#25780=CARTESIAN_POINT ( 'NONE',  ( -21.04999999999994387, 64.35000000001120668, -3.123107484524795474 ) ) ;
#25793=CARTESIAN_POINT ( 'NONE',  ( -21.14999999999994174, 74.83745509109094485, -43.82310748452479743 ) ) ;
#25812=DIRECTION ( 'NONE',  ( 1.000000000000000000, 0.000000000000000000, 0.000000000000000000 ) ) ;
#25826=ORIENTED_EDGE ( 'NONE', *, *, #138172, .T. ) ;
#25835=CARTESIAN_POINT ( 'NONE',  ( -11.59999999999994458, 67.75000000001118394, -21.02310748452479316 ) ) ;
#25838=ORIENTED_EDGE ( 'NONE', *, *, #68350, .T. ) ;
#25851=CIRCLE ( 'NONE', #129872, 0.1999999999999987899 ) ;
#25901=ORIENTED_EDGE ( 'NONE', *, *, #144006, .F. ) ;
#25928=ORIENTED_EDGE ( 'NONE', *, *, #31723, .T. ) ;
#25935=VECTOR ( 'NONE', #75727, 1000.000000000000000 ) ;
#25967=CARTESIAN_POINT ( 'NONE',  ( -11.59999999999994458, 64.35000000001120668, -18.32310748452479388 ) ) ;
#26045=DIRECTION ( 'NONE',  ( 0.000000000000000000, -0.000000000000000000, -1.000000000000000000 ) ) ;
#26051=VERTEX_POINT ( 'NONE', #224441 ) ;
#26124=ORIENTED_EDGE ( 'NONE', *, *, #153269, .T. ) ;
#26188=AXIS2_PLACEMENT_3D ( 'NONE', #39635, #179141, #198668 ) ;
#26247=VERTEX_POINT ( 'NONE', #199126 ) ;
#26253=DIRECTION ( 'NONE',  ( 0.000000000000000000, 0.1332476588733589318, -0.9910827722268049644 ) ) ;
#26266=ORIENTED_EDGE ( 'NONE', *, *, #202074, .F. ) ;
#26285=CARTESIAN_POINT ( 'NONE',  ( 21.15000000000005187, 77.83551161375991967, -47.52760213295649550 ) ) ;
#26316=DIRECTION ( 'NONE',  ( 0.000000000000000000, -1.000000000000000000, 0.000000000000000000 ) ) ;
#26344=ORIENTED_EDGE ( 'NONE', *, *, #224199, .F. ) ;
#26363=AXIS2_PLACEMENT_3D ( 'NONE', #94406, #35753, #90549 ) ;
#26400=CIRCLE ( 'NONE', #88906, 0.1000000000000002554 ) ;
#26416=VERTEX_POINT ( 'NONE', #201686 ) ;
#26452=DIRECTION ( 'NONE',  ( 0.000000000000000000, 0.9889818879709272315, 0.1480365673253073999 ) ) ;
#26548=DIRECTION ( 'NONE',  ( -1.000000000000000000, 0.000000000000000000, -0.000000000000000000 ) ) ;
#26588=DIRECTION ( 'NONE',  ( 0.000000000000000000, 1.000000000000000000, 0.000000000000000000 ) ) ;
#26603=DIRECTION ( 'NONE',  ( -1.000000000000000000, 0.000000000000000000, -0.000000000000000000 ) ) ;
#26610=EDGE_CURVE ( 'NONE', #110468, #43374, #257443, .T. ) ;
#26622=VECTOR ( 'NONE', #26790, 1000.000000000000114 ) ;
#26702=AXIS2_PLACEMENT_3D ( 'NONE', #89209, #70973, #147922 ) ;
#26713=TOROIDAL_SURFACE ( 'NONE', #35107, 0.2000000000000000111, 0.1000000000000000056 ) ;
#26714=ORIENTED_EDGE ( 'NONE', *, *, #40228, .T. ) ;
#26757=ORIENTED_EDGE ( 'NONE', *, *, #236881, .T. ) ;
#26761=AXIS2_PLACEMENT_3D ( 'NONE', #36043, #33507, #94709 ) ;
#26790=DIRECTION ( 'NONE',  ( -0.000000000000000000, -0.1332476588733589318, 0.9910827722268049644 ) ) ;
#26819=CARTESIAN_POINT ( 'NONE',  ( -20.94999999999994245, 67.65000000001118963, -3.023107484524792277 ) ) ;
#26916=EDGE_CURVE ( 'NONE', #40901, #11972, #139154, .T. ) ;
#26990=EDGE_CURVE ( 'NONE', #99338, #117682, #178995, .T. ) ;
#27019=DIRECTION ( 'NONE',  ( -0.000000000000000000, 0.9910827722268049644, -0.1332476588733589318 ) ) ;
#27034=MECHANICAL_DESIGN_GEOMETRIC_PRESENTATION_REPRESENTATION('',(#43754),#131232);
#27044=DIRECTION ( 'NONE',  ( -1.000000000000000000, 0.000000000000000000, 0.000000000000000000 ) ) ;
#27060=DIRECTION ( 'NONE',  ( -0.000000000000000000, -0.000000000000000000, 1.000000000000000000 ) ) ;
#27061=AXIS2_PLACEMENT_3D ( 'NONE', #157512, #160063, #60922 ) ;
#27066=DIRECTION ( 'NONE',  ( 0.000000000000000000, 0.000000000000000000, 1.000000000000000000 ) ) ;
#27079=ORIENTED_EDGE ( 'NONE', *, *, #98305, .F. ) ;
#27111=DIRECTION ( 'NONE',  ( 0.000000000000000000, 0.000000000000000000, 1.000000000000000000 ) ) ;
#27125=ORIENTED_EDGE ( 'NONE', *, *, #64526, .F. ) ;
#27139=ORIENTED_EDGE ( 'NONE', *, *, #105775, .T. ) ;
#27144=VECTOR ( 'NONE', #37852, 1000.000000000000114 ) ;
#27155=DIRECTION ( 'NONE',  ( 0.000000000000000000, 0.000000000000000000, -1.000000000000000000 ) ) ;
#27187=CIRCLE ( 'NONE', #23265, 0.1000000000000028644 ) ;
#27217=DIRECTION ( 'NONE',  ( 1.000000000000000000, 0.000000000000000000, -0.000000000000000000 ) ) ;
#27224=CARTESIAN_POINT ( 'NONE',  ( -21.14999999999994174, 87.50449464844290048, -37.85861909827351468 ) ) ;
#27242=DIRECTION ( 'NONE',  ( 0.000000000000000000, 0.000000000000000000, 1.000000000000000000 ) ) ;
#27258=DIRECTION ( 'NONE',  ( 0.000000000000000000, 0.000000000000000000, 1.000000000000000000 ) ) ;
#27331=DIRECTION ( 'NONE',  ( 0.000000000000000000, 0.000000000000000000, 1.000000000000000000 ) ) ;
#27350=ORIENTED_EDGE ( 'NONE', *, *, #253920, .F. ) ;
#27461=DIRECTION ( 'NONE',  ( 0.000000000000000000, 0.000000000000000000, -1.000000000000000000 ) ) ;
#27508=ADVANCED_FACE ( 'NONE', ( #172913 ), #252378, .T. ) ;
#27561=ORIENTED_EDGE ( 'NONE', *, *, #72035, .F. ) ;
#27615=AXIS2_PLACEMENT_3D ( 'NONE', #111673, #66127, #145651 ) ;
#27624=EDGE_CURVE ( 'NONE', #222419, #64966, #164682, .T. ) ;
#27633=CYLINDRICAL_SURFACE ( 'NONE', #190890, 0.09999999999999939493 ) ;
#27638=CIRCLE ( 'NONE', #156804, 0.1000000000000032391 ) ;
#27786=LINE ( 'NONE', #249383, #68062 ) ;
#27797=LINE ( 'NONE', #146397, #91083 ) ;
#27845=AXIS2_PLACEMENT_3D ( 'NONE', #38076, #97999, #134563 ) ;
#27931=CIRCLE ( 'NONE', #173698, 0.1000000000000028644 ) ;
#27975=DIRECTION ( 'NONE',  ( 0.000000000000000000, 0.000000000000000000, 1.000000000000000000 ) ) ;
#27983=CARTESIAN_POINT ( 'NONE',  ( 23.50000000000005684, 78.05591623545335267, -49.16694968567509250 ) ) ;
#28051=DIRECTION ( 'NONE',  ( 1.000000000000000000, 0.000000000000000000, 0.000000000000000000 ) ) ;
#28126=ORIENTED_EDGE ( 'NONE', *, *, #209683, .T. ) ;
#28143=AXIS2_PLACEMENT_3D ( 'NONE', #199475, #20843, #80766 ) ;
#28221=CIRCLE ( 'NONE', #20012, 0.09999999999999939493 ) ;
#28239=CARTESIAN_POINT ( 'NONE',  ( 23.40000000000005542, 82.72707916847673459, -26.51159310135756897 ) ) ;
#28273=AXIS2_PLACEMENT_3D ( 'NONE', #17336, #57718, #156867 ) ;
#28301=DIRECTION ( 'NONE',  ( 1.000000000000000000, 0.000000000000000000, 0.000000000000000000 ) ) ;
#28383=VERTEX_POINT ( 'NONE', #92705 ) ;
#28434=VERTEX_POINT ( 'NONE', #232253 ) ;
#28486=DIRECTION ( 'NONE',  ( 1.000000000000000000, -0.000000000000000000, -0.000000000000000000 ) ) ;
#28507=DIRECTION ( 'NONE',  ( 0.000000000000000000, 0.000000000000000000, 1.000000000000000000 ) ) ;
#28545=VECTOR ( 'NONE', #22285, 1000.000000000000000 ) ;
#28575=AXIS2_PLACEMENT_3D ( 'NONE', #124355, #25266, #205145 ) ;
#28595=EDGE_CURVE ( 'NONE', #6953, #15908, #102461, .T. ) ;
#28608=CIRCLE ( 'NONE', #61306, 0.09999999999999530098 ) ;
#28655=CARTESIAN_POINT ( 'NONE',  ( -5.999999999999938716, 64.75000000001119815, -22.02310748452479316 ) ) ;
#28690=DIRECTION ( 'NONE',  ( 1.000000000000000000, 0.000000000000000000, 0.000000000000000000 ) ) ;
#28785=CIRCLE ( 'NONE', #203523, 0.1000000000000032391 ) ;
#28843=AXIS2_PLACEMENT_3D ( 'NONE', #196713, #216272, #199299 ) ;
#28872=EDGE_LOOP ( 'NONE', ( #44899, #120045, #167856, #246607 ) ) ;
#28897=EDGE_CURVE ( 'NONE', #234836, #191279, #141476, .T. ) ;
#28919=ORIENTED_EDGE ( 'NONE', *, *, #155742, .F. ) ;
#28922=DIRECTION ( 'NONE',  ( 0.000000000000000000, -0.1332476588733448597, 0.9910827722268067408 ) ) ;
#28959=DIRECTION ( 'NONE',  ( 0.000000000000000000, 0.000000000000000000, -1.000000000000000000 ) ) ;
#28960=CARTESIAN_POINT ( 'NONE',  ( 13.40000000000005898, 66.35000000001119247, -21.02310748452479316 ) ) ;
#29069=TOROIDAL_SURFACE ( 'NONE', #83144, 11.65000000000000036, 0.1000000000000000056 ) ;
#29073=FACE_OUTER_BOUND ( 'NONE', #35595, .T. ) ;
#29091=DIRECTION ( 'NONE',  ( 0.000000000000000000, 0.000000000000000000, -1.000000000000000000 ) ) ;
#29093=EDGE_CURVE ( 'NONE', #253828, #145505, #165429, .T. ) ;
#29123=DIRECTION ( 'NONE',  ( 1.000000000000000000, 0.000000000000000000, 0.000000000000000000 ) ) ;
#29127=CARTESIAN_POINT ( 'NONE',  ( 20.95000000000005258, 66.25000000001119815, -6.023107484524794941 ) ) ;
#29139=DIRECTION ( 'NONE',  ( 0.000000000000000000, -0.9910827722268055195, 0.1332476588733540468 ) ) ;
#29162=DIRECTION ( 'NONE',  ( 0.000000000000000000, 0.000000000000000000, -1.000000000000000000 ) ) ;
#29193=CIRCLE ( 'NONE', #158362, 0.09999999999999939493 ) ;
#29198=EDGE_CURVE ( 'NONE', #88017, #178217, #98729, .T. ) ;
#29258=DIRECTION ( 'NONE',  ( 1.000000000000000000, 0.000000000000000000, 0.000000000000000000 ) ) ;
#29267=CIRCLE ( 'NONE', #245698, 4.049999999999998046 ) ;
#29269=AXIS2_PLACEMENT_3D ( 'NONE', #186584, #13087, #229558 ) ;
#29288=ORIENTED_EDGE ( 'NONE', *, *, #55209, .F. ) ;
#29300=DIRECTION ( 'NONE',  ( 0.000000000000000000, 0.000000000000000000, 1.000000000000000000 ) ) ;
#29307=EDGE_CURVE ( 'NONE', #175937, #15261, #61356, .T. ) ;
#29320=CARTESIAN_POINT ( 'NONE',  ( -40.23850191057533010, 87.75000000001119815, -4.523107484524794053 ) ) ;
#29322=VERTEX_POINT ( 'NONE', #227123 ) ;
#29335=DIRECTION ( 'NONE',  ( 1.000000000000000000, 0.000000000000000000, 0.000000000000000000 ) ) ;
#29369=DIRECTION ( 'NONE',  ( 0.000000000000000000, -0.1480365673253065117, 0.9889818879709274535 ) ) ;
#29406=EDGE_LOOP ( 'NONE', ( #26714, #104894 ) ) ;
#29463=CARTESIAN_POINT ( 'NONE',  ( -11.59999999999994458, 64.35000000001120668, -23.62310748452479103 ) ) ;
#29487=AXIS2_PLACEMENT_3D ( 'NONE', #208975, #256722, #18162 ) ;
#29502=EDGE_CURVE ( 'NONE', #150745, #20544, #147488, .T. ) ;
#29525=CARTESIAN_POINT ( 'NONE',  ( -23.39999999999994529, 76.00000000001119815, -40.07310748452479032 ) ) ;
#29554=ADVANCED_FACE ( 'NONE', ( #73233 ), #56182, .T. ) ;
#29578=CARTESIAN_POINT ( 'NONE',  ( -23.49999999999994316, 87.60324567546805952, -37.87437456276921210 ) ) ;
#29585=AXIS2_PLACEMENT_3D ( 'NONE', #238854, #139730, #120231 ) ;
#29630=DIRECTION ( 'NONE',  ( -1.000000000000000000, -0.000000000000000000, -0.000000000000000000 ) ) ;
#29631=ADVANCED_FACE ( 'NONE', ( #135725 ), #101664, .F. ) ;
#29728=CARTESIAN_POINT ( 'NONE',  ( 23.40000000000005542, 74.16448838626247664, -47.52760213295649550 ) ) ;
#29740=AXIS2_PLACEMENT_3D ( 'NONE', #74087, #151034, #93616 ) ;
#29860=ORIENTED_EDGE ( 'NONE', *, *, #176621, .T. ) ;
#29901=ORIENTED_EDGE ( 'NONE', *, *, #88526, .T. ) ;
#29995=DIRECTION ( 'NONE',  ( -1.000000000000000000, 0.000000000000000000, 0.000000000000000000 ) ) ;
#30001=SPHERICAL_SURFACE ( 'NONE', #156225, 0.1000000000000000056 ) ;
#30027=EDGE_CURVE ( 'NONE', #150828, #24890, #143107, .T. ) ;
#30080=EDGE_CURVE ( 'NONE', #1569, #119358, #240949, .T. ) ;
#30110=VERTEX_POINT ( 'NONE', #126109 ) ;
#30121=ORIENTED_EDGE ( 'NONE', *, *, #157124, .F. ) ;
#30166=VECTOR ( 'NONE', #14806, 1000.000000000000000 ) ;
#30190=EDGE_CURVE ( 'NONE', #153040, #53024, #93497, .T. ) ;
#30197=ORIENTED_EDGE ( 'NONE', *, *, #48637, .F. ) ;
#30200=ORIENTED_EDGE ( 'NONE', *, *, #131741, .F. ) ;
#30206=CARTESIAN_POINT ( 'NONE',  ( 23.40000000000004476, 77.16254490893143725, -44.02310748452479316 ) ) ;
#30214=CARTESIAN_POINT ( 'NONE',  ( 21.15000000000005187, 87.60324567546805952, -37.87437456276921210 ) ) ;
#30228=EDGE_CURVE ( 'NONE', #167941, #141859, #156078, .T. ) ;
#30250=VERTEX_POINT ( 'NONE', #94694 ) ;
#30307=CARTESIAN_POINT ( 'NONE',  ( -13.39999999999994529, 64.25000000001119815, -23.72310748452479245 ) ) ;
#30313=VERTEX_POINT ( 'NONE', #16475 ) ;
#30345=FACE_BOUND ( 'NONE', #90075, .T. ) ;
#30352=( NAMED_UNIT ( * ) SI_UNIT ( $, .STERADIAN. ) SOLID_ANGLE_UNIT ( ) );
#30358=EDGE_LOOP ( 'NONE', ( #103076, #100172, #84483, #32103 ) ) ;
#30372=ORIENTED_EDGE ( 'NONE', *, *, #81123, .T. ) ;
#30416=AXIS2_PLACEMENT_3D ( 'NONE', #182361, #222738, #44127 ) ;
#30427=VERTEX_POINT ( 'NONE', #221055 ) ;
#30437=CYLINDRICAL_SURFACE ( 'NONE', #184229, 0.09999999999999982514 ) ;
#30526=CIRCLE ( 'NONE', #226105, 11.65000000000000036 ) ;
#30527=CIRCLE ( 'NONE', #242696, 0.1000000000000002554 ) ;
#30541=SPHERICAL_SURFACE ( 'NONE', #8920, 0.1000000000000000056 ) ;
#30573=CARTESIAN_POINT ( 'NONE',  ( -23.39999999999994529, 83.90000000001120384, -34.77310748452479316 ) ) ;
#30704=EDGE_LOOP ( 'NONE', ( #65613, #54999, #195544, #31991 ) ) ;
#30760=ORIENTED_EDGE ( 'NONE', *, *, #78503, .T. ) ;
#30770=CARTESIAN_POINT ( 'NONE',  ( 21.05000000000005400, 74.83745509109094485, -44.02310748452479316 ) ) ;
#30848=CARTESIAN_POINT ( 'NONE',  ( 23.40000000000005187, 87.60324567546805952, -37.87437456276921210 ) ) ;
#30852=AXIS2_PLACEMENT_3D ( 'NONE', #25967, #185026, #166785 ) ;
#30888=CARTESIAN_POINT ( 'NONE',  ( 23.40000000000005187, 74.94272479589878344, -8.023107484524793165 ) ) ;
#30957=AXIS2_PLACEMENT_3D ( 'NONE', #28960, #90141, #108448 ) ;
#31001=CARTESIAN_POINT ( 'NONE',  ( -21.14999999999994174, 64.35000000001120668, -3.023107484524792277 ) ) ;
#31021=CARTESIAN_POINT ( 'NONE',  ( 5.551115123125782702E-14, 67.65000000001118963, -3.023107484524792277 ) ) ;
#31047=LINE ( 'NONE', #147086, #83279 ) ;
#31049=AXIS2_PLACEMENT_3D ( 'NONE', #193404, #153011, #33076 ) ;
#31055=DIRECTION ( 'NONE',  ( 0.000000000000000000, -0.9910827722268049644, 0.1332476588733589318 ) ) ;
#31119=AXIS2_PLACEMENT_3D ( 'NONE', #147910, #227425, #118396 ) ;
#31198=DIRECTION ( 'NONE',  ( -1.284434275755705296E-16, 0.7071067811865471286, -0.7071067811865479058 ) ) ;
#31254=CARTESIAN_POINT ( 'NONE',  ( -20.94999999999994600, 65.15000000001120384, -51.02310748452479316 ) ) ;
#31302=CARTESIAN_POINT ( 'NONE',  ( 21.15000000000005542, 76.00000000001119815, -3.123107484524795474 ) ) ;
#31368=CYLINDRICAL_SURFACE ( 'NONE', #188182, 0.09999999999999939493 ) ;
#31370=ORIENTED_EDGE ( 'NONE', *, *, #107579, .F. ) ;
#31387=CYLINDRICAL_SURFACE ( 'NONE', #29269, 0.1000000000000028644 ) ;
#31451=ORIENTED_EDGE ( 'NONE', *, *, #85489, .F. ) ;
#31474=CARTESIAN_POINT ( 'NONE',  ( 23.50000000000005684, 76.00000000001119815, -36.02310748452479316 ) ) ;
#31475=CARTESIAN_POINT ( 'NONE',  ( -23.49999999999994316, 74.26359666348515987, -47.54092689884382850 ) ) ;
#31542=VECTOR ( 'NONE', #120140, 1000.000000000000000 ) ;
#31566=ORIENTED_EDGE ( 'NONE', *, *, #25457, .F. ) ;
#31619=AXIS2_PLACEMENT_3D ( 'NONE', #32297, #109225, #188769 ) ;
#31622=ORIENTED_EDGE ( 'NONE', *, *, #150792, .F. ) ;
#31694=ORIENTED_EDGE ( 'NONE', *, *, #17871, .T. ) ;
#31723=EDGE_CURVE ( 'NONE', #42311, #77787, #85257, .T. ) ;
#31736=CARTESIAN_POINT ( 'NONE',  ( -21.04999999999994387, 76.00000000001119815, -36.02310748452479316 ) ) ;
#31741=CARTESIAN_POINT ( 'NONE',  ( 21.15000000000005542, 76.00000000001119815, -3.123107484524795474 ) ) ;
#31767=AXIS2_PLACEMENT_3D ( 'NONE', #87931, #228769, #110082 ) ;
#31793=LINE ( 'NONE', #111301, #215456 ) ;
#31796=DIRECTION ( 'NONE',  ( -1.000000000000000000, 0.000000000000000000, 0.000000000000000000 ) ) ;
#31849=ORIENTED_EDGE ( 'NONE', *, *, #241026, .F. ) ;
#31921=CARTESIAN_POINT ( 'NONE',  ( -21.14999999999994174, 74.83745509109094485, -43.92310748452479885 ) ) ;
#31939=ADVANCED_FACE ( 'NONE', ( #14802 ), #185442, .T. ) ;
#31942=DIRECTION ( 'NONE',  ( 1.000000000000000000, 0.000000000000000000, 0.000000000000000000 ) ) ;
#31951=DIRECTION ( 'NONE',  ( 0.000000000000000000, 0.000000000000000000, -1.000000000000000000 ) ) ;
#31991=ORIENTED_EDGE ( 'NONE', *, *, #44106, .F. ) ;
#32046=DIRECTION ( 'NONE',  ( 0.000000000000000000, 0.000000000000000000, 1.000000000000000000 ) ) ;
#32072=CIRCLE ( 'NONE', #223557, 0.09999999999999530098 ) ;
#32103=ORIENTED_EDGE ( 'NONE', *, *, #35005, .F. ) ;
#32164=DIRECTION ( 'NONE',  ( -1.000000000000000000, 0.000000000000000000, 0.000000000000000000 ) ) ;
#32252=EDGE_LOOP ( 'NONE', ( #77552, #66453, #184306, #12634, #12682, #110240, #39806, #206284, #110789, #205045, #112973, #74274, #100981, #7567, #45989, #206010, #178838, #230447, #767, #166948, #45451, #173025, #254600 ) ) ;
#32296=ORIENTED_EDGE ( 'NONE', *, *, #40549, .T. ) ;
#32297=CARTESIAN_POINT ( 'NONE',  ( 21.15000000000005187, 64.35000000001120668, -51.02310748452479316 ) ) ;
#32338=ORIENTED_EDGE ( 'NONE', *, *, #80584, .F. ) ;
#32348=DIRECTION ( 'NONE',  ( 0.000000000000000000, 0.000000000000000000, 1.000000000000000000 ) ) ;
#32410=VECTOR ( 'NONE', #112280, 1000.000000000000000 ) ;
#32474=AXIS2_PLACEMENT_3D ( 'NONE', #2432, #199391, #40337 ) ;
#32508=EDGE_LOOP ( 'NONE', ( #229177, #61659, #83499 ) ) ;
#32543=EDGE_LOOP ( 'NONE', ( #163790, #202314, #210711, #164596 ) ) ;
#32566=ORIENTED_EDGE ( 'NONE', *, *, #239328, .T. ) ;
#32575=ORIENTED_EDGE ( 'NONE', *, *, #97664, .F. ) ;
#32636=AXIS2_PLACEMENT_3D ( 'NONE', #56262, #177553, #159255 ) ;
#32708=VERTEX_POINT ( 'NONE', #54555 ) ;
#32751=ADVANCED_FACE ( 'NONE', ( #216183 ), #117109, .F. ) ;
#32796=DIRECTION ( 'NONE',  ( 0.000000000000000000, -0.000000000000000000, -1.000000000000000000 ) ) ;
#32820=DIRECTION ( 'NONE',  ( -0.000000000000000000, -0.1480365673253065117, 0.9889818879709273425 ) ) ;
#32823=DIRECTION ( 'NONE',  ( 1.000000000000000000, -0.000000000000000000, -0.000000000000000000 ) ) ;
#32827=VECTOR ( 'NONE', #177854, 1000.000000000000000 ) ;
#32906=EDGE_CURVE ( 'NONE', #179303, #143490, #35966, .T. ) ;
#32943=DIRECTION ( 'NONE',  ( 1.000000000000000000, 0.000000000000000000, 0.000000000000000000 ) ) ;
#32949=EDGE_CURVE ( 'NONE', #107789, #1569, #227473, .T. ) ;
#32963=LINE ( 'NONE', #111175, #43856 ) ;
#32967=DIRECTION ( 'NONE',  ( 0.000000000000000000, -0.4856429311786307768, -0.8741572761215385956 ) ) ;
#33018=CARTESIAN_POINT ( 'NONE',  ( -21.14999999999994174, 67.85000000001119247, -3.123107484524795474 ) ) ;
#33031=VERTEX_POINT ( 'NONE', #7407 ) ;
#33054=ADVANCED_FACE ( 'NONE', ( #144331 ), #146907, .T. ) ;
#33076=DIRECTION ( 'NONE',  ( 0.000000000000000000, -0.1332476588733448597, 0.9910827722268067408 ) ) ;
#33086=VERTEX_POINT ( 'NONE', #149523 ) ;
#33153=CIRCLE ( 'NONE', #4077, 4.150000000000001243 ) ;
#33161=ORIENTED_EDGE ( 'NONE', *, *, #44961, .F. ) ;
#33176=EDGE_CURVE ( 'NONE', #243985, #250992, #232914, .T. ) ;
#33217=VECTOR ( 'NONE', #79735, 1000.000000000000000 ) ;
#33244=AXIS2_PLACEMENT_3D ( 'NONE', #131879, #32823, #229702 ) ;
#33246=CARTESIAN_POINT ( 'NONE',  ( -5.899999999999938183, 64.65000000001120384, -22.12310748452479103 ) ) ;
#33262=DIRECTION ( 'NONE',  ( -1.000000000000000000, 0.000000000000000000, 0.000000000000000000 ) ) ;
#33263=CARTESIAN_POINT ( 'NONE',  ( 20.95000000000005258, 87.75000000001119815, -4.623107484524796362 ) ) ;
#33283=DIRECTION ( 'NONE',  ( 0.000000000000000000, 0.9910827722268049644, -0.1332476588733589318 ) ) ;
#33287=AXIS2_PLACEMENT_3D ( 'NONE', #41331, #219938, #96124 ) ;
#33334=DIRECTION ( 'NONE',  ( -1.000000000000000000, 5.467925025959462129E-15, 3.427148797533442008E-14 ) ) ;
#33353=CIRCLE ( 'NONE', #58232, 0.1000000000000021844 ) ;
#33358=SPHERICAL_SURFACE ( 'NONE', #54474, 0.1000000000000000056 ) ;
#33403=DIRECTION ( 'NONE',  ( 0.000000000000000000, 0.000000000000000000, 1.000000000000000000 ) ) ;
#33428=DIRECTION ( 'NONE',  ( -0.000000000000000000, 1.000000000000000000, -0.000000000000000000 ) ) ;
#33437=EDGE_CURVE ( 'NONE', #176509, #73651, #32072, .T. ) ;
#33444=ADVANCED_FACE ( 'NONE', ( #163630 ), #144039, .F. ) ;
#33479=DIRECTION ( 'NONE',  ( 0.000000000000000000, 0.1332476588733636502, -0.9910827722268044093 ) ) ;
#33497=CARTESIAN_POINT ( 'NONE',  ( -21.04999999999994387, 74.63923853664559260, -43.99645795275012006 ) ) ;
#33507=DIRECTION ( 'NONE',  ( 1.000000000000000000, 0.000000000000000000, 0.000000000000000000 ) ) ;
#33512=VERTEX_POINT ( 'NONE', #79589 ) ;
#33546=CARTESIAN_POINT ( 'NONE',  ( -13.39999999999994351, 64.35000000001120668, -18.42310748452479174 ) ) ;
#33561=ORIENTED_EDGE ( 'NONE', *, *, #200124, .T. ) ;
#33593=PLANE ( 'NONE',  #168187 ) ;
#33613=VERTEX_POINT ( 'NONE', #103008 ) ;
#33632=DIRECTION ( 'NONE',  ( 0.000000000000000000, 0.000000000000000000, -1.000000000000000000 ) ) ;
#33653=ADVANCED_FACE ( 'NONE', ( #139564 ), #202916, .T. ) ;
#33665=ORIENTED_EDGE ( 'NONE', *, *, #2437, .F. ) ;
#33715=CARTESIAN_POINT ( 'NONE',  ( 21.15000000000005542, 77.36076146337680370, -43.99645795275012006 ) ) ;
#33719=VECTOR ( 'NONE', #98133, 1000.000000000000000 ) ;
#33759=CARTESIAN_POINT ( 'NONE',  ( -0.8999999999999437339, 67.75000000001118394, -10.02310748452479139 ) ) ;
#33801=ORIENTED_EDGE ( 'NONE', *, *, #3089, .F. ) ;
#33821=CARTESIAN_POINT ( 'NONE',  ( 11.60000000000006004, 67.75000000001118394, -21.02310748452479316 ) ) ;
#33860=CARTESIAN_POINT ( 'NONE',  ( -40.23850191057533010, 87.75000000001122658, -30.02310748452481448 ) ) ;
#33972=EDGE_CURVE ( 'NONE', #230960, #161116, #140543, .T. ) ;
#34000=ORIENTED_EDGE ( 'NONE', *, *, #17355, .F. ) ;
#34081=CIRCLE ( 'NONE', #179799, 0.09999999999999939493 ) ;
#34097=ORIENTED_EDGE ( 'NONE', *, *, #15219, .T. ) ;
#34162=EDGE_CURVE ( 'NONE', #131851, #191399, #11779, .T. ) ;
#34318=LINE ( 'NONE', #78538, #71779 ) ;
#34334=TOROIDAL_SURFACE ( 'NONE', #225804, 0.2000000000000000111, 0.1000000000000000056 ) ;
#34352=VERTEX_POINT ( 'NONE', #155982 ) ;
#34360=ORIENTED_EDGE ( 'NONE', *, *, #180033, .F. ) ;
#34437=VECTOR ( 'NONE', #52758, 1000.000000000000000 ) ;
#34473=ORIENTED_EDGE ( 'NONE', *, *, #134741, .T. ) ;
#34482=ORIENTED_EDGE ( 'NONE', *, *, #186650, .F. ) ;
#34533=DIRECTION ( 'NONE',  ( 0.000000000000000000, 0.000000000000000000, 1.000000000000000000 ) ) ;
#34545=ORIENTED_EDGE ( 'NONE', *, *, #175702, .F. ) ;
#34576=ORIENTED_EDGE ( 'NONE', *, *, #229330, .T. ) ;
#34577=VECTOR ( 'NONE', #115540, 1000.000000000000000 ) ;
#34580=CARTESIAN_POINT ( 'NONE',  ( -5.999999999999938716, 64.35000000001120668, -22.02310748452479316 ) ) ;
#34584=ORIENTED_EDGE ( 'NONE', *, *, #157293, .F. ) ;
#34585=AXIS2_PLACEMENT_3D ( 'NONE', #30888, #110382, #10006 ) ;
#34689=CARTESIAN_POINT ( 'NONE',  ( 21.15000000000005542, 87.50449464844290048, -34.18759587077607165 ) ) ;
#34717=AXIS2_PLACEMENT_3D ( 'NONE', #94664, #174257, #38554 ) ;
#34718=AXIS2_PLACEMENT_3D ( 'NONE', #108093, #88489, #148502 ) ;
#34730=EDGE_CURVE ( 'NONE', #46490, #88642, #106277, .T. ) ;
#34751=ORIENTED_EDGE ( 'NONE', *, *, #94673, .F. ) ;
#34769=CYLINDRICAL_SURFACE ( 'NONE', #190139, 0.09999999999999939493 ) ;
#34928=DIRECTION ( 'NONE',  ( 0.000000000000000000, 0.000000000000000000, 1.000000000000000000 ) ) ;
#34933=VERTEX_POINT ( 'NONE', #252220 ) ;
#34973=DIRECTION ( 'NONE',  ( 0.000000000000000000, 0.000000000000000000, -1.000000000000000000 ) ) ;
#35004=EDGE_CURVE ( 'NONE', #182432, #114575, #73628, .T. ) ;
#35005=EDGE_CURVE ( 'NONE', #252143, #19078, #256026, .T. ) ;
#35042=EDGE_CURVE ( 'NONE', #80585, #216962, #245169, .T. ) ;
#35094=CARTESIAN_POINT ( 'NONE',  ( 23.40000000000005187, 87.50449464844290048, -34.18759587077607165 ) ) ;
#35107=AXIS2_PLACEMENT_3D ( 'NONE', #119620, #175751, #98713 ) ;
#35117=ORIENTED_EDGE ( 'NONE', *, *, #32949, .F. ) ;
#35134=TOROIDAL_SURFACE ( 'NONE', #147527, 0.2000000000000000111, 0.1000000000000000056 ) ;
#35194=CARTESIAN_POINT ( 'NONE',  ( 0.9000000000000547562, 67.75000000001118394, -12.62310748452478926 ) ) ;
#35250=DIRECTION ( 'NONE',  ( -1.000000000000000000, 0.000000000000000000, 0.000000000000000000 ) ) ;
#35308=DIRECTION ( 'NONE',  ( 0.000000000000000000, -0.8741572761215280485, 0.4856429311786498171 ) ) ;
#35309=CARTESIAN_POINT ( 'NONE',  ( -23.49999999999994316, 87.60324567546805952, -37.87437456276921210 ) ) ;
#35334=VECTOR ( 'NONE', #64360, 1000.000000000000000 ) ;
#35372=FACE_OUTER_BOUND ( 'NONE', #182739, .T. ) ;
#35375=DIRECTION ( 'NONE',  ( 1.000000000000000000, 0.000000000000000000, 0.000000000000000000 ) ) ;
#35528=CARTESIAN_POINT ( 'NONE',  ( -40.23850191057533010, 65.19115966511134275, -29.92310748452479174 ) ) ;
#35563=EDGE_CURVE ( 'NONE', #107789, #3259, #41366, .T. ) ;
#35595=EDGE_LOOP ( 'NONE', ( #24911, #27079, #5698, #56755 ) ) ;
#35611=LINE ( 'NONE', #98079, #84610 ) ;
#35639=DIRECTION ( 'NONE',  ( -1.000000000000000000, 0.000000000000000000, 0.000000000000000000 ) ) ;
#35664=ADVANCED_FACE ( 'NONE', ( #193910 ), #37250, .T. ) ;
#35753=DIRECTION ( 'NONE',  ( 0.000000000000000000, -0.7071067811865479058, -0.7071067811865472397 ) ) ;
#35800=FACE_OUTER_BOUND ( 'NONE', #202502, .T. ) ;
#35823=ORIENTED_EDGE ( 'NONE', *, *, #114958, .F. ) ;
#35839=VERTEX_POINT ( 'NONE', #96062 ) ;
#35841=DIRECTION ( 'NONE',  ( 0.000000000000000000, 0.000000000000000000, -1.000000000000000000 ) ) ;
#35896=EDGE_LOOP ( 'NONE', ( #157198, #161187, #192107, #181373 ) ) ;
#35960=FACE_OUTER_BOUND ( 'NONE', #206442, .T. ) ;
#35966=CIRCLE ( 'NONE', #206641, 0.09999999999999982514 ) ;
#36008=EDGE_LOOP ( 'NONE', ( #88239, #140014, #60653, #116586 ) ) ;
#36010=VECTOR ( 'NONE', #169131, 1000.000000000000000 ) ;
#36043=CARTESIAN_POINT ( 'NONE',  ( -21.14999999999994174, 84.00000000001119815, -34.86056257560453986 ) ) ;
#36051=DIRECTION ( 'NONE',  ( 0.000000000000000000, -0.000000000000000000, 1.000000000000000000 ) ) ;
#36069=DIRECTION ( 'NONE',  ( 0.000000000000000000, 0.1575546449569757979, 0.9875102702516471709 ) ) ;
#36112=ORIENTED_EDGE ( 'NONE', *, *, #161700, .F. ) ;
#36128=CARTESIAN_POINT ( 'NONE',  ( -23.49999999999994316, 83.90000000001120384, -34.77310748452479316 ) ) ;
#36151=CARTESIAN_POINT ( 'NONE',  ( 11.60000000000006004, 64.25000000001119815, -23.72310748452479601 ) ) ;
#36155=FACE_OUTER_BOUND ( 'NONE', #178887, .T. ) ;
#36158=VERTEX_POINT ( 'NONE', #116617 ) ;
#36173=DIRECTION ( 'NONE',  ( 0.000000000000000000, 0.000000000000000000, -1.000000000000000000 ) ) ;
#36187=EDGE_LOOP ( 'NONE', ( #238784, #147611, #59854, #21313 ) ) ;
#36219=ORIENTED_EDGE ( 'NONE', *, *, #83120, .F. ) ;
#36221=DIRECTION ( 'NONE',  ( 1.000000000000000000, -3.427148797533456523E-14, 5.467925025959484217E-15 ) ) ;
#36383=EDGE_CURVE ( 'NONE', #113855, #97476, #95301, .T. ) ;
#36386=DIRECTION ( 'NONE',  ( 0.000000000000000000, 0.1575546449569757979, -0.9875102702516471709 ) ) ;
#36407=DIRECTION ( 'NONE',  ( 0.000000000000000000, -0.9875102702516471709, 0.1575546449569757979 ) ) ;
#36412=EDGE_CURVE ( 'NONE', #30313, #23353, #99929, .T. ) ;
#36461=CARTESIAN_POINT ( 'NONE',  ( 11.60000000000006004, 67.72071067812984779, -17.05239680640613997 ) ) ;
#36484=ORIENTED_EDGE ( 'NONE', *, *, #222834, .T. ) ;
#36516=TOROIDAL_SURFACE ( 'NONE', #73922, 4.150000000000000355, 0.1000000000000000056 ) ;
#36533=DIRECTION ( 'NONE',  ( 0.000000000000000000, 0.000000000000000000, -1.000000000000000000 ) ) ;
#36637=ORIENTED_EDGE ( 'NONE', *, *, #199609, .T. ) ;
#36743=ORIENTED_EDGE ( 'NONE', *, *, #198891, .F. ) ;
#36763=EDGE_LOOP ( 'NONE', ( #129007, #38564, #67896, #80029 ) ) ;
#36774=DIRECTION ( 'NONE',  ( 1.000000000000000000, -0.000000000000000000, 0.000000000000000000 ) ) ;
#36787=ORIENTED_EDGE ( 'NONE', *, *, #171652, .T. ) ;
#36809=DIRECTION ( 'NONE',  ( 1.000000000000000000, 0.000000000000000000, -0.000000000000000000 ) ) ;
#36836=CIRCLE ( 'NONE', #182566, 0.1000000000000002554 ) ;
#36879=CIRCLE ( 'NONE', #182605, 0.09999999999999939493 ) ;
#36884=TOROIDAL_SURFACE ( 'NONE', #182608, 0.2000000000000000111, 0.1000000000000000056 ) ;
#36896=LINE ( 'NONE', #61561, #16560 ) ;
#36933=CARTESIAN_POINT ( 'NONE',  ( 21.15000000000005187, 83.90000000001120384, -34.77310748452479316 ) ) ;
#36941=DIRECTION ( 'NONE',  ( 1.000000000000000000, 0.000000000000000000, 0.000000000000000000 ) ) ;
#36988=AXIS2_PLACEMENT_3D ( 'NONE', #78228, #161655, #62533 ) ;
#37090=DIRECTION ( 'NONE',  ( 0.000000000000000000, -0.9910827722268049644, 0.1332476588733589318 ) ) ;
#37111=ADVANCED_FACE ( 'NONE', ( #160304 ), #83143, .T. ) ;
#37130=CARTESIAN_POINT ( 'NONE',  ( -23.39999999999994529, 74.83745509109094485, -43.82310748452479743 ) ) ;
#37242=ORIENTED_EDGE ( 'NONE', *, *, #2812, .F. ) ;
#37248=DIRECTION ( 'NONE',  ( -1.000000000000000000, 0.000000000000000000, 0.000000000000000000 ) ) ;
#37250=TOROIDAL_SURFACE ( 'NONE', #182997, 0.2000000000000000111, 0.1000000000000000056 ) ;
#37270=ORIENTED_EDGE ( 'NONE', *, *, #72035, .T. ) ;
#37314=CARTESIAN_POINT ( 'NONE',  ( -23.49999999999994316, 84.00000000001119815, -34.86056257560453986 ) ) ;
#37315=DIRECTION ( 'NONE',  ( -1.000000000000000000, 0.000000000000000000, 0.000000000000000000 ) ) ;
#37338=CARTESIAN_POINT ( 'NONE',  ( -21.14999999999994174, 74.73834681386826162, -44.00978271863746016 ) ) ;
#37349=ORIENTED_EDGE ( 'NONE', *, *, #13983, .F. ) ;
#37375=CARTESIAN_POINT ( 'NONE',  ( -13.39999999999994529, 67.72071067812984779, -24.99381816264344991 ) ) ;
#37435=VECTOR ( 'NONE', #134079, 1000.000000000000000 ) ;
#37477=ORIENTED_EDGE ( 'NONE', *, *, #117834, .F. ) ;
#37479=FACE_OUTER_BOUND ( 'NONE', #48186, .T. ) ;
#37494=DIRECTION ( 'NONE',  ( 0.000000000000000000, 0.000000000000000000, 1.000000000000000000 ) ) ;
#37497=DIRECTION ( 'NONE',  ( 0.000000000000000000, 0.9889818879709272315, 0.1480365673253073999 ) ) ;
#37510=DIRECTION ( 'NONE',  ( 1.000000000000000000, 0.000000000000000000, 0.000000000000000000 ) ) ;
#37556=ADVANCED_FACE ( 'NONE', ( #241742 ), #61833, .T. ) ;
#37603=ORIENTED_EDGE ( 'NONE', *, *, #101397, .T. ) ;
#37663=DIRECTION ( 'NONE',  ( 0.000000000000000000, 0.000000000000000000, -1.000000000000000000 ) ) ;
#37681=DIRECTION ( 'NONE',  ( 0.000000000000000000, -1.000000000000000000, 0.000000000000000000 ) ) ;
#37752=DIRECTION ( 'NONE',  ( 1.000000000000000000, 0.000000000000000000, 0.000000000000000000 ) ) ;
#37770=DIRECTION ( 'NONE',  ( -4.282643121434362058E-15, 0.9875102702516478370, 0.1575546449569727447 ) ) ;
#37809=DIRECTION ( 'NONE',  ( -1.000000000000000000, -0.000000000000000000, -0.000000000000000000 ) ) ;
#37851=VERTEX_POINT ( 'NONE', #137199 ) ;
#37852=DIRECTION ( 'NONE',  ( 0.000000000000000000, 0.1332476588733589040, 0.9910827722268048534 ) ) ;
#37894=LINE ( 'NONE', #100382, #25935 ) ;
#37950=CIRCLE ( 'NONE', #25459, 0.09999999999999939493 ) ;
#37956=LINE ( 'NONE', #134439, #122531 ) ;
#37992=ADVANCED_FACE ( 'NONE', ( #126625 ), #96200, .T. ) ;
#37998=DIRECTION ( 'NONE',  ( 0.000000000000000000, 0.000000000000000000, -1.000000000000000000 ) ) ;
#38019=ORIENTED_EDGE ( 'NONE', *, *, #83120, .T. ) ;
#38065=DIRECTION ( 'NONE',  ( -1.000000000000000000, -0.000000000000000000, 0.000000000000000000 ) ) ;
#38073=LINE ( 'NONE', #41928, #138905 ) ;
#38076=CARTESIAN_POINT ( 'NONE',  ( -21.14999999999994174, 74.16448838626247664, -47.52760213295649550 ) ) ;
#38078=LINE ( 'NONE', #154201, #48164 ) ;
#38115=DIRECTION ( 'NONE',  ( 0.000000000000000000, -0.000000000000000000, 1.000000000000000000 ) ) ;
#38153=DIRECTION ( 'NONE',  ( 0.000000000000000000, 0.000000000000000000, -1.000000000000000000 ) ) ;
#38183=EDGE_CURVE ( 'NONE', #123360, #26051, #50391, .T. ) ;
#38189=EDGE_CURVE ( 'NONE', #74170, #117682, #154514, .T. ) ;
#38235=CARTESIAN_POINT ( 'NONE',  ( -0.8999999999999437339, 64.35000000001120668, -12.72310748452478890 ) ) ;
#38311=EDGE_CURVE ( 'NONE', #167673, #148669, #51042, .T. ) ;
#38317=ORIENTED_EDGE ( 'NONE', *, *, #235973, .F. ) ;
#38320=ADVANCED_FACE ( 'NONE', ( #116879 ), #79004, .T. ) ;
#38403=DIRECTION ( 'NONE',  ( 0.000000000000000000, 0.000000000000000000, -1.000000000000000000 ) ) ;
#38450=DIRECTION ( 'NONE',  ( -1.000000000000000000, -0.000000000000000000, 0.000000000000000000 ) ) ;
#38554=DIRECTION ( 'NONE',  ( 0.000000000000000000, 0.000000000000000000, -1.000000000000000000 ) ) ;
#38564=ORIENTED_EDGE ( 'NONE', *, *, #61929, .T. ) ;
#38569=AXIS2_PLACEMENT_3D ( 'NONE', #6339, #106718, #227973 ) ;
#38570=CARTESIAN_POINT ( 'NONE',  ( -21.14999999999994174, 84.00000000001119815, -37.18565239344504647 ) ) ;
#38590=CARTESIAN_POINT ( 'NONE',  ( -21.04999999999994387, 67.85000000001119247, -25.49719488170504533 ) ) ;
#38613=AXIS2_PLACEMENT_3D ( 'NONE', #80642, #83199, #1101 ) ;
#38614=VERTEX_POINT ( 'NONE', #222170 ) ;
#38633=DIRECTION ( 'NONE',  ( -1.444674012291107001E-15, 0.1332476588733650935, -0.9910827722268042983 ) ) ;
#38724=EDGE_LOOP ( 'NONE', ( #108239, #195940, #130204, #179754 ) ) ;
#38735=EDGE_CURVE ( 'NONE', #167673, #191399, #63736, .T. ) ;
#38749=AXIS2_PLACEMENT_3D ( 'NONE', #232529, #107412, #149132 ) ;
#38752=ORIENTED_EDGE ( 'NONE', *, *, #97664, .T. ) ;
#38832=AXIS2_PLACEMENT_3D ( 'NONE', #142800, #223631, #28051 ) ;
#38912=EDGE_LOOP ( 'NONE', ( #214633, #11531, #107837, #231440 ) ) ;
#38981=ORIENTED_EDGE ( 'NONE', *, *, #1338, .F. ) ;
#39035=DIRECTION ( 'NONE',  ( 0.000000000000000000, 0.000000000000000000, -1.000000000000000000 ) ) ;
#39093=LINE ( 'NONE', #1199, #172546 ) ;
#39101=EDGE_CURVE ( 'NONE', #33613, #252227, #77238, .T. ) ;
#39118=ORIENTED_EDGE ( 'NONE', *, *, #56475, .T. ) ;
#39172=ORIENTED_EDGE ( 'NONE', *, *, #78192, .F. ) ;
#39177=SPHERICAL_SURFACE ( 'NONE', #210730, 0.1000000000000000056 ) ;
#39179=ORIENTED_EDGE ( 'NONE', *, *, #215818, .T. ) ;
#39183=CIRCLE ( 'NONE', #93305, 4.049999999999998046 ) ;
#39197=EDGE_LOOP ( 'NONE', ( #151826, #230246, #159815, #242471 ) ) ;
#39222=DIRECTION ( 'NONE',  ( 0.000000000000000000, 0.000000000000000000, -1.000000000000000000 ) ) ;
#39273=EDGE_CURVE ( 'NONE', #143932, #64265, #84725, .T. ) ;
#39282=CARTESIAN_POINT ( 'NONE',  ( -23.39999999999994529, 74.16448838626247664, -47.52760213295649550 ) ) ;
#39283=VERTEX_POINT ( 'NONE', #113508 ) ;
#39290=CARTESIAN_POINT ( 'NONE',  ( -11.59999999999994458, 67.72071067812984779, -24.99381816264344991 ) ) ;
#39332=CARTESIAN_POINT ( 'NONE',  ( 6.000000000000060396, 64.35000000001120668, -26.02310748452479316 ) ) ;
#39338=VECTOR ( 'NONE', #234611, 999.9999999999998863 ) ;
#39348=ADVANCED_FACE ( 'NONE', ( #249180 ), #159784, .T. ) ;
#39368=CARTESIAN_POINT ( 'NONE',  ( 0.9000000000000547562, 64.35000000001120668, -12.62310748452478926 ) ) ;
#39369=ORIENTED_EDGE ( 'NONE', *, *, #1753, .T. ) ;
#39413=CARTESIAN_POINT ( 'NONE',  ( 23.50000000000005684, 74.94272479589878344, -3.123107484524795474 ) ) ;
#39444=DIRECTION ( 'NONE',  ( -0.000000000000000000, -0.9875102702516493913, 0.1575546449569621699 ) ) ;
#39446=AXIS2_PLACEMENT_3D ( 'NONE', #215036, #135480, #13015 ) ;
#39606=EDGE_LOOP ( 'NONE', ( #103083, #210435, #250986, #96131, #140529, #199645, #250132 ) ) ;
#39622=AXIS2_PLACEMENT_3D ( 'NONE', #170132, #249638, #190961 ) ;
#39628=ORIENTED_EDGE ( 'NONE', *, *, #68638, .T. ) ;
#39635=CARTESIAN_POINT ( 'NONE',  ( -5.999999999999938716, 64.65000000001120384, -22.12310748452479103 ) ) ;
#39761=DIRECTION ( 'NONE',  ( 0.000000000000000000, 0.9875102702516498354, 0.1575546449569600882 ) ) ;
#39793=EDGE_LOOP ( 'NONE', ( #225587, #63086, #247735, #76844 ) ) ;
#39806=ORIENTED_EDGE ( 'NONE', *, *, #253484, .T. ) ;
#39902=ORIENTED_EDGE ( 'NONE', *, *, #149215, .T. ) ;
#39907=CIRCLE ( 'NONE', #139827, 0.1000000000000002554 ) ;
#39979=CARTESIAN_POINT ( 'NONE',  ( 23.40000000000005187, 76.00000000001119815, -36.02310748452479316 ) ) ;
#40027=DIRECTION ( 'NONE',  ( 0.000000000000000000, 0.1332476588733589318, -0.9910827722268049644 ) ) ;
#40031=ORIENTED_EDGE ( 'NONE', *, *, #152151, .T. ) ;
#40053=AXIS2_PLACEMENT_3D ( 'NONE', #132468, #149485, #33403 ) ;
#40076=EDGE_CURVE ( 'NONE', #187747, #165490, #215659, .T. ) ;
#40090=LINE ( 'NONE', #180860, #163421 ) ;
#40093=FACE_OUTER_BOUND ( 'NONE', #185412, .T. ) ;
#40105=LINE ( 'NONE', #43918, #53051 ) ;
#40109=DIRECTION ( 'NONE',  ( 1.000000000000000000, 0.000000000000000000, 0.000000000000000000 ) ) ;
#40114=CARTESIAN_POINT ( 'NONE',  ( 21.05000000000005400, 66.15000000001120384, -4.523107484524794053 ) ) ;
#40157=VERTEX_POINT ( 'NONE', #201094 ) ;
#40167=ORIENTED_EDGE ( 'NONE', *, *, #233329, .F. ) ;
#40218=DIRECTION ( 'NONE',  ( -1.000000000000000000, 0.000000000000000000, 0.000000000000000000 ) ) ;
#40228=EDGE_CURVE ( 'NONE', #187434, #112788, #44990, .T. ) ;
#40315=DIRECTION ( 'NONE',  ( 0.000000000000000000, 0.000000000000000000, -1.000000000000000000 ) ) ;
#40325=CIRCLE ( 'NONE', #223422, 0.1999999999999987899 ) ;
#40337=DIRECTION ( 'NONE',  ( 0.000000000000000000, 0.000000000000000000, -1.000000000000000000 ) ) ;
#40365=SPHERICAL_SURFACE ( 'NONE', #129462, 0.1000000000000000056 ) ;
#40389=DIRECTION ( 'NONE',  ( 3.469446951953620500E-14, 0.000000000000000000, 1.000000000000000000 ) ) ;
#40421=DIRECTION ( 'NONE',  ( 0.000000000000000000, 0.000000000000000000, -1.000000000000000000 ) ) ;
#40439=CARTESIAN_POINT ( 'NONE',  ( -13.39999999999994529, 67.75000000001118394, -18.42310748452479174 ) ) ;
#40458=EDGE_CURVE ( 'NONE', #194487, #45940, #199304, .T. ) ;
#40474=ORIENTED_EDGE ( 'NONE', *, *, #197713, .T. ) ;
#40531=DIRECTION ( 'NONE',  ( 0.000000000000000000, -0.1332476588733589040, -0.9910827722268049644 ) ) ;
#40544=EDGE_CURVE ( 'NONE', #23353, #238821, #36836, .T. ) ;
#40549=EDGE_CURVE ( 'NONE', #136469, #118259, #215836, .T. ) ;
#40555=DIRECTION ( 'NONE',  ( 0.000000000000000000, 0.000000000000000000, 1.000000000000000000 ) ) ;
#40557=VERTEX_POINT ( 'NONE', #97803 ) ;
#40584=ORIENTED_EDGE ( 'NONE', *, *, #60970, .T. ) ;
#40589=ORIENTED_EDGE ( 'NONE', *, *, #212153, .T. ) ;
#40612=ORIENTED_EDGE ( 'NONE', *, *, #12239, .T. ) ;
#40617=ORIENTED_EDGE ( 'NONE', *, *, #61009, .F. ) ;
#40643=AXIS2_PLACEMENT_3D ( 'NONE', #222337, #42444, #25471 ) ;
#40695=VECTOR ( 'NONE', #67076, 1000.000000000000114 ) ;
#40761=ORIENTED_EDGE ( 'NONE', *, *, #159184, .F. ) ;
#40765=EDGE_LOOP ( 'NONE', ( #174649, #139018, #130584, #202846 ) ) ;
#40795=AXIS2_PLACEMENT_3D ( 'NONE', #210736, #227718, #67375 ) ;
#40829=AXIS2_PLACEMENT_3D ( 'NONE', #73664, #208030, #13662 ) ;
#40901=VERTEX_POINT ( 'NONE', #233213 ) ;
#40979=VERTEX_POINT ( 'NONE', #119670 ) ;
#41022=CARTESIAN_POINT ( 'NONE',  ( 0.9000000000000547562, 64.35000000001120668, -12.72310748452478890 ) ) ;
#41062=CARTESIAN_POINT ( 'NONE',  ( -21.04999999999994387, 83.80000000001119531, -34.86056257560453986 ) ) ;
#41075=DIRECTION ( 'NONE',  ( -1.000000000000000000, 0.000000000000000000, 0.000000000000000000 ) ) ;
#41109=CARTESIAN_POINT ( 'NONE',  ( 13.40000000000005898, 67.75000000001118394, -21.02310748452479316 ) ) ;
#41167=EDGE_LOOP ( 'NONE', ( #205966, #53786, #24570, #111384 ) ) ;
#41180=DIRECTION ( 'NONE',  ( 0.000000000000000000, -0.000000000000000000, 1.000000000000000000 ) ) ;
#41224=VECTOR ( 'NONE', #14882, 1000.000000000000114 ) ;
#41280=ORIENTED_EDGE ( 'NONE', *, *, #148987, .T. ) ;
#41318=CARTESIAN_POINT ( 'NONE',  ( -21.04999999999994387, 65.15000000001120384, -4.423107484524790856 ) ) ;
#41331=CARTESIAN_POINT ( 'NONE',  ( 21.15000000000005542, 74.16448838626247664, -47.52760213295649550 ) ) ;
#41333=DIRECTION ( 'NONE',  ( -0.000000000000000000, 0.9910827722268039652, 0.1332476588733670919 ) ) ;
#41366=CIRCLE ( 'NONE', #49714, 0.1000000000000028644 ) ;
#41417=CYLINDRICAL_SURFACE ( 'NONE', #183518, 0.1000000000000028644 ) ;
#41465=CIRCLE ( 'NONE', #203941, 0.1000000000000028644 ) ;
#41478=ORIENTED_EDGE ( 'NONE', *, *, #192409, .T. ) ;
#41493=DIRECTION ( 'NONE',  ( -4.336808689942017736E-16, 0.000000000000000000, -1.000000000000000000 ) ) ;
#41539=AXIS2_PLACEMENT_3D ( 'NONE', #33759, #192793, #213623 ) ;
#41572=ORIENTED_EDGE ( 'NONE', *, *, #40544, .T. ) ;
#41575=DIRECTION ( 'NONE',  ( 1.000000000000000000, 0.000000000000000000, 0.000000000000000000 ) ) ;
#41671=DIRECTION ( 'NONE',  ( 0.000000000000000000, 0.000000000000000000, 1.000000000000000000 ) ) ;
#41843=DIRECTION ( 'NONE',  ( -0.000000000000000000, 1.000000000000000000, -0.000000000000000000 ) ) ;
#41849=VERTEX_POINT ( 'NONE', #135395 ) ;
#41876=EDGE_CURVE ( 'NONE', #114288, #33031, #245819, .T. ) ;
#41877=ORIENTED_EDGE ( 'NONE', *, *, #88840, .T. ) ;
#41928=CARTESIAN_POINT ( 'NONE',  ( 13.40000000000005898, 64.35000000001120668, -23.62310748452479103 ) ) ;
#42084=AXIS2_PLACEMENT_3D ( 'NONE', #117002, #98672, #223785 ) ;
#42097=EDGE_CURVE ( 'NONE', #243775, #22457, #79040, .T. ) ;
#42109=ORIENTED_EDGE ( 'NONE', *, *, #228921, .T. ) ;
#42164=CYLINDRICAL_SURFACE ( 'NONE', #59094, 0.09999999999999982514 ) ;
#42219=DIRECTION ( 'NONE',  ( 1.000000000000000000, 0.000000000000000000, 0.000000000000000000 ) ) ;
#42241=EDGE_CURVE ( 'NONE', #194487, #175937, #150606, .T. ) ;
#42311=VERTEX_POINT ( 'NONE', #219232 ) ;
#42370=ORIENTED_EDGE ( 'NONE', *, *, #25012, .T. ) ;
#42443=ORIENTED_EDGE ( 'NONE', *, *, #170169, .T. ) ;
#42444=DIRECTION ( 'NONE',  ( -0.000000000000000000, 0.000000000000000000, -1.000000000000000000 ) ) ;
#42522=EDGE_CURVE ( 'NONE', #204034, #131851, #203537, .T. ) ;
#42541=CARTESIAN_POINT ( 'NONE',  ( 21.05000000000005400, 82.74366731733570646, -26.36310895752070138 ) ) ;
#42569=EDGE_LOOP ( 'NONE', ( #88999, #189318, #54057 ) ) ;
#42645=CARTESIAN_POINT ( 'NONE',  ( -0.8999999999999437339, 67.75000000001118394, -12.62310748452478926 ) ) ;
#42662=ADVANCED_FACE ( 'NONE', ( #258012 ), #194272, .F. ) ;
#42705=ORIENTED_EDGE ( 'NONE', *, *, #48637, .T. ) ;
#42713=FACE_OUTER_BOUND ( 'NONE', #35896, .T. ) ;
#42716=DIRECTION ( 'NONE',  ( 0.000000000000000000, 0.000000000000000000, 1.000000000000000000 ) ) ;
#42721=CARTESIAN_POINT ( 'NONE',  ( 21.05000000000005400, 87.50449464844290048, -34.18759587077607165 ) ) ;
#42740=ORIENTED_EDGE ( 'NONE', *, *, #107579, .T. ) ;
#42769=CARTESIAN_POINT ( 'NONE',  ( -21.14999999999994174, 83.90000000001120384, -37.18565239344504647 ) ) ;
#42781=CARTESIAN_POINT ( 'NONE',  ( -11.59999999999994458, 64.35000000001120668, -21.02310748452479316 ) ) ;
#42792=CIRCLE ( 'NONE', #9468, 0.09999999999999982514 ) ;
#42795=FACE_OUTER_BOUND ( 'NONE', #148304, .T. ) ;
#42886=EDGE_CURVE ( 'NONE', #38614, #230960, #12755, .T. ) ;
#42922=ADVANCED_FACE ( 'NONE', ( #109247 ), #169276, .T. ) ;
#42956=DIRECTION ( 'NONE',  ( 1.000000000000000000, 0.000000000000000000, 0.000000000000000000 ) ) ;
#42974=EDGE_CURVE ( 'NONE', #64265, #132923, #31047, .T. ) ;
#42988=VECTOR ( 'NONE', #93398, 1000.000000000000000 ) ;
#43003=DIRECTION ( 'NONE',  ( 1.000000000000000000, 0.000000000000000000, 0.000000000000000000 ) ) ;
#43072=ORIENTED_EDGE ( 'NONE', *, *, #190528, .F. ) ;
#43081=AXIS2_PLACEMENT_3D ( 'NONE', #95227, #90073, #15726 ) ;
#43110=DIRECTION ( 'NONE',  ( 0.000000000000000000, 0.000000000000000000, -1.000000000000000000 ) ) ;
#43141=AXIS2_PLACEMENT_3D ( 'NONE', #213854, #35250, #194320 ) ;
#43144=ORIENTED_EDGE ( 'NONE', *, *, #38311, .F. ) ;
#43170=AXIS2_PLACEMENT_3D ( 'NONE', #174226, #116772, #175487 ) ;
#43277=CYLINDRICAL_SURFACE ( 'NONE', #136716, 0.1000000000000028644 ) ;
#43322=LINE ( 'NONE', #117709, #165597 ) ;
#43334=VECTOR ( 'NONE', #44078, 1000.000000000000000 ) ;
#43368=CARTESIAN_POINT ( 'NONE',  ( 23.40000000000005187, 79.78873604695631627, -7.297728304630792806 ) ) ;
#43372=ORIENTED_EDGE ( 'NONE', *, *, #60513, .F. ) ;
#43374=VERTEX_POINT ( 'NONE', #148084 ) ;
#43427=CARTESIAN_POINT ( 'NONE',  ( -5.899999999999938183, 64.35000000001120668, -26.02310748452479316 ) ) ;
#43457=EDGE_CURVE ( 'NONE', #170630, #251948, #241704, .T. ) ;
#43553=LINE ( 'NONE', #24002, #125084 ) ;
#43618=TOROIDAL_SURFACE ( 'NONE', #51969, 0.2000000000000000111, 0.1000000000000000056 ) ;
#43644=CARTESIAN_POINT ( 'NONE',  ( 20.95000000000005258, 64.35000000001119247, -5.923107484524795296 ) ) ;
#43675=ORIENTED_EDGE ( 'NONE', *, *, #190528, .T. ) ;
#43696=DIRECTION ( 'NONE',  ( -0.000000000000000000, -0.9910827722268042983, 0.1332476588733650935 ) ) ;
#43731=CARTESIAN_POINT ( 'NONE',  ( -21.14999999999994174, 77.16254490893143725, -43.92310748452479885 ) ) ;
#43739=ORIENTED_EDGE ( 'NONE', *, *, #172205, .T. ) ;
#43754=STYLED_ITEM ( 'NONE', ( #108588 ), #200717 ) ;
#43847=CARTESIAN_POINT ( 'NONE',  ( -0.8999999999999437339, 67.75000000001118394, -10.02310748452479139 ) ) ;
#43856=VECTOR ( 'NONE', #91606, 1000.000000000000000 ) ;
#43914=ORIENTED_EDGE ( 'NONE', *, *, #234616, .F. ) ;
#43918=CARTESIAN_POINT ( 'NONE',  ( -23.49999999999994316, 77.83551161375991967, -47.62760213295649692 ) ) ;
#44029=EDGE_CURVE ( 'NONE', #109797, #182432, #187742, .T. ) ;
#44044=DIRECTION ( 'NONE',  ( 1.000000000000000000, -0.000000000000000000, 0.000000000000000000 ) ) ;
#44045=VERTEX_POINT ( 'NONE', #171883 ) ;
#44067=CARTESIAN_POINT ( 'NONE',  ( -20.94999999999994600, 66.25000000001119815, -4.623107484524796362 ) ) ;
#44078=DIRECTION ( 'NONE',  ( 1.000000000000000000, 0.000000000000000000, 0.000000000000000000 ) ) ;
#44106=EDGE_CURVE ( 'NONE', #56611, #44045, #186612, .T. ) ;
#44112=CYLINDRICAL_SURFACE ( 'NONE', #38613, 0.09999999999999530098 ) ;
#44127=DIRECTION ( 'NONE',  ( 0.000000000000000000, 0.000000000000000000, 1.000000000000000000 ) ) ;
#44141=CARTESIAN_POINT ( 'NONE',  ( -11.59999999999994458, 67.75000000001118394, -21.02310748452479316 ) ) ;
#44228=ORIENTED_EDGE ( 'NONE', *, *, #253920, .T. ) ;
#44230=CIRCLE ( 'NONE', #215089, 4.041421356237314022 ) ;
#44254=ORIENTED_EDGE ( 'NONE', *, *, #200564, .F. ) ;
#44256=ORIENTED_EDGE ( 'NONE', *, *, #169123, .T. ) ;
#44264=CARTESIAN_POINT ( 'NONE',  ( -23.39999999999994529, 77.25000000001119815, -43.82310748452479743 ) ) ;
#44290=EDGE_CURVE ( 'NONE', #250175, #121523, #101234, .T. ) ;
#44312=DIRECTION ( 'NONE',  ( 0.000000000000000000, 0.000000000000000000, -1.000000000000000000 ) ) ;
#44338=FILL_AREA_STYLE_COLOUR ( '', #69842 ) ;
#44352=DIRECTION ( 'NONE',  ( -1.000000000000000000, 0.000000000000000000, 0.000000000000000000 ) ) ;
#44384=ORIENTED_EDGE ( 'NONE', *, *, #158548, .F. ) ;
#44423=CARTESIAN_POINT ( 'NONE',  ( 6.100000000000061817, 64.35000000001120668, -22.12310748452479103 ) ) ;
#44506=AXIS2_PLACEMENT_3D ( 'NONE', #67834, #88657, #187801 ) ;
#44509=AXIS2_PLACEMENT_3D ( 'NONE', #216327, #115966, #96366 ) ;
#44522=DIRECTION ( 'NONE',  ( 1.000000000000000000, 0.000000000000000000, 0.000000000000000000 ) ) ;
#44581=AXIS2_PLACEMENT_3D ( 'NONE', #149943, #131637, #52083 ) ;
#44616=LINE ( 'NONE', #8064, #114164 ) ;
#44639=VECTOR ( 'NONE', #234147, 1000.000000000000000 ) ;
#44640=ADVANCED_FACE ( 'NONE', ( #198791 ), #158424, .T. ) ;
#44662=ADVANCED_FACE ( 'NONE', ( #203933 ), #80092, .T. ) ;
#44697=ORIENTED_EDGE ( 'NONE', *, *, #40076, .T. ) ;
#44728=FACE_OUTER_BOUND ( 'NONE', #89809, .T. ) ;
#44746=CARTESIAN_POINT ( 'NONE',  ( -20.94999999999994600, 65.25000000001119815, -3.123107484524795474 ) ) ;
#44766=( LENGTH_UNIT ( ) NAMED_UNIT ( * ) SI_UNIT ( .MILLI., .METRE. ) );
#44774=CARTESIAN_POINT ( 'NONE',  ( 21.15000000000005187, 76.00000000001119815, -36.02310748452479316 ) ) ;
#44789=CYLINDRICAL_SURFACE ( 'NONE', #78760, 0.09999999999999939493 ) ;
#44813=LINE ( 'NONE', #64379, #203496 ) ;
#44892=DIRECTION ( 'NONE',  ( 0.000000000000000000, -0.000000000000000000, -1.000000000000000000 ) ) ;
#44899=ORIENTED_EDGE ( 'NONE', *, *, #29093, .T. ) ;
#44929=DIRECTION ( 'NONE',  ( -0.000000000000000000, 1.000000000000000000, -0.000000000000000000 ) ) ;
#44933=AXIS2_PLACEMENT_3D ( 'NONE', #251341, #113129, #72752 ) ;
#44961=EDGE_CURVE ( 'NONE', #42311, #75854, #34318, .T. ) ;
#44990=CIRCLE ( 'NONE', #78292, 4.150000000000001243 ) ;
#45001=DIRECTION ( 'NONE',  ( -1.000000000000000000, 0.000000000000000000, 0.000000000000000000 ) ) ;
#45025=CARTESIAN_POINT ( 'NONE',  ( -13.39999999999994529, 67.72071067812984779, -17.05239680640613642 ) ) ;
#45094=DIRECTION ( 'NONE',  ( 1.000000000000000000, -0.000000000000000000, 0.000000000000000000 ) ) ;
#45128=FACE_OUTER_BOUND ( 'NONE', #129484, .T. ) ;
#45146=CARTESIAN_POINT ( 'NONE',  ( -23.49999999999994316, 74.25000000001119815, -47.64205752314703801 ) ) ;
#45154=CIRCLE ( 'NONE', #49249, 0.1000000000000028644 ) ;
#45216=VERTEX_POINT ( 'NONE', #96358 ) ;
#45270=ADVANCED_FACE ( 'NONE', ( #198037 ), #44112, .T. ) ;
#45330=CIRCLE ( 'NONE', #49434, 0.09999999999999939493 ) ;
#45354=DIRECTION ( 'NONE',  ( 0.000000000000000000, 0.9910827722268055195, 0.1332476588733540468 ) ) ;
#45370=DIRECTION ( 'NONE',  ( 0.000000000000000000, 0.000000000000000000, -1.000000000000000000 ) ) ;
#45396=ORIENTED_EDGE ( 'NONE', *, *, #33176, .F. ) ;
#45402=AXIS2_PLACEMENT_3D ( 'NONE', #10915, #74768, #55128 ) ;
#45417=ORIENTED_EDGE ( 'NONE', *, *, #205499, .T. ) ;
#45442=ORIENTED_EDGE ( 'NONE', *, *, #55748, .F. ) ;
#45451=ORIENTED_EDGE ( 'NONE', *, *, #246410, .T. ) ;
#45480=AXIS2_PLACEMENT_3D ( 'NONE', #74572, #160513, #37998 ) ;
#45485=DIRECTION ( 'NONE',  ( 0.000000000000000000, 0.000000000000000000, 1.000000000000000000 ) ) ;
#45498=FACE_OUTER_BOUND ( 'NONE', #17919, .T. ) ;
#45514=CARTESIAN_POINT ( 'NONE',  ( -13.39999999999994529, 67.75000000001118394, -23.62310748452479103 ) ) ;
#45566=EDGE_LOOP ( 'NONE', ( #12679, #101942, #7879, #60698 ) ) ;
#45594=CIRCLE ( 'NONE', #83136, 0.1999999999999987899 ) ;
#45615=SURFACE_STYLE_USAGE ( .BOTH. , #78299 ) ;
#45667=EDGE_CURVE ( 'NONE', #144818, #40557, #11178, .T. ) ;
#45681=AXIS2_PLACEMENT_3D ( 'NONE', #68672, #209453, #13830 ) ;
#45718=LINE ( 'NONE', #9165, #118910 ) ;
#45757=DIRECTION ( 'NONE',  ( 1.000000000000000000, 0.000000000000000000, 0.000000000000000000 ) ) ;
#45767=DIRECTION ( 'NONE',  ( 1.000000000000000000, 0.000000000000000000, 0.000000000000000000 ) ) ;
#45779=LINE ( 'NONE', #146157, #195896 ) ;
#45799=EDGE_CURVE ( 'NONE', #190938, #119358, #192929, .T. ) ;
#45866=LINE ( 'NONE', #181550, #24777 ) ;
#45898=AXIS2_PLACEMENT_3D ( 'NONE', #192712, #36221, #115736 ) ;
#45940=VERTEX_POINT ( 'NONE', #239205 ) ;
#45972=ORIENTED_EDGE ( 'NONE', *, *, #253358, .T. ) ;
#45989=ORIENTED_EDGE ( 'NONE', *, *, #163051, .T. ) ;
#46019=CARTESIAN_POINT ( 'NONE',  ( 0.9000000000000547562, 67.72071067812984779, -10.02310748452479139 ) ) ;
#46036=SURFACE_STYLE_USAGE ( .BOTH. , #49893 ) ;
#46143=DIRECTION ( 'NONE',  ( 0.000000000000000000, -0.5774316882803290918, -0.8164390028469542537 ) ) ;
#46198=LINE ( 'NONE', #108748, #92484 ) ;
#46237=VECTOR ( 'NONE', #11253, 1000.000000000000000 ) ;
#46282=SPHERICAL_SURFACE ( 'NONE', #38832, 0.1000000000000000056 ) ;
#46289=DIRECTION ( 'NONE',  ( -0.000000000000000000, -0.000000000000000000, 1.000000000000000000 ) ) ;
#46299=AXIS2_PLACEMENT_3D ( 'NONE', #254058, #75466, #154999 ) ;
#46347=CARTESIAN_POINT ( 'NONE',  ( -21.14999999999994174, 74.26359666348515987, -47.54092689884382850 ) ) ;
#46428=ADVANCED_FACE ( 'NONE', ( #218683 ), #26713, .T. ) ;
#46485=DIRECTION ( 'NONE',  ( 1.000000000000000000, 0.000000000000000000, 0.000000000000000000 ) ) ;
#46490=VERTEX_POINT ( 'NONE', #96171 ) ;
#46513=LINE ( 'NONE', #205588, #13756 ) ;
#46617=DIRECTION ( 'NONE',  ( 0.000000000000000000, -1.000000000000000000, 0.000000000000000000 ) ) ;
#46632=AXIS2_PLACEMENT_3D ( 'NONE', #106866, #52018, #92433 ) ;
#46652=DIRECTION ( 'NONE',  ( -0.000000000000000000, 1.000000000000000000, -0.000000000000000000 ) ) ;
#46717=DIRECTION ( 'NONE',  ( -0.000000000000000000, 1.000000000000000000, -0.000000000000000000 ) ) ;
#46738=EDGE_CURVE ( 'NONE', #230960, #66524, #51217, .T. ) ;
#46740=AXIS2_PLACEMENT_3D ( 'NONE', #100939, #181818, #81392 ) ;
#46751=FACE_OUTER_BOUND ( 'NONE', #238283, .T. ) ;
#46767=CYLINDRICAL_SURFACE ( 'NONE', #113843, 0.09999999999999982514 ) ;
#46770=ORIENTED_EDGE ( 'NONE', *, *, #38189, .F. ) ;
#46777=DIRECTION ( 'NONE',  ( 0.000000000000000000, -1.000000000000000000, 0.000000000000000000 ) ) ;
#46788=LINE ( 'NONE', #126339, #23080 ) ;
#46862=CARTESIAN_POINT ( 'NONE',  ( 23.40000000000005542, 83.98667523412385094, -37.28476067066772970 ) ) ;
#46895=CARTESIAN_POINT ( 'NONE',  ( -20.94999999999994600, 64.25000000001119815, -5.923107484524795296 ) ) ;
#46905=CARTESIAN_POINT ( 'NONE',  ( 23.40000000000005542, 76.00000000001119815, -3.023107484524792277 ) ) ;
#46908=AXIS2_PLACEMENT_3D ( 'NONE', #151717, #172583, #9589 ) ;
#46913=PLANE ( 'NONE',  #221818 ) ;
#46943=CIRCLE ( 'NONE', #126051, 0.1000000000000028644 ) ;
#46970=DIRECTION ( 'NONE',  ( 0.000000000000000000, -1.156482317317873105E-15, -1.000000000000000000 ) ) ;
#47032=CARTESIAN_POINT ( 'NONE',  ( -0.8999999999999437339, 64.35000000001120668, -7.423107484524793520 ) ) ;
#47038=ORIENTED_EDGE ( 'NONE', *, *, #149215, .F. ) ;
#47041=CIRCLE ( 'NONE', #105270, 0.1000000000000032391 ) ;
#47048=EDGE_CURVE ( 'NONE', #50040, #40157, #51391, .T. ) ;
#47100=CARTESIAN_POINT ( 'NONE',  ( 21.15000000000005187, 74.94272479589878344, -8.023107484524793165 ) ) ;
#47103=FACE_OUTER_BOUND ( 'NONE', #161036, .T. ) ;
#47124=DIRECTION ( 'NONE',  ( -1.000000000000000000, 0.000000000000000000, 0.000000000000000000 ) ) ;
#47160=DIRECTION ( 'NONE',  ( 1.000000000000000000, -0.000000000000000000, -0.000000000000000000 ) ) ;
#47174=DIRECTION ( 'NONE',  ( 0.000000000000000000, 0.000000000000000000, 1.000000000000000000 ) ) ;
#47182=PLANE ( 'NONE',  #70475 ) ;
#47189=AXIS2_PLACEMENT_3D ( 'NONE', #124247, #126799, #165953 ) ;
#47207=CARTESIAN_POINT ( 'NONE',  ( 23.50000000000005684, 76.00000000001119815, -36.02310748452479316 ) ) ;
#47221=ORIENTED_EDGE ( 'NONE', *, *, #84259, .F. ) ;
#47251=ORIENTED_EDGE ( 'NONE', *, *, #39273, .T. ) ;
#47396=LINE ( 'NONE', #126952, #165446 ) ;
#47407=DIRECTION ( 'NONE',  ( 0.000000000000000000, 0.000000000000000000, 1.000000000000000000 ) ) ;
#47424=EDGE_CURVE ( 'NONE', #144016, #113568, #11916, .T. ) ;
#47458=CARTESIAN_POINT ( 'NONE',  ( -23.39999999999994529, 64.25000000001119815, -3.123107484524795474 ) ) ;
#47469=ADVANCED_FACE ( 'NONE', ( #70614 ), #9319, .T. ) ;
#47517=LINE ( 'NONE', #86632, #59659 ) ;
#47593=DIRECTION ( 'NONE',  ( -0.000000000000000000, 0.000000000000000000, -1.000000000000000000 ) ) ;
#47691=EDGE_LOOP ( 'NONE', ( #237598, #230914, #76016, #64885 ) ) ;
#47747=CARTESIAN_POINT ( 'NONE',  ( -5.899999999999938183, 64.65000000001120384, -22.12310748452479103 ) ) ;
#47887=ORIENTED_EDGE ( 'NONE', *, *, #148497, .F. ) ;
#47892=ADVANCED_FACE ( 'NONE', ( #58050 ), #205911, .T. ) ;
#47923=AXIS2_PLACEMENT_3D ( 'NONE', #103436, #108597, #9491 ) ;
#47930=EDGE_LOOP ( 'NONE', ( #182577, #20003, #215934, #249879 ) ) ;
#47931=EDGE_LOOP ( 'NONE', ( #181341, #134228, #163971, #216047 ) ) ;
#47953=CYLINDRICAL_SURFACE ( 'NONE', #123787, 0.1000000000000021844 ) ;
#47957=VECTOR ( 'NONE', #101118, 1000.000000000000000 ) ;
#47991=DIRECTION ( 'NONE',  ( 0.000000000000000000, -0.1332476588733589040, -0.9910827722268048534 ) ) ;
#48006=CARTESIAN_POINT ( 'NONE',  ( -21.04999999999994387, 65.36599112033563586, -30.02023607076051803 ) ) ;
#48011=CARTESIAN_POINT ( 'NONE',  ( -23.49999999999994316, 84.00000000001119815, -37.18565239344504647 ) ) ;
#48023=ADVANCED_FACE ( 'NONE', ( #35960 ), #24114, .F. ) ;
#48046=DIRECTION ( 'NONE',  ( 3.469446951953515108E-14, -1.000000000000000000, 0.000000000000000000 ) ) ;
#48164=VECTOR ( 'NONE', #74660, 1000.000000000000000 ) ;
#48186=EDGE_LOOP ( 'NONE', ( #209623, #250278, #238000, #8676 ) ) ;
#48198=CYLINDRICAL_SURFACE ( 'NONE', #168511, 0.09999999999999939493 ) ;
#48202=ADVANCED_FACE ( 'NONE', ( #53925 ), #56238, .F. ) ;
#48210=ORIENTED_EDGE ( 'NONE', *, *, #68832, .T. ) ;
#48301=ORIENTED_EDGE ( 'NONE', *, *, #117874, .F. ) ;
#48303=EDGE_LOOP ( 'NONE', ( #45417, #8251, #29288, #130669 ) ) ;
#48419=AXIS2_PLACEMENT_3D ( 'NONE', #196627, #74163, #156262 ) ;
#48444=ORIENTED_EDGE ( 'NONE', *, *, #81722, .T. ) ;
#48449=CIRCLE ( 'NONE', #152537, 0.1999999999999987899 ) ;
#48494=ORIENTED_EDGE ( 'NONE', *, *, #72723, .F. ) ;
#48543=ORIENTED_EDGE ( 'NONE', *, *, #129131, .F. ) ;
#48545=ORIENTED_EDGE ( 'NONE', *, *, #214901, .T. ) ;
#48561=ORIENTED_EDGE ( 'NONE', *, *, #122571, .T. ) ;
#48595=CARTESIAN_POINT ( 'NONE',  ( 23.40000000000005542, 74.73834681386826162, -44.00978271863746016 ) ) ;
#48615=DIRECTION ( 'NONE',  ( 0.000000000000000000, 0.000000000000000000, 1.000000000000000000 ) ) ;
#48637=EDGE_CURVE ( 'NONE', #167224, #228476, #90210, .T. ) ;
#48660=ORIENTED_EDGE ( 'NONE', *, *, #165404, .F. ) ;
#48739=ORIENTED_EDGE ( 'NONE', *, *, #28595, .F. ) ;
#48750=CIRCLE ( 'NONE', #186122, 0.09999999999999939493 ) ;
#48775=AXIS2_PLACEMENT_3D ( 'NONE', #196878, #114783, #212611 ) ;
#48777=EDGE_LOOP ( 'NONE', ( #209965, #242755, #169860, #186120 ) ) ;
#48790=DIRECTION ( 'NONE',  ( -1.000000000000000000, 0.000000000000000000, 0.000000000000000000 ) ) ;
#48805=CARTESIAN_POINT ( 'NONE',  ( -23.49999999999994316, 79.88763423575340994, -7.282924647898262549 ) ) ;
#48843=EDGE_CURVE ( 'NONE', #97363, #211140, #148506, .T. ) ;
#48860=ORIENTED_EDGE ( 'NONE', *, *, #46738, .F. ) ;
#48940=DIRECTION ( 'NONE',  ( 1.000000000000000000, -0.000000000000000000, -0.000000000000000000 ) ) ;
#48950=VECTOR ( 'NONE', #11539, 1000.000000000000114 ) ;
#48989=CARTESIAN_POINT ( 'NONE',  ( -21.04999999999994387, 77.16254490893143725, -43.82310748452479743 ) ) ;
#49063=LINE ( 'NONE', #138839, #17117 ) ;
#49104=DIRECTION ( 'NONE',  ( -0.000000000000000000, 1.000000000000000000, 0.000000000000000000 ) ) ;
#49150=CIRCLE ( 'NONE', #19951, 0.1000000000000028644 ) ;
#49165=EDGE_LOOP ( 'NONE', ( #229805, #15581, #43372, #82638 ) ) ;
#49193=VERTEX_POINT ( 'NONE', #51234 ) ;
#49249=AXIS2_PLACEMENT_3D ( 'NONE', #72437, #33334, #11165 ) ;
#49258=EDGE_LOOP ( 'NONE', ( #107562, #185036, #152079, #224520, #135766, #42370, #51250, #186445, #182657, #166634, #154376, #190901, #247545, #15387, #151696, #185396, #227966, #181924 ) ) ;
#49265=ORIENTED_EDGE ( 'NONE', *, *, #38189, .T. ) ;
#49272=EDGE_CURVE ( 'NONE', #10605, #123853, #47396, .T. ) ;
#49277=DIRECTION ( 'NONE',  ( 0.000000000000000000, -1.000000000000000000, 0.000000000000000000 ) ) ;
#49311=DIRECTION ( 'NONE',  ( 0.000000000000000000, -1.000000000000000000, 0.000000000000000000 ) ) ;
#49434=AXIS2_PLACEMENT_3D ( 'NONE', #93946, #76948, #156534 ) ;
#49464=DIRECTION ( 'NONE',  ( 0.000000000000000000, 0.9889818879709272315, 0.1480365673253073999 ) ) ;
#49478=ADVANCED_FACE ( 'NONE', ( #240186 ), #170176, .T. ) ;
#49531=CARTESIAN_POINT ( 'NONE',  ( -23.49999999999994316, 77.25000000001119815, -43.92310748452479885 ) ) ;
#49559=FACE_OUTER_BOUND ( 'NONE', #156576, .T. ) ;
#49678=DIRECTION ( 'NONE',  ( 0.000000000000000000, 0.1332476588733589318, 0.9910827722268049644 ) ) ;
#49708=DIRECTION ( 'NONE',  ( 1.000000000000000000, 0.000000000000000000, 0.000000000000000000 ) ) ;
#49714=AXIS2_PLACEMENT_3D ( 'NONE', #246175, #147051, #240082 ) ;
#49769=CARTESIAN_POINT ( 'NONE',  ( -23.39999999999994529, 76.00000000001119815, -36.02310748452479316 ) ) ;
#49772=DIRECTION ( 'NONE',  ( -1.000000000000000000, 0.000000000000000000, 4.336808689942017736E-16 ) ) ;
#49799=EDGE_CURVE ( 'NONE', #3259, #176509, #199568, .T. ) ;
#49804=ORIENTED_EDGE ( 'NONE', *, *, #235973, .T. ) ;
#49817=EDGE_LOOP ( 'NONE', ( #41478, #96927, #106977, #140142 ) ) ;
#49833=ORIENTED_EDGE ( 'NONE', *, *, #60513, .T. ) ;
#49893=SURFACE_SIDE_STYLE ('',( #245541 ) ) ;
#49908=CARTESIAN_POINT ( 'NONE',  ( 23.40000000000005542, 64.35000000001120668, -3.123107484524795474 ) ) ;
#49977=TOROIDAL_SURFACE ( 'NONE', #20978, 11.65000000000000036, 0.1000000000000000056 ) ;
#50040=VERTEX_POINT ( 'NONE', #209732 ) ;
#50075=DIRECTION ( 'NONE',  ( -1.000000000000000000, -0.000000000000000000, -0.000000000000000000 ) ) ;
#50086=DIRECTION ( 'NONE',  ( 1.000000000000000000, -0.000000000000000000, -0.000000000000000000 ) ) ;
#50107=AXIS2_PLACEMENT_3D ( 'NONE', #105962, #186827, #8187 ) ;
#50152=EDGE_LOOP ( 'NONE', ( #34097, #130540, #187396, #181433 ) ) ;
#50165=EDGE_CURVE ( 'NONE', #210784, #9389, #97447, .T. ) ;
#50217=FACE_OUTER_BOUND ( 'NONE', #242898, .T. ) ;
#50238=DIRECTION ( 'NONE',  ( 0.000000000000000000, 0.000000000000000000, 1.000000000000000000 ) ) ;
#50271=ORIENTED_EDGE ( 'NONE', *, *, #53881, .F. ) ;
#50284=ORIENTED_EDGE ( 'NONE', *, *, #215019, .T. ) ;
#50293=VECTOR ( 'NONE', #124961, 1000.000000000000000 ) ;
#50297=CIRCLE ( 'NONE', #108578, 0.1000000000000002554 ) ;
#50299=EDGE_CURVE ( 'NONE', #80879, #68170, #243401, .T. ) ;
#50347=VERTEX_POINT ( 'NONE', #188564 ) ;
#50354=VECTOR ( 'NONE', #98668, 1000.000000000000000 ) ;
#50389=FACE_OUTER_BOUND ( 'NONE', #64470, .T. ) ;
#50391=CIRCLE ( 'NONE', #216999, 11.75000000000000000 ) ;
#50417=CARTESIAN_POINT ( 'NONE',  ( -21.14999999999994174, 83.80000000001119531, -37.18565239344504647 ) ) ;
#50428=ORIENTED_EDGE ( 'NONE', *, *, #85563, .F. ) ;
#50498=ORIENTED_EDGE ( 'NONE', *, *, #167446, .F. ) ;
#50499=ADVANCED_FACE ( 'NONE', ( #254898 ), #29069, .T. ) ;
#50508=DIRECTION ( 'NONE',  ( 1.000000000000000000, 0.000000000000000000, 0.000000000000000000 ) ) ;
#50531=ORIENTED_EDGE ( 'NONE', *, *, #138533, .F. ) ;
#50553=AXIS2_PLACEMENT_3D ( 'NONE', #224879, #43696, #223589 ) ;
#50567=DIRECTION ( 'NONE',  ( -1.000000000000000000, 0.000000000000000000, 0.000000000000000000 ) ) ;
#50617=CARTESIAN_POINT ( 'NONE',  ( 11.60000000000006004, 64.35000000001120668, -18.42310748452479530 ) ) ;
#50686=EDGE_CURVE ( 'NONE', #137320, #113073, #33353, .T. ) ;
#50732=ORIENTED_EDGE ( 'NONE', *, *, #125578, .F. ) ;
#50820=ORIENTED_EDGE ( 'NONE', *, *, #67987, .F. ) ;
#50827=VERTEX_POINT ( 'NONE', #182525 ) ;
#50840=CIRCLE ( 'NONE', #242393, 0.1000000000000028644 ) ;
#50878=LINE ( 'NONE', #232129, #212439 ) ;
#50966=PLANE ( 'NONE',  #238727 ) ;
#51042=CIRCLE ( 'NONE', #250965, 2.600000000000000089 ) ;
#51189=ORIENTED_EDGE ( 'NONE', *, *, #253119, .F. ) ;
#51217=CIRCLE ( 'NONE', #118468, 0.1000000000000016709 ) ;
#51218=DIRECTION ( 'NONE',  ( 1.000000000000000000, -0.000000000000000000, -0.000000000000000000 ) ) ;
#51234=CARTESIAN_POINT ( 'NONE',  ( 23.50000000000005684, 64.35000000001120668, -3.123107484524795474 ) ) ;
#51243=DIRECTION ( 'NONE',  ( 0.000000000000000000, -1.000000000000000000, 0.000000000000000000 ) ) ;
#51250=ORIENTED_EDGE ( 'NONE', *, *, #67100, .F. ) ;
#51314=ADVANCED_FACE ( 'NONE', ( #197891 ), #41417, .T. ) ;
#51391=CIRCLE ( 'NONE', #218000, 0.1999999999999987899 ) ;
#51408=ADVANCED_FACE ( 'NONE', ( #208188 ), #225140, .T. ) ;
#51463=CARTESIAN_POINT ( 'NONE',  ( 21.15000000000005187, 87.50449464844290048, -34.18759587077607165 ) ) ;
#51523=AXIS2_PLACEMENT_3D ( 'NONE', #156880, #137272, #18622 ) ;
#51528=EDGE_LOOP ( 'NONE', ( #108943, #48543, #113860 ) ) ;
#51536=ORIENTED_EDGE ( 'NONE', *, *, #257500, .T. ) ;
#51549=EDGE_CURVE ( 'NONE', #128131, #24547, #150217, .T. ) ;
#51585=AXIS2_PLACEMENT_3D ( 'NONE', #156629, #137023, #60039 ) ;
#51599=CARTESIAN_POINT ( 'NONE',  ( 5.900000000000059863, 64.35000000001120668, -26.12310748452479103 ) ) ;
#51638=EDGE_LOOP ( 'NONE', ( #132788, #88966, #254042, #200561 ) ) ;
#51647=CIRCLE ( 'NONE', #18365, 0.1999999999999987899 ) ;
#51657=CARTESIAN_POINT ( 'NONE',  ( -23.39999999999994529, 76.00000000001119815, -31.87310748452479459 ) ) ;
#51697=FACE_OUTER_BOUND ( 'NONE', #132990, .T. ) ;
#51783=FACE_OUTER_BOUND ( 'NONE', #32252, .T. ) ;
#51797=ADVANCED_FACE ( 'NONE', ( #8399 ), #87892, .T. ) ;
#51836=VECTOR ( 'NONE', #81596, 1000.000000000000000 ) ;
#51879=CARTESIAN_POINT ( 'NONE',  ( 21.15000000000005542, 87.50449464844290048, -37.85861909827351468 ) ) ;
#51905=ADVANCED_FACE ( 'NONE', ( #150481 ), #30541, .F. ) ;
#51913=DIRECTION ( 'NONE',  ( 0.000000000000000000, -1.000000000000000000, 0.000000000000000000 ) ) ;
#51918=AXIS2_PLACEMENT_3D ( 'NONE', #241529, #182867, #184111 ) ;
#51962=ORIENTED_EDGE ( 'NONE', *, *, #196634, .F. ) ;
#51969=AXIS2_PLACEMENT_3D ( 'NONE', #110413, #88257, #189961 ) ;
#51970=VECTOR ( 'NONE', #122187, 1000.000000000000000 ) ;
#51994=VERTEX_POINT ( 'NONE', #197290 ) ;
#52005=DIRECTION ( 'NONE',  ( -1.000000000000000000, 0.000000000000000000, 0.000000000000000000 ) ) ;
#52018=DIRECTION ( 'NONE',  ( 1.000000000000000000, 0.000000000000000000, 0.000000000000000000 ) ) ;
#52047=EDGE_CURVE ( 'NONE', #166555, #197879, #250515, .T. ) ;
#52076=ORIENTED_EDGE ( 'NONE', *, *, #204943, .F. ) ;
#52082=LINE ( 'NONE', #211178, #122898 ) ;
#52083=DIRECTION ( 'NONE',  ( 0.000000000000000000, -0.8741572761215442577, 0.4856429311786202851 ) ) ;
#52087=CIRCLE ( 'NONE', #243646, 0.1000000000000002554 ) ;
#52095=EDGE_CURVE ( 'NONE', #160549, #88017, #4782, .T. ) ;
#52205=AXIS2_PLACEMENT_3D ( 'NONE', #216940, #78707, #239093 ) ;
#52211=DIRECTION ( 'NONE',  ( 0.000000000000000000, 1.000000000000000000, 0.000000000000000000 ) ) ;
#52230=VECTOR ( 'NONE', #36774, 1000.000000000000000 ) ;
#52280=DIRECTION ( 'NONE',  ( 0.000000000000000000, 0.000000000000000000, -1.000000000000000000 ) ) ;
#52328=VERTEX_POINT ( 'NONE', #189299 ) ;
#52357=DIRECTION ( 'NONE',  ( 1.284434275755705789E-16, -0.7071067811865472397, 0.7071067811865479058 ) ) ;
#52379=FACE_OUTER_BOUND ( 'NONE', #48303, .T. ) ;
#52429=CARTESIAN_POINT ( 'NONE',  ( 11.60000000000006182, 66.35000000001119247, -23.62310748452479103 ) ) ;
#52432=DIRECTION ( 'NONE',  ( 0.000000000000000000, 0.000000000000000000, 1.000000000000000000 ) ) ;
#52437=ORIENTED_EDGE ( 'NONE', *, *, #209683, .F. ) ;
#52446=ORIENTED_EDGE ( 'NONE', *, *, #110149, .T. ) ;
#52497=FACE_OUTER_BOUND ( 'NONE', #155092, .T. ) ;
#52508=FACE_OUTER_BOUND ( 'NONE', #20815, .T. ) ;
#52514=AXIS2_PLACEMENT_3D ( 'NONE', #60754, #221116, #120774 ) ;
#52515=ORIENTED_EDGE ( 'NONE', *, *, #240703, .T. ) ;
#52526=DIRECTION ( 'NONE',  ( 0.000000000000000000, 0.000000000000000000, -1.000000000000000000 ) ) ;
#52528=ORIENTED_EDGE ( 'NONE', *, *, #251511, .F. ) ;
#52546=CARTESIAN_POINT ( 'NONE',  ( 23.50000000000005684, 73.52684270758111040, -52.27034697567518862 ) ) ;
#52679=CIRCLE ( 'NONE', #94373, 11.65000000000000036 ) ;
#52757=CARTESIAN_POINT ( 'NONE',  ( -23.49999999999994316, 64.35000000001120668, -26.12310748452479103 ) ) ;
#52758=DIRECTION ( 'NONE',  ( 1.000000000000000000, 0.000000000000000000, 0.000000000000000000 ) ) ;
#52769=FACE_OUTER_BOUND ( 'NONE', #79827, .T. ) ;
#52786=PLANE ( 'NONE',  #122786 ) ;
#52854=VECTOR ( 'NONE', #146789, 1000.000000000000000 ) ;
#52892=LINE ( 'NONE', #13774, #181904 ) ;
#52941=CARTESIAN_POINT ( 'NONE',  ( 23.50000000000005684, 87.50449464844290048, -37.85861909827351468 ) ) ;
#52956=DIRECTION ( 'NONE',  ( -0.000000000000000000, -0.000000000000000000, 1.000000000000000000 ) ) ;
#52973=EDGE_CURVE ( 'NONE', #104499, #135971, #86742, .T. ) ;
#52979=CYLINDRICAL_SURFACE ( 'NONE', #152377, 0.09999999999999939493 ) ;
#52987=LINE ( 'NONE', #97207, #42988 ) ;
#53009=CARTESIAN_POINT ( 'NONE',  ( 23.50000000000005684, 83.97335046823651794, -37.38386894789040582 ) ) ;
#53018=ORIENTED_EDGE ( 'NONE', *, *, #199533, .F. ) ;
#53024=VERTEX_POINT ( 'NONE', #250953 ) ;
#53051=VECTOR ( 'NONE', #161318, 1000.000000000000000 ) ;
#53150=CYLINDRICAL_SURFACE ( 'NONE', #44933, 0.09999999999999939493 ) ;
#53175=DIRECTION ( 'NONE',  ( 0.000000000000000000, -0.4856429311786358283, -0.8741572761215357090 ) ) ;
#53254=TOROIDAL_SURFACE ( 'NONE', #178175, 0.2000000000000000111, 0.1000000000000000056 ) ;
#53268=DIRECTION ( 'NONE',  ( -0.000000000000000000, 1.000000000000000000, -0.000000000000000000 ) ) ;
#53279=FACE_OUTER_BOUND ( 'NONE', #36763, .T. ) ;
#53296=EDGE_LOOP ( 'NONE', ( #169110, #40589, #243288, #225183 ) ) ;
#53393=FACE_OUTER_BOUND ( 'NONE', #189612, .T. ) ;
#53455=ORIENTED_EDGE ( 'NONE', *, *, #208102, .T. ) ;
#53534=AXIS2_PLACEMENT_3D ( 'NONE', #140068, #137503, #158408 ) ;
#53550=DIRECTION ( 'NONE',  ( -1.000000000000000000, 0.000000000000000000, 0.000000000000000000 ) ) ;
#53572=CARTESIAN_POINT ( 'NONE',  ( 5.551115123125782702E-14, 64.35000000001120668, -3.123107484524795474 ) ) ;
#53573=DIRECTION ( 'NONE',  ( -1.000000000000000000, -0.000000000000000000, -0.000000000000000000 ) ) ;
#53673=VERTEX_POINT ( 'NONE', #192011 ) ;
#53786=ORIENTED_EDGE ( 'NONE', *, *, #56196, .F. ) ;
#53860=CARTESIAN_POINT ( 'NONE',  ( 20.95000000000005613, 67.85000000001119247, -3.123107484524795474 ) ) ;
#53881=EDGE_CURVE ( 'NONE', #213499, #160549, #130089, .T. ) ;
#53897=LINE ( 'NONE', #171331, #59533 ) ;
#53925=FACE_OUTER_BOUND ( 'NONE', #196975, .T. ) ;
#53936=DIRECTION ( 'NONE',  ( 1.000000000000000000, 0.000000000000000000, 0.000000000000000000 ) ) ;
#53938=VECTOR ( 'NONE', #92371, 1000.000000000000000 ) ;
#54028=AXIS2_PLACEMENT_3D ( 'NONE', #33860, #92493, #96327 ) ;
#54030=CARTESIAN_POINT ( 'NONE',  ( -40.23850191057533010, 65.19115966511134275, -30.02310748452479316 ) ) ;
#54057=ORIENTED_EDGE ( 'NONE', *, *, #159555, .F. ) ;
#54063=CYLINDRICAL_SURFACE ( 'NONE', #40829, 0.09999999999999939493 ) ;
#54074=DIRECTION ( 'NONE',  ( 0.000000000000000000, -0.000000000000000000, 1.000000000000000000 ) ) ;
#54086=ADVANCED_FACE ( 'NONE', ( #144198 ), #185909, .F. ) ;
#54126=EDGE_CURVE ( 'NONE', #53673, #86047, #81638, .T. ) ;
#54137=AXIS2_PLACEMENT_3D ( 'NONE', #209037, #146474, #248165 ) ;
#54146=ORIENTED_EDGE ( 'NONE', *, *, #122571, .F. ) ;
#54194=DIRECTION ( 'NONE',  ( 0.000000000000000000, 0.000000000000000000, -1.000000000000000000 ) ) ;
#54213=CARTESIAN_POINT ( 'NONE',  ( -21.04999999999994387, 64.35000000001120668, -30.02310748452479316 ) ) ;
#54299=ORIENTED_EDGE ( 'NONE', *, *, #20775, .T. ) ;
#54422=CARTESIAN_POINT ( 'NONE',  ( -23.49999999999994316, 74.94272479589878344, -8.023107484524793165 ) ) ;
#54436=FACE_OUTER_BOUND ( 'NONE', #252872, .T. ) ;
#54474=AXIS2_PLACEMENT_3D ( 'NONE', #253625, #72459, #13752 ) ;
#54483=AXIS2_PLACEMENT_3D ( 'NONE', #221956, #81172, #223259 ) ;
#54555=CARTESIAN_POINT ( 'NONE',  ( 21.15000000000005542, 83.98667523412385094, -37.28476067066772970 ) ) ;
#54597=DIRECTION ( 'NONE',  ( 0.000000000000000000, 2.362176648138631684E-15, -1.000000000000000000 ) ) ;
#54700=DIRECTION ( 'NONE',  ( 0.000000000000000000, 1.000000000000000000, 0.000000000000000000 ) ) ;
#54774=ORIENTED_EDGE ( 'NONE', *, *, #108751, .F. ) ;
#54778=EDGE_LOOP ( 'NONE', ( #163314, #22748, #240782, #149065 ) ) ;
#54836=VECTOR ( 'NONE', #112232, 1000.000000000000000 ) ;
#54878=AXIS2_PLACEMENT_3D ( 'NONE', #43644, #44929, #64492 ) ;
#54888=DIRECTION ( 'NONE',  ( 0.000000000000000000, 0.000000000000000000, 1.000000000000000000 ) ) ;
#54997=ADVANCED_FACE ( 'NONE', ( #208735 ), #6652, .T. ) ;
#54999=ORIENTED_EDGE ( 'NONE', *, *, #233329, .T. ) ;
#55037=AXIS2_PLACEMENT_3D ( 'NONE', #24132, #4530, #81477 ) ;
#55111=AXIS2_PLACEMENT_3D ( 'NONE', #30770, #88114, #71174 ) ;
#55128=DIRECTION ( 'NONE',  ( 0.000000000000000000, 0.000000000000000000, 1.000000000000000000 ) ) ;
#55147=ORIENTED_EDGE ( 'NONE', *, *, #12659, .F. ) ;
#55150=DIRECTION ( 'NONE',  ( 1.444674012291107001E-15, -0.9910827722268042983, 0.1332476588733650935 ) ) ;
#55192=EDGE_CURVE ( 'NONE', #59396, #40979, #122436, .T. ) ;
#55207=ORIENTED_EDGE ( 'NONE', *, *, #149141, .F. ) ;
#55209=EDGE_CURVE ( 'NONE', #80209, #186900, #238965, .T. ) ;
#55293=EDGE_CURVE ( 'NONE', #184620, #117140, #39093, .T. ) ;
#55300=FACE_OUTER_BOUND ( 'NONE', #50152, .T. ) ;
#55318=DIRECTION ( 'NONE',  ( 0.000000000000000000, 0.000000000000000000, 1.000000000000000000 ) ) ;
#55323=CARTESIAN_POINT ( 'NONE',  ( -13.39999999999994529, 64.35000000001120668, -23.62310748452479103 ) ) ;
#55361=AXIS2_PLACEMENT_3D ( 'NONE', #164942, #85367, #188361 ) ;
#55388=ORIENTED_EDGE ( 'NONE', *, *, #190146, .F. ) ;
#55411=CIRCLE ( 'NONE', #134539, 0.09999999999999530098 ) ;
#55519=AXIS2_PLACEMENT_3D ( 'NONE', #132013, #57596, #159303 ) ;
#55566=ORIENTED_EDGE ( 'NONE', *, *, #228458, .F. ) ;
#55580=CARTESIAN_POINT ( 'NONE',  ( 21.15000000000005187, 74.94272479589878344, -3.023107484524792277 ) ) ;
#55631=AXIS2_PLACEMENT_3D ( 'NONE', #16704, #115785, #152376 ) ;
#55748=EDGE_CURVE ( 'NONE', #133820, #12214, #189516, .T. ) ;
#55792=ORIENTED_EDGE ( 'NONE', *, *, #26916, .F. ) ;
#55805=CARTESIAN_POINT ( 'NONE',  ( 6.100000000000049383, 64.25000000001119815, -51.02310748452480738 ) ) ;
#55817=AXIS2_PLACEMENT_3D ( 'NONE', #127336, #86897, #8675 ) ;
#55824=EDGE_CURVE ( 'NONE', #128131, #60636, #135247, .T. ) ;
#55877=TOROIDAL_SURFACE ( 'NONE', #1726, 0.2000000000000000111, 0.1000000000000000056 ) ;
#55882=LINE ( 'NONE', #232003, #255555 ) ;
#55918=ORIENTED_EDGE ( 'NONE', *, *, #178344, .T. ) ;
#55923=ORIENTED_EDGE ( 'NONE', *, *, #253119, .T. ) ;
#55924=AXIS2_PLACEMENT_3D ( 'NONE', #17509, #59172, #94475 ) ;
#55971=LINE ( 'NONE', #35194, #148981 ) ;
#55999=DIRECTION ( 'NONE',  ( 1.733608814749328402E-15, 0.9910827722268042983, 0.1332476588733650935 ) ) ;
#56017=CIRCLE ( 'NONE', #73015, 0.09999999999999939493 ) ;
#56044=CARTESIAN_POINT ( 'NONE',  ( 5.900000000000061640, 64.65000000001120384, -22.12310748452479103 ) ) ;
#56180=FACE_OUTER_BOUND ( 'NONE', #77189, .T. ) ;
#56182=CYLINDRICAL_SURFACE ( 'NONE', #68384, 0.09999999999999635569 ) ;
#56196=EDGE_CURVE ( 'NONE', #73651, #21018, #216453, .T. ) ;
#56210=ORIENTED_EDGE ( 'NONE', *, *, #156519, .F. ) ;
#56238=TOROIDAL_SURFACE ( 'NONE', #202013, 0.2000000000000000111, 0.1000000000000000056 ) ;
#56260=EDGE_CURVE ( 'NONE', #202492, #111962, #60418, .T. ) ;
#56262=CARTESIAN_POINT ( 'NONE',  ( -23.39999999999994529, 76.00000000001119815, -3.123107484524795474 ) ) ;
#56325=LINE ( 'NONE', #1495, #33217 ) ;
#56373=ORIENTED_EDGE ( 'NONE', *, *, #151885, .T. ) ;
#56375=ORIENTED_EDGE ( 'NONE', *, *, #169312, .F. ) ;
#56422=ADVANCED_FACE ( 'NONE', ( #250893 ), #89632, .F. ) ;
#56475=EDGE_CURVE ( 'NONE', #85681, #154033, #206178, .T. ) ;
#56482=AXIS2_PLACEMENT_3D ( 'NONE', #218605, #40027, #101200 ) ;
#56492=EDGE_LOOP ( 'NONE', ( #14340, #133213, #16528, #157885 ) ) ;
#56513=ORIENTED_EDGE ( 'NONE', *, *, #182966, .T. ) ;
#56519=EDGE_LOOP ( 'NONE', ( #153802, #6839, #13264, #77785 ) ) ;
#56611=VERTEX_POINT ( 'NONE', #159528 ) ;
#56734=ADVANCED_FACE ( 'NONE', ( #15549 ), #96318, .F. ) ;
#56754=DIRECTION ( 'NONE',  ( 0.000000000000000000, 0.000000000000000000, 1.000000000000000000 ) ) ;
#56755=ORIENTED_EDGE ( 'NONE', *, *, #719, .F. ) ;
#56776=DIRECTION ( 'NONE',  ( 0.000000000000000000, 0.000000000000000000, -1.000000000000000000 ) ) ;
#56842=EDGE_LOOP ( 'NONE', ( #48545, #210768, #62987, #238345 ) ) ;
#56891=VERTEX_POINT ( 'NONE', #161470 ) ;
#56907=DIRECTION ( 'NONE',  ( 0.000000000000000000, -0.5774316882803290918, -0.8164390028469542537 ) ) ;
#56949=DIRECTION ( 'NONE',  ( 0.000000000000000000, -0.000000000000000000, 1.000000000000000000 ) ) ;
#56979=EDGE_LOOP ( 'NONE', ( #58632, #214193, #179751 ) ) ;
#56988=CARTESIAN_POINT ( 'NONE',  ( 20.95000000000005258, 65.19115966511134275, -30.02310748452479316 ) ) ;
#57005=DIRECTION ( 'NONE',  ( 1.000000000000000000, 0.000000000000000000, 0.000000000000000000 ) ) ;
#57017=ORIENTED_EDGE ( 'NONE', *, *, #160949, .T. ) ;
#57046=AXIS2_PLACEMENT_3D ( 'NONE', #173938, #176476, #14843 ) ;
#57126=DIRECTION ( 'NONE',  ( -0.000000000000000000, 0.000000000000000000, 1.000000000000000000 ) ) ;
#57159=DIRECTION ( 'NONE',  ( -1.000000000000000000, 0.000000000000000000, 0.000000000000000000 ) ) ;
#57264=FACE_OUTER_BOUND ( 'NONE', #177900, .T. ) ;
#57278=DIRECTION ( 'NONE',  ( 0.000000000000000000, 0.000000000000000000, 1.000000000000000000 ) ) ;
#57313=ORIENTED_EDGE ( 'NONE', *, *, #196851, .T. ) ;
#57316=DIRECTION ( 'NONE',  ( 1.000000000000000000, 0.000000000000000000, 0.000000000000000000 ) ) ;
#57362=CIRCLE ( 'NONE', #207247, 0.1000000000000028644 ) ;
#57466=DIRECTION ( 'NONE',  ( 0.000000000000000000, -0.1480365673253065395, 0.9889818879709274535 ) ) ;
#57481=ADVANCED_FACE ( 'NONE', ( #187146 ), #123305, .F. ) ;
#57539=CARTESIAN_POINT ( 'NONE',  ( 21.05000000000005400, 65.15000000001120384, -4.423107484524790856 ) ) ;
#57562=DIRECTION ( 'NONE',  ( 1.000000000000000000, -0.000000000000000000, -0.000000000000000000 ) ) ;
#57587=CARTESIAN_POINT ( 'NONE',  ( -20.94999999999994600, 66.15000000001120384, -4.623107484524796362 ) ) ;
#57596=DIRECTION ( 'NONE',  ( -1.444674012291107001E-15, 0.1332476588733650935, 0.9910827722268042983 ) ) ;
#57624=CARTESIAN_POINT ( 'NONE',  ( 23.40000000000005542, 83.80000000001119531, -34.86056257560453986 ) ) ;
#57677=CARTESIAN_POINT ( 'NONE',  ( 21.15000000000005542, 87.50449464844290048, -34.18759587077607165 ) ) ;
#57680=CARTESIAN_POINT ( 'NONE',  ( 23.40000000000005542, 74.16448838626247664, -47.52760213295649550 ) ) ;
#57699=ADVANCED_FACE ( 'NONE', ( #256024 ), #77421, .F. ) ;
#57713=DIRECTION ( 'NONE',  ( 6.423964682151766729E-15, 0.1575546449569727725, 0.9875102702516478370 ) ) ;
#57718=DIRECTION ( 'NONE',  ( 0.000000000000000000, -0.4856429311786292224, -0.8741572761215394838 ) ) ;
#57819=VERTEX_POINT ( 'NONE', #121729 ) ;
#57846=ADVANCED_FACE ( 'NONE', ( #164693 ), #223362, .T. ) ;
#57955=EDGE_LOOP ( 'NONE', ( #143602, #12772, #107182, #174390 ) ) ;
#58016=ORIENTED_EDGE ( 'NONE', *, *, #194843, .F. ) ;
#58050=FACE_OUTER_BOUND ( 'NONE', #38912, .T. ) ;
#58100=CIRCLE ( 'NONE', #45480, 0.1999999999999996503 ) ;
#58120=CARTESIAN_POINT ( 'NONE',  ( -13.39999999999994351, 67.65000000001118963, -16.98168612828748181 ) ) ;
#58134=EDGE_CURVE ( 'NONE', #170630, #179524, #110660, .T. ) ;
#58135=DIRECTION ( 'NONE',  ( 0.000000000000000000, 0.000000000000000000, 1.000000000000000000 ) ) ;
#58155=DIRECTION ( 'NONE',  ( 0.000000000000000000, -0.000000000000000000, -1.000000000000000000 ) ) ;
#58156=VERTEX_POINT ( 'NONE', #137125 ) ;
#58158=VECTOR ( 'NONE', #5026, 1000.000000000000000 ) ;
#58229=DIRECTION ( 'NONE',  ( 0.000000000000000000, 0.7071067811865473507, -0.7071067811865477948 ) ) ;
#58232=AXIS2_PLACEMENT_3D ( 'NONE', #207525, #9304, #28922 ) ;
#58244=AXIS2_PLACEMENT_3D ( 'NONE', #103920, #141779, #204318 ) ;
#58262=FACE_OUTER_BOUND ( 'NONE', #3291, .T. ) ;
#58284=PLANE ( 'NONE',  #246022 ) ;
#58338=DIRECTION ( 'NONE',  ( 1.000000000000000000, 0.000000000000000000, 0.000000000000000000 ) ) ;
#58345=VECTOR ( 'NONE', #99881, 1000.000000000000000 ) ;
#58370=ORIENTED_EDGE ( 'NONE', *, *, #62942, .T. ) ;
#58376=LINE ( 'NONE', #55805, #139200 ) ;
#58406=FACE_OUTER_BOUND ( 'NONE', #153043, .T. ) ;
#58457=DIRECTION ( 'NONE',  ( 1.000000000000000000, 0.000000000000000000, 0.000000000000000000 ) ) ;
#58519=AXIS2_PLACEMENT_3D ( 'NONE', #130547, #190553, #52280 ) ;
#58520=DIRECTION ( 'NONE',  ( 0.000000000000000000, -0.9875102702516471709, 0.1575546449569757979 ) ) ;
#58543=LINE ( 'NONE', #118561, #203117 ) ;
#58552=DIRECTION ( 'NONE',  ( 0.000000000000000000, 1.000000000000000000, 0.000000000000000000 ) ) ;
#58558=DIRECTION ( 'NONE',  ( 0.000000000000000000, -1.000000000000000000, 0.000000000000000000 ) ) ;
#58592=AXIS2_PLACEMENT_3D ( 'NONE', #100030, #19238, #154934 ) ;
#58623=ORIENTED_EDGE ( 'NONE', *, *, #124509, .T. ) ;
#58632=ORIENTED_EDGE ( 'NONE', *, *, #102474, .F. ) ;
#58660=DIRECTION ( 'NONE',  ( -1.000000000000000000, -0.000000000000000000, -0.000000000000000000 ) ) ;
#58723=DIRECTION ( 'NONE',  ( 0.000000000000000000, 1.156482317317873105E-15, 1.000000000000000000 ) ) ;
#58763=ADVANCED_FACE ( 'NONE', ( #170226 ), #150613, .F. ) ;
#58780=EDGE_LOOP ( 'NONE', ( #156868, #140983, #140869, #115238 ) ) ;
#58800=DIRECTION ( 'NONE',  ( -1.000000000000000000, 4.624352451196580357E-15, 3.439547145395922042E-14 ) ) ;
#58872=SPHERICAL_SURFACE ( 'NONE', #27845, 0.1000000000000000056 ) ;
#58968=CIRCLE ( 'NONE', #163074, 0.09999999999999939493 ) ;
#59013=CIRCLE ( 'NONE', #175782, 0.09999999999999982514 ) ;
#59049=AXIS2_PLACEMENT_3D ( 'NONE', #181577, #23803, #83695 ) ;
#59085=CARTESIAN_POINT ( 'NONE',  ( -20.94999999999994600, 67.85000000001119247, -25.49719488170504533 ) ) ;
#59094=AXIS2_PLACEMENT_3D ( 'NONE', #196396, #125537, #77720 ) ;
#59095=ORIENTED_EDGE ( 'NONE', *, *, #250769, .F. ) ;
#59147=EDGE_CURVE ( 'NONE', #210574, #51994, #190157, .T. ) ;
#59172=DIRECTION ( 'NONE',  ( 1.000000000000000000, 0.000000000000000000, 0.000000000000000000 ) ) ;
#59188=ORIENTED_EDGE ( 'NONE', *, *, #14679, .T. ) ;
#59245=CARTESIAN_POINT ( 'NONE',  ( -5.899999999999938183, 64.75000000001119815, -22.12310748452479103 ) ) ;
#59338=CARTESIAN_POINT ( 'NONE',  ( -21.04999999999994387, 66.15000000001120384, -5.923107484524795296 ) ) ;
#59396=VERTEX_POINT ( 'NONE', #189131 ) ;
#59401=VECTOR ( 'NONE', #32796, 1000.000000000000000 ) ;
#59404=FACE_OUTER_BOUND ( 'NONE', #82174, .T. ) ;
#59424=DIRECTION ( 'NONE',  ( 0.000000000000000000, 1.181088324069315448E-15, 1.000000000000000000 ) ) ;
#59491=CARTESIAN_POINT ( 'NONE',  ( -23.49999999999994316, 64.35000000001120668, -36.02310748452479316 ) ) ;
#59493=VERTEX_POINT ( 'NONE', #238521 ) ;
#59533=VECTOR ( 'NONE', #150448, 1000.000000000000000 ) ;
#59551=CYLINDRICAL_SURFACE ( 'NONE', #164028, 11.74999999999999645 ) ;
#59606=SPHERICAL_SURFACE ( 'NONE', #72746, 0.1000000000000000056 ) ;
#59642=CARTESIAN_POINT ( 'NONE',  ( -20.94999999999994245, 67.65000000001118963, -3.123107484524795474 ) ) ;
#59645=ADVANCED_FACE ( 'NONE', ( #63735 ), #242368, .T. ) ;
#59659=VECTOR ( 'NONE', #3256, 1000.000000000000000 ) ;
#59692=ADVANCED_FACE ( 'NONE', ( #101546 ), #186268, .F. ) ;
#59725=DIRECTION ( 'NONE',  ( 0.000000000000000000, 1.000000000000000000, 0.000000000000000000 ) ) ;
#59791=ORIENTED_EDGE ( 'NONE', *, *, #146774, .T. ) ;
#59796=CARTESIAN_POINT ( 'NONE',  ( -13.39999999999994529, 67.75000000001118394, -16.98168612828748181 ) ) ;
#59798=CARTESIAN_POINT ( 'NONE',  ( -23.39999999999994529, 87.50449464844290048, -37.85861909827351468 ) ) ;
#59830=FACE_OUTER_BOUND ( 'NONE', #1441, .T. ) ;
#59854=ORIENTED_EDGE ( 'NONE', *, *, #144943, .T. ) ;
#59944=EDGE_CURVE ( 'NONE', #196305, #257282, #87653, .T. ) ;
#59948=CYLINDRICAL_SURFACE ( 'NONE', #155662, 0.1000000000000028644 ) ;
#59983=DIRECTION ( 'NONE',  ( 0.000000000000000000, 0.000000000000000000, -1.000000000000000000 ) ) ;
#59984=DIRECTION ( 'NONE',  ( 0.000000000000000000, 0.1332476588733589318, 0.9910827722268049644 ) ) ;
#60006=DIRECTION ( 'NONE',  ( 0.000000000000000000, -1.000000000000000000, 0.000000000000000000 ) ) ;
#60011=DIRECTION ( 'NONE',  ( 0.000000000000000000, 0.000000000000000000, -1.000000000000000000 ) ) ;
#60029=CIRCLE ( 'NONE', #76604, 0.1000000000000002554 ) ;
#60039=DIRECTION ( 'NONE',  ( 0.000000000000000000, 0.000000000000000000, 1.000000000000000000 ) ) ;
#60081=VECTOR ( 'NONE', #8191, 1000.000000000000000 ) ;
#60123=VERTEX_POINT ( 'NONE', #10258 ) ;
#60163=CARTESIAN_POINT ( 'NONE',  ( -23.39999999999994529, 82.72707916847673459, -26.51159310135756897 ) ) ;
#60240=CARTESIAN_POINT ( 'NONE',  ( -23.39999999999994529, 84.00000000001119815, -37.18565239344504647 ) ) ;
#60247=ORIENTED_EDGE ( 'NONE', *, *, #133750, .T. ) ;
#60349=VECTOR ( 'NONE', #198424, 1000.000000000000000 ) ;
#60418=CIRCLE ( 'NONE', #85337, 5.000000000000000888 ) ;
#60442=CARTESIAN_POINT ( 'NONE',  ( 21.15000000000005542, 82.74366731733570646, -26.36310895752070138 ) ) ;
#60483=CIRCLE ( 'NONE', #218887, 0.1999999999999996503 ) ;
#60513=EDGE_CURVE ( 'NONE', #104499, #118363, #58968, .T. ) ;
#60519=VECTOR ( 'NONE', #171434, 1000.000000000000000 ) ;
#60527=EDGE_CURVE ( 'NONE', #89909, #235335, #134004, .T. ) ;
#60586=EDGE_LOOP ( 'NONE', ( #153524, #126120, #159048, #9233 ) ) ;
#60596=VERTEX_POINT ( 'NONE', #205550 ) ;
#60602=CARTESIAN_POINT ( 'NONE',  ( -11.59999999999994458, 66.35000000001119247, -18.42310748452479174 ) ) ;
#60617=DIRECTION ( 'NONE',  ( 0.000000000000000000, 0.000000000000000000, 1.000000000000000000 ) ) ;
#60632=CARTESIAN_POINT ( 'NONE',  ( 5.900000000000059863, 64.65000000001120384, -25.92310748452479174 ) ) ;
#60636=VERTEX_POINT ( 'NONE', #192430 ) ;
#60641=ADVANCED_FACE ( 'NONE', ( #232857 ), #129892, .T. ) ;
#60653=ORIENTED_EDGE ( 'NONE', *, *, #70480, .T. ) ;
#60678=CYLINDRICAL_SURFACE ( 'NONE', #68980, 0.1000000000000021844 ) ;
#60698=ORIENTED_EDGE ( 'NONE', *, *, #119766, .F. ) ;
#60723=VERTEX_POINT ( 'NONE', #60602 ) ;
#60727=FACE_BOUND ( 'NONE', #240556, .T. ) ;
#60752=CARTESIAN_POINT ( 'NONE',  ( -23.39999999999994529, 76.00000000001119815, -31.97310748452479601 ) ) ;
#60754=CARTESIAN_POINT ( 'NONE',  ( -11.59999999999994458, 67.72071067812984779, -21.02310748452479316 ) ) ;
#60761=ORIENTED_EDGE ( 'NONE', *, *, #82603, .T. ) ;
#60778=FACE_OUTER_BOUND ( 'NONE', #95441, .T. ) ;
#60801=DIRECTION ( 'NONE',  ( -1.000000000000000000, 0.000000000000000000, -0.000000000000000000 ) ) ;
#60807=ORIENTED_EDGE ( 'NONE', *, *, #34730, .T. ) ;
#60819=CARTESIAN_POINT ( 'NONE',  ( -0.8999999999999437339, 66.35000000001119247, -10.02310748452479139 ) ) ;
#60922=DIRECTION ( 'NONE',  ( 1.000000000000000000, 0.000000000000000000, 0.000000000000000000 ) ) ;
#60949=DIRECTION ( 'NONE',  ( 0.000000000000000000, 0.8741572761215280485, -0.4856429311786498171 ) ) ;
#60970=EDGE_CURVE ( 'NONE', #6953, #30427, #168769, .T. ) ;
#60974=EDGE_LOOP ( 'NONE', ( #85160, #189381, #127104, #255279, #163358, #25826, #26344, #19913, #108439, #145119, #229710, #199222, #242386, #182046, #127061, #83139 ) ) ;
#61009=EDGE_CURVE ( 'NONE', #257282, #18100, #192150, .T. ) ;
#61070=CARTESIAN_POINT ( 'NONE',  ( -23.49999999999994316, 83.80000000001119531, -37.18565239344504647 ) ) ;
#61072=EDGE_CURVE ( 'NONE', #191279, #211462, #125990, .T. ) ;
#61080=DIRECTION ( 'NONE',  ( 0.000000000000000000, 1.000000000000000000, 0.000000000000000000 ) ) ;
#61082=VECTOR ( 'NONE', #172437, 1000.000000000000000 ) ;
#61204=DIRECTION ( 'NONE',  ( 0.000000000000000000, 0.000000000000000000, 1.000000000000000000 ) ) ;
#61233=EDGE_CURVE ( 'NONE', #26247, #200341, #42792, .T. ) ;
#61234=CARTESIAN_POINT ( 'NONE',  ( 21.15000000000004476, 77.16254490893143725, -44.02310748452479316 ) ) ;
#61238=CIRCLE ( 'NONE', #44506, 0.1000000000000028644 ) ;
#61249=DIRECTION ( 'NONE',  ( -0.000000000000000000, 1.000000000000000000, -0.000000000000000000 ) ) ;
#61306=AXIS2_PLACEMENT_3D ( 'NONE', #89600, #244827, #45354 ) ;
#61312=VERTEX_POINT ( 'NONE', #192781 ) ;
#61318=ADVANCED_FACE ( 'NONE', ( #190216 ), #188925, .F. ) ;
#61325=DIRECTION ( 'NONE',  ( 0.000000000000000000, -0.4856429311786307768, -0.8741572761215385956 ) ) ;
#61336=CARTESIAN_POINT ( 'NONE',  ( 21.15000000000005187, 76.00000000001119815, -36.02310748452479316 ) ) ;
#61356=CIRCLE ( 'NONE', #207123, 0.09999999999999939493 ) ;
#61404=EDGE_CURVE ( 'NONE', #84197, #183369, #92854, .T. ) ;
#61441=ADVANCED_FACE ( 'NONE', ( #218729 ), #98761, .T. ) ;
#61477=DIRECTION ( 'NONE',  ( 0.000000000000000000, 0.000000000000000000, 1.000000000000000000 ) ) ;
#61487=AXIS2_PLACEMENT_3D ( 'NONE', #160566, #22339, #240084 ) ;
#61513=EDGE_CURVE ( 'NONE', #135372, #149012, #46513, .T. ) ;
#61540=DIRECTION ( 'NONE',  ( 0.000000000000000000, 0.000000000000000000, 1.000000000000000000 ) ) ;
#61561=CARTESIAN_POINT ( 'NONE',  ( -21.04999999999994387, 66.15000000001120384, -6.023107484524794941 ) ) ;
#61568=DIRECTION ( 'NONE',  ( -0.000000000000000000, 1.000000000000000000, -0.000000000000000000 ) ) ;
#61639=DIRECTION ( 'NONE',  ( -1.000000000000000000, 0.000000000000000000, 0.000000000000000000 ) ) ;
#61659=ORIENTED_EDGE ( 'NONE', *, *, #177797, .F. ) ;
#61669=VERTEX_POINT ( 'NONE', #52941 ) ;
#61675=ORIENTED_EDGE ( 'NONE', *, *, #77710, .F. ) ;
#61678=ORIENTED_EDGE ( 'NONE', *, *, #113581, .T. ) ;
#61740=DIRECTION ( 'NONE',  ( -0.000000000000000000, 1.000000000000000000, -0.000000000000000000 ) ) ;
#61742=AXIS2_PLACEMENT_3D ( 'NONE', #230955, #190543, #113548 ) ;
#61814=DIRECTION ( 'NONE',  ( -0.000000000000000000, 1.000000000000000000, -0.000000000000000000 ) ) ;
#61829=DIRECTION ( 'NONE',  ( -1.000000000000000000, 0.000000000000000000, 0.000000000000000000 ) ) ;
#61833=CYLINDRICAL_SURFACE ( 'NONE', #220746, 0.1000000000000021844 ) ;
#61854=DIRECTION ( 'NONE',  ( 1.000000000000000000, 0.000000000000000000, 0.000000000000000000 ) ) ;
#61896=DIRECTION ( 'NONE',  ( -1.000000000000000000, 0.000000000000000000, 0.000000000000000000 ) ) ;
#61897=ORIENTED_EDGE ( 'NONE', *, *, #33972, .T. ) ;
#61904=ORIENTED_EDGE ( 'NONE', *, *, #50299, .F. ) ;
#61929=EDGE_CURVE ( 'NONE', #146220, #197879, #80541, .T. ) ;
#61957=AXIS2_PLACEMENT_3D ( 'NONE', #155078, #195484, #36407 ) ;
#61967=ORIENTED_EDGE ( 'NONE', *, *, #138199, .F. ) ;
#62001=VERTEX_POINT ( 'NONE', #24123 ) ;
#62069=VERTEX_POINT ( 'NONE', #128351 ) ;
#62082=CARTESIAN_POINT ( 'NONE',  ( 6.000000000000060396, 64.35000000001120668, -25.92310748452479174 ) ) ;
#62164=LINE ( 'NONE', #197807, #50354 ) ;
#62195=DIRECTION ( 'NONE',  ( -0.000000000000000000, 1.000000000000000000, -0.000000000000000000 ) ) ;
#62235=AXIS2_PLACEMENT_3D ( 'NONE', #204129, #224967, #85441 ) ;
#62324=DIRECTION ( 'NONE',  ( 0.000000000000000000, 0.000000000000000000, 1.000000000000000000 ) ) ;
#62349=EDGE_CURVE ( 'NONE', #210574, #45940, #179055, .T. ) ;
#62506=DIRECTION ( 'NONE',  ( -1.000000000000000000, 0.000000000000000000, 0.000000000000000000 ) ) ;
#62511=CARTESIAN_POINT ( 'NONE',  ( -23.49999999999994316, 74.16448838626247664, -47.62760213295649692 ) ) ;
#62533=DIRECTION ( 'NONE',  ( 0.000000000000000000, 0.000000000000000000, -1.000000000000000000 ) ) ;
#62574=DIRECTION ( 'NONE',  ( 1.000000000000000000, -0.000000000000000000, -0.000000000000000000 ) ) ;
#62649=ADVANCED_FACE ( 'NONE', ( #56180 ), #72583, .T. ) ;
#62657=ORIENTED_EDGE ( 'NONE', *, *, #41876, .F. ) ;
#62721=DIRECTION ( 'NONE',  ( -0.000000000000000000, 1.000000000000000000, -0.000000000000000000 ) ) ;
#62748=VECTOR ( 'NONE', #119127, 1000.000000000000000 ) ;
#62758=FACE_OUTER_BOUND ( 'NONE', #1121, .T. ) ;
#62765=ADVANCED_FACE ( 'NONE', ( #80876 ), #97859, .F. ) ;
#62838=CARTESIAN_POINT ( 'NONE',  ( 21.05000000000005400, 82.64476912853859858, -26.37791261425322986 ) ) ;
#62841=ADVANCED_FACE ( 'NONE', ( #23531 ), #139565, .T. ) ;
#62876=EDGE_CURVE ( 'NONE', #137320, #66524, #243237, .T. ) ;
#62926=DIRECTION ( 'NONE',  ( 0.000000000000000000, 0.000000000000000000, -1.000000000000000000 ) ) ;
#62942=EDGE_CURVE ( 'NONE', #134658, #187156, #225511, .T. ) ;
#62968=VECTOR ( 'NONE', #31198, 1000.000000000000000 ) ;
#62987=ORIENTED_EDGE ( 'NONE', *, *, #227971, .F. ) ;
#63025=ORIENTED_EDGE ( 'NONE', *, *, #197713, .F. ) ;
#63076=ORIENTED_EDGE ( 'NONE', *, *, #127605, .F. ) ;
#63085=LINE ( 'NONE', #219587, #146608 ) ;
#63086=ORIENTED_EDGE ( 'NONE', *, *, #139837, .T. ) ;
#63095=CARTESIAN_POINT ( 'NONE',  ( -21.14999999999994174, 69.83923505573476120, -35.48358590217651454 ) ) ;
#63115=VERTEX_POINT ( 'NONE', #138903 ) ;
#63117=FACE_OUTER_BOUND ( 'NONE', #120188, .T. ) ;
#63153=CYLINDRICAL_SURFACE ( 'NONE', #211077, 0.09999999999999939493 ) ;
#63173=ORIENTED_EDGE ( 'NONE', *, *, #97292, .T. ) ;
#63228=EDGE_CURVE ( 'NONE', #255132, #46490, #211771, .T. ) ;
#63274=CARTESIAN_POINT ( 'NONE',  ( -20.94999999999994245, 67.85000000001119247, -3.023107484524792277 ) ) ;
#63415=VECTOR ( 'NONE', #23019, 1000.000000000000000 ) ;
#63550=CARTESIAN_POINT ( 'NONE',  ( 5.900000000000061640, 64.65000000001120384, -22.12310748452479103 ) ) ;
#63603=DIRECTION ( 'NONE',  ( 0.000000000000000000, 0.000000000000000000, -1.000000000000000000 ) ) ;
#63614=ORIENTED_EDGE ( 'NONE', *, *, #118898, .T. ) ;
#63618=VECTOR ( 'NONE', #187352, 1000.000000000000000 ) ;
#63650=ORIENTED_EDGE ( 'NONE', *, *, #69337, .F. ) ;
#63735=FACE_OUTER_BOUND ( 'NONE', #149067, .T. ) ;
#63736=CIRCLE ( 'NONE', #180439, 0.09999999999999939493 ) ;
#63789=ORIENTED_EDGE ( 'NONE', *, *, #118912, .T. ) ;
#63922=ORIENTED_EDGE ( 'NONE', *, *, #44029, .T. ) ;
#63929=EDGE_CURVE ( 'NONE', #33086, #43374, #172560, .T. ) ;
#64072=ORIENTED_EDGE ( 'NONE', *, *, #198891, .T. ) ;
#64134=EDGE_CURVE ( 'NONE', #211462, #255132, #193543, .T. ) ;
#64147=ADVANCED_FACE ( 'NONE', ( #88310 ), #111764, .T. ) ;
#64166=LINE ( 'NONE', #23786, #221709 ) ;
#64217=ORIENTED_EDGE ( 'NONE', *, *, #215398, .T. ) ;
#64265=VERTEX_POINT ( 'NONE', #37375 ) ;
#64312=AXIS2_PLACEMENT_3D ( 'NONE', #192462, #214577, #132487 ) ;
#64360=DIRECTION ( 'NONE',  ( 1.000000000000000000, -0.000000000000000000, -0.000000000000000000 ) ) ;
#64379=CARTESIAN_POINT ( 'NONE',  ( -0.8999999999999437339, 67.75000000001118394, -5.981686128287480919 ) ) ;
#64416=DIRECTION ( 'NONE',  ( 0.000000000000000000, -0.9910827722268042983, 0.1332476588733650935 ) ) ;
#64444=ORIENTED_EDGE ( 'NONE', *, *, #1769, .T. ) ;
#64446=CIRCLE ( 'NONE', #160328, 4.049999999999998046 ) ;
#64470=EDGE_LOOP ( 'NONE', ( #124920, #152055, #130, #50428 ) ) ;
#64492=DIRECTION ( 'NONE',  ( 0.000000000000000000, 0.000000000000000000, -1.000000000000000000 ) ) ;
#64526=EDGE_CURVE ( 'NONE', #82762, #80585, #182008, .T. ) ;
#64528=AXIS2_PLACEMENT_3D ( 'NONE', #106288, #172435, #154157 ) ;
#64548=EDGE_LOOP ( 'NONE', ( #119819, #204770, #8249, #69307 ) ) ;
#64552=EDGE_CURVE ( 'NONE', #114106, #226270, #114607, .T. ) ;
#64576=DIRECTION ( 'NONE',  ( 0.000000000000000000, 0.000000000000000000, -1.000000000000000000 ) ) ;
#64587=EDGE_CURVE ( 'NONE', #52328, #251948, #211522, .T. ) ;
#64638=EDGE_CURVE ( 'NONE', #28434, #8217, #122996, .T. ) ;
#64665=AXIS2_PLACEMENT_3D ( 'NONE', #133811, #170435, #210790 ) ;
#64694=ORIENTED_EDGE ( 'NONE', *, *, #253975, .F. ) ;
#64742=VECTOR ( 'NONE', #201715, 1000.000000000000000 ) ;
#64746=EDGE_CURVE ( 'NONE', #201487, #23181, #220517, .T. ) ;
#64800=DIRECTION ( 'NONE',  ( 1.000000000000000000, -0.000000000000000000, -0.000000000000000000 ) ) ;
#64823=ADVANCED_FACE ( 'NONE', ( #87401 ), #203515, .T. ) ;
#64824=CARTESIAN_POINT ( 'NONE',  ( 21.05000000000005400, 74.83745509109094485, -43.82310748452479743 ) ) ;
#64847=EDGE_CURVE ( 'NONE', #205114, #211183, #45718, .T. ) ;
#64879=CARTESIAN_POINT ( 'NONE',  ( 0.9000000000000547562, 64.35000000001120668, -7.423107484524793520 ) ) ;
#64885=ORIENTED_EDGE ( 'NONE', *, *, #64552, .F. ) ;
#64926=CARTESIAN_POINT ( 'NONE',  ( -23.49999999999994316, 76.00000000001119815, -36.02310748452479316 ) ) ;
#64966=VERTEX_POINT ( 'NONE', #36461 ) ;
#64981=TOROIDAL_SURFACE ( 'NONE', #69289, 4.041421356237310469, 0.1000000000000000056 ) ;
#64995=CIRCLE ( 'NONE', #52514, 3.970710678118657189 ) ;
#65093=DIRECTION ( 'NONE',  ( 0.000000000000000000, 0.7071067811865472397, -0.7071067811865479058 ) ) ;
#65153=CARTESIAN_POINT ( 'NONE',  ( -13.39999999999994351, 64.35000000001120668, -23.72310748452479245 ) ) ;
#65159=CARTESIAN_POINT ( 'NONE',  ( 23.50000000000005684, 83.80000000001119531, -34.86056257560453986 ) ) ;
#65211=AXIS2_PLACEMENT_3D ( 'NONE', #38570, #17702, #157260 ) ;
#65222=AXIS2_PLACEMENT_3D ( 'NONE', #77713, #195144, #138954 ) ;
#65252=EDGE_CURVE ( 'NONE', #143490, #183369, #247460, .T. ) ;
#65270=EDGE_CURVE ( 'NONE', #250175, #168296, #219017, .T. ) ;
#65322=LINE ( 'NONE', #241410, #223548 ) ;
#65331=ADVANCED_FACE ( 'NONE', ( #10142 ), #128814, .T. ) ;
#65349=CARTESIAN_POINT ( 'NONE',  ( 13.40000000000005898, 64.35000000001120668, -18.32310748452479743 ) ) ;
#65402=ADVANCED_FACE ( 'NONE', ( #197755 ), #135198, .F. ) ;
#65408=EDGE_CURVE ( 'NONE', #249539, #15261, #178225, .T. ) ;
#65417=SPHERICAL_SURFACE ( 'NONE', #169261, 0.1000000000000000056 ) ;
#65444=ORIENTED_EDGE ( 'NONE', *, *, #80409, .T. ) ;
#65458=DIRECTION ( 'NONE',  ( 3.469446951953515108E-14, 1.000000000000000000, 0.000000000000000000 ) ) ;
#65477=ORIENTED_EDGE ( 'NONE', *, *, #249965, .T. ) ;
#65498=CIRCLE ( 'NONE', #211269, 0.09999999999999939493 ) ;
#65513=VERTEX_POINT ( 'NONE', #195225 ) ;
#65523=ORIENTED_EDGE ( 'NONE', *, *, #15540, .F. ) ;
#65524=AXIS2_PLACEMENT_3D ( 'NONE', #4591, #24188, #243205 ) ;
#65526=AXIS2_PLACEMENT_3D ( 'NONE', #6567, #86073, #224332 ) ;
#65553=AXIS2_PLACEMENT_3D ( 'NONE', #88408, #243656, #207111 ) ;
#65564=AXIS2_PLACEMENT_3D ( 'NONE', #255754, #32943, #137140 ) ;
#65613=ORIENTED_EDGE ( 'NONE', *, *, #81032, .F. ) ;
#65703=CARTESIAN_POINT ( 'NONE',  ( -21.04999999999994387, 67.75000000001118394, -25.49719488170504533 ) ) ;
#65710=CARTESIAN_POINT ( 'NONE',  ( -21.14999999999994174, 82.72707916847673459, -26.51159310135756897 ) ) ;
#65713=CARTESIAN_POINT ( 'NONE',  ( -23.49999999999994316, 83.90000000001120384, -34.77310748452479316 ) ) ;
#65734=CARTESIAN_POINT ( 'NONE',  ( -5.899999999999938183, 64.75000000001119815, -25.92310748452479174 ) ) ;
#65767=CARTESIAN_POINT ( 'NONE',  ( 21.15000000000005542, 64.35000000001120668, -3.123107484524795474 ) ) ;
#65800=DIRECTION ( 'NONE',  ( 0.000000000000000000, -1.000000000000000000, 0.000000000000000000 ) ) ;
#65857=DIRECTION ( 'NONE',  ( 0.000000000000000000, 0.000000000000000000, -1.000000000000000000 ) ) ;
#65960=AXIS2_PLACEMENT_3D ( 'NONE', #66517, #186467, #245155 ) ;
#65975=CARTESIAN_POINT ( 'NONE',  ( -40.23850191057533010, 87.75000000001119815, -6.023107484524794941 ) ) ;
#66074=EDGE_LOOP ( 'NONE', ( #5491, #156169, #90225, #170499 ) ) ;
#66087=CARTESIAN_POINT ( 'NONE',  ( 11.60000000000006004, 67.72071067812984779, -24.99381816264344991 ) ) ;
#66099=LINE ( 'NONE', #29578, #63618 ) ;
#66120=TOROIDAL_SURFACE ( 'NONE', #207608, 11.65000000000000036, 0.1000000000000000056 ) ;
#66127=DIRECTION ( 'NONE',  ( -1.000000000000000000, 0.000000000000000000, 0.000000000000000000 ) ) ;
#66146=DIRECTION ( 'NONE',  ( 0.000000000000000000, 0.000000000000000000, -1.000000000000000000 ) ) ;
#66157=EDGE_CURVE ( 'NONE', #15171, #252227, #194474, .T. ) ;
#66194=ADVANCED_FACE ( 'NONE', ( #117615 ), #155496, .T. ) ;
#66200=TOROIDAL_SURFACE ( 'NONE', #120227, 0.2000000000000000111, 0.1000000000000000056 ) ;
#66210=CARTESIAN_POINT ( 'NONE',  ( 23.40000000000005542, 77.16254490893143725, -43.82310748452479743 ) ) ;
#66218=EDGE_LOOP ( 'NONE', ( #158675, #56375, #232320, #172470 ) ) ;
#66251=VECTOR ( 'NONE', #174116, 1000.000000000000000 ) ;
#66281=ORIENTED_EDGE ( 'NONE', *, *, #99980, .F. ) ;
#66298=LINE ( 'NONE', #105374, #72627 ) ;
#66307=DIRECTION ( 'NONE',  ( 1.000000000000000000, 0.000000000000000000, 0.000000000000000000 ) ) ;
#66371=AXIS2_PLACEMENT_3D ( 'NONE', #67329, #145573, #6060 ) ;
#66404=DIRECTION ( 'NONE',  ( 0.000000000000000000, -1.000000000000000000, 0.000000000000000000 ) ) ;
#66414=ORIENTED_EDGE ( 'NONE', *, *, #185293, .F. ) ;
#66453=ORIENTED_EDGE ( 'NONE', *, *, #184155, .T. ) ;
#66517=CARTESIAN_POINT ( 'NONE',  ( -23.39999999999994529, 74.94272479589878344, -3.123107484524795474 ) ) ;
#66519=AXIS2_PLACEMENT_3D ( 'NONE', #100834, #4333, #205096 ) ;
#66524=VERTEX_POINT ( 'NONE', #209667 ) ;
#66537=EDGE_LOOP ( 'NONE', ( #216400, #14257, #137720, #112062 ) ) ;
#66547=ORIENTED_EDGE ( 'NONE', *, *, #99862, .T. ) ;
#66641=DIRECTION ( 'NONE',  ( 1.000000000000000000, 0.000000000000000000, 0.000000000000000000 ) ) ;
#66799=AXIS2_PLACEMENT_3D ( 'NONE', #6102, #101311, #60949 ) ;
#66817=ORIENTED_EDGE ( 'NONE', *, *, #175582, .F. ) ;
#66838=LINE ( 'NONE', #6859, #173414 ) ;
#66857=VECTOR ( 'NONE', #98857, 1000.000000000000000 ) ;
#66883=LINE ( 'NONE', #166017, #19937 ) ;
#66892=FILL_AREA_STYLE_COLOUR ( '', #122884 ) ;
#66894=CIRCLE ( 'NONE', #121095, 0.1000000000000028644 ) ;
#66913=DIRECTION ( 'NONE',  ( 0.000000000000000000, 1.000000000000000000, 0.000000000000000000 ) ) ;
#66919=DIRECTION ( 'NONE',  ( -0.000000000000000000, -1.000000000000000000, -0.000000000000000000 ) ) ;
#66976=SPHERICAL_SURFACE ( 'NONE', #7576, 0.1000000000000000056 ) ;
#66986=CARTESIAN_POINT ( 'NONE',  ( -23.39999999999994529, 82.84256550613280012, -26.34830530078816935 ) ) ;
#67000=CARTESIAN_POINT ( 'NONE',  ( 5.900000000000059863, 64.35000000001120668, -25.92310748452479174 ) ) ;
#67024=EDGE_CURVE ( 'NONE', #231870, #34933, #253067, .T. ) ;
#67053=ORIENTED_EDGE ( 'NONE', *, *, #158079, .T. ) ;
#67075=CARTESIAN_POINT ( 'NONE',  ( -23.49999999999994316, 74.94272479589878344, -8.023107484524793165 ) ) ;
#67076=DIRECTION ( 'NONE',  ( 0.000000000000000000, 0.1332476588733589318, -0.9910827722268049644 ) ) ;
#67100=EDGE_CURVE ( 'NONE', #15908, #15171, #107500, .T. ) ;
#67103=DIRECTION ( 'NONE',  ( 0.000000000000000000, 0.000000000000000000, -1.000000000000000000 ) ) ;
#67203=DIRECTION ( 'NONE',  ( 0.000000000000000000, 0.000000000000000000, 1.000000000000000000 ) ) ;
#67297=CIRCLE ( 'NONE', #29740, 4.150000000000001243 ) ;
#67329=CARTESIAN_POINT ( 'NONE',  ( 21.15000000000005542, 74.16448838626247664, -47.52760213295649550 ) ) ;
#67375=DIRECTION ( 'NONE',  ( 0.000000000000000000, 0.000000000000000000, -1.000000000000000000 ) ) ;
#67434=DIRECTION ( 'NONE',  ( 0.000000000000000000, 0.000000000000000000, -1.000000000000000000 ) ) ;
#67450=EDGE_CURVE ( 'NONE', #22457, #189336, #82157, .T. ) ;
#67497=VECTOR ( 'NONE', #78363, 1000.000000000000114 ) ;
#67532=EDGE_LOOP ( 'NONE', ( #73636, #17084, #21288, #93338 ) ) ;
#67560=ADVANCED_FACE ( 'NONE', ( #123157 ), #244489, .T. ) ;
#67678=ORIENTED_EDGE ( 'NONE', *, *, #49272, .F. ) ;
#67745=AXIS2_PLACEMENT_3D ( 'NONE', #176437, #255896, #77304 ) ;
#67801=ORIENTED_EDGE ( 'NONE', *, *, #162331, .T. ) ;
#67834=CARTESIAN_POINT ( 'NONE',  ( -21.14999999999994174, 84.00000000001119815, -37.18565239344504647 ) ) ;
#67848=EDGE_CURVE ( 'NONE', #116279, #111921, #31793, .T. ) ;
#67883=EDGE_CURVE ( 'NONE', #30427, #60636, #135973, .T. ) ;
#67891=CARTESIAN_POINT ( 'NONE',  ( -23.39999999999994529, 87.50449464844290048, -34.18759587077607165 ) ) ;
#67896=ORIENTED_EDGE ( 'NONE', *, *, #176658, .F. ) ;
#67908=AXIS2_PLACEMENT_3D ( 'NONE', #65710, #86527, #46143 ) ;
#67917=EDGE_LOOP ( 'NONE', ( #247589, #5523, #79649, #4173 ) ) ;
#67970=DIRECTION ( 'NONE',  ( 1.000000000000000000, -0.000000000000000000, -0.000000000000000000 ) ) ;
#67987=EDGE_CURVE ( 'NONE', #118259, #133767, #43322, .T. ) ;
#68006=ORIENTED_EDGE ( 'NONE', *, *, #169123, .F. ) ;
#68020=CIRCLE ( 'NONE', #34718, 0.09999999999999939493 ) ;
#68024=DIRECTION ( 'NONE',  ( 0.000000000000000000, 0.000000000000000000, 1.000000000000000000 ) ) ;
#68062=VECTOR ( 'NONE', #208955, 1000.000000000000114 ) ;
#68170=VERTEX_POINT ( 'NONE', #73180 ) ;
#68232=AXIS2_PLACEMENT_3D ( 'NONE', #242819, #122892, #144989 ) ;
#68325=DIRECTION ( 'NONE',  ( 0.000000000000000000, 0.000000000000000000, 1.000000000000000000 ) ) ;
#68335=VERTEX_POINT ( 'NONE', #199535 ) ;
#68350=EDGE_CURVE ( 'NONE', #77791, #34933, #18304, .T. ) ;
#68381=DIRECTION ( 'NONE',  ( -2.889348024582214003E-16, -0.1332476588733650935, -0.9910827722268042983 ) ) ;
#68382=DIRECTION ( 'NONE',  ( 1.000000000000000000, -0.000000000000000000, -0.000000000000000000 ) ) ;
#68384=AXIS2_PLACEMENT_3D ( 'NONE', #154069, #57466, #194456 ) ;
#68392=DIRECTION ( 'NONE',  ( -0.000000000000000000, -1.000000000000000000, 0.000000000000000000 ) ) ;
#68393=DIRECTION ( 'NONE',  ( 0.000000000000000000, 0.1332476588733589040, -0.9910827722268049644 ) ) ;
#68462=DIRECTION ( 'NONE',  ( 0.000000000000000000, -0.9889818879709272315, -0.1480365673253073999 ) ) ;
#68599=TOROIDAL_SURFACE ( 'NONE', #130942, 0.2000000000000000111, 0.1000000000000000056 ) ;
#68617=DIRECTION ( 'NONE',  ( 0.000000000000000000, 0.000000000000000000, 1.000000000000000000 ) ) ;
#68635=DIRECTION ( 'NONE',  ( 0.000000000000000000, 0.000000000000000000, 1.000000000000000000 ) ) ;
#68638=EDGE_CURVE ( 'NONE', #23353, #74847, #174562, .T. ) ;
#68647=EDGE_CURVE ( 'NONE', #216962, #184062, #109376, .T. ) ;
#68652=ADVANCED_FACE ( 'NONE', ( #53279 ), #132825, .F. ) ;
#68672=CARTESIAN_POINT ( 'NONE',  ( 21.15000000000005542, 77.83551161375991967, -47.52760213295649550 ) ) ;
#68683=AXIS2_PLACEMENT_3D ( 'NONE', #233875, #155657, #172670 ) ;
#68703=DIRECTION ( 'NONE',  ( 0.000000000000000000, 0.000000000000000000, 1.000000000000000000 ) ) ;
#68773=DIRECTION ( 'NONE',  ( 0.000000000000000000, 0.000000000000000000, 1.000000000000000000 ) ) ;
#68832=EDGE_CURVE ( 'NONE', #201062, #12214, #87292, .T. ) ;
#68875=EDGE_LOOP ( 'NONE', ( #8784, #224060, #98636 ) ) ;
#68883=DIRECTION ( 'NONE',  ( 0.000000000000000000, 0.000000000000000000, 1.000000000000000000 ) ) ;
#68912=EDGE_CURVE ( 'NONE', #1657, #230912, #158262, .T. ) ;
#68922=DIRECTION ( 'NONE',  ( -1.000000000000000000, -3.439547145395919517E-14, 4.624352451196577991E-15 ) ) ;
#68940=AXIS2_PLACEMENT_3D ( 'NONE', #225796, #129295, #65458 ) ;
#68980=AXIS2_PLACEMENT_3D ( 'NONE', #155977, #219760, #198921 ) ;
#69023=ORIENTED_EDGE ( 'NONE', *, *, #253975, .T. ) ;
#69076=ORIENTED_EDGE ( 'NONE', *, *, #158548, .T. ) ;
#69111=ORIENTED_EDGE ( 'NONE', *, *, #121247, .T. ) ;
#69129=VERTEX_POINT ( 'NONE', #59338 ) ;
#69133=LINE ( 'NONE', #148664, #115074 ) ;
#69143=DIRECTION ( 'NONE',  ( 0.000000000000000000, 1.000000000000000000, 0.000000000000000000 ) ) ;
#69289=AXIS2_PLACEMENT_3D ( 'NONE', #103942, #204340, #165228 ) ;
#69307=ORIENTED_EDGE ( 'NONE', *, *, #206989, .F. ) ;
#69334=CARTESIAN_POINT ( 'NONE',  ( 23.40000000000005187, 74.94272479589878344, -8.023107484524793165 ) ) ;
#69337=EDGE_CURVE ( 'NONE', #9389, #74847, #89053, .T. ) ;
#69370=DIRECTION ( 'NONE',  ( 0.000000000000000000, 0.000000000000000000, -1.000000000000000000 ) ) ;
#69416=ORIENTED_EDGE ( 'NONE', *, *, #68647, .F. ) ;
#69425=LINE ( 'NONE', #207653, #118055 ) ;
#69428=ADVANCED_FACE ( 'NONE', ( #176162 ), #133164, .F. ) ;
#69436=CARTESIAN_POINT ( 'NONE',  ( -21.04999999999994387, 79.78873604695631627, -7.297728304630792806 ) ) ;
#69475=CIRCLE ( 'NONE', #215201, 4.049999999999998046 ) ;
#69476=ORIENTED_EDGE ( 'NONE', *, *, #246668, .T. ) ;
#69489=FACE_OUTER_BOUND ( 'NONE', #39197, .T. ) ;
#69506=DIRECTION ( 'NONE',  ( 0.000000000000000000, -1.000000000000000000, 0.000000000000000000 ) ) ;
#69512=CARTESIAN_POINT ( 'NONE',  ( -21.04999999999994387, 64.35000000001120668, -5.923107484524795296 ) ) ;
#69526=ADVANCED_FACE ( 'NONE', ( #101699 ), #68599, .T. ) ;
#69558=DIRECTION ( 'NONE',  ( 1.000000000000000000, 0.000000000000000000, 0.000000000000000000 ) ) ;
#69595=FACE_OUTER_BOUND ( 'NONE', #135083, .T. ) ;
#69639=AXIS2_PLACEMENT_3D ( 'NONE', #31302, #93792, #91246 ) ;
#69678=CARTESIAN_POINT ( 'NONE',  ( -20.94999999999994600, 87.75000000001119815, -5.923107484524795296 ) ) ;
#69701=TOROIDAL_SURFACE ( 'NONE', #165372, 0.2000000000000000111, 0.1000000000000000056 ) ;
#69723=CARTESIAN_POINT ( 'NONE',  ( -20.94999999999994600, 66.15000000001120384, -4.623107484524796362 ) ) ;
#69764=AXIS2_PLACEMENT_3D ( 'NONE', #86290, #224538, #167177 ) ;
#69811=AXIS2_PLACEMENT_3D ( 'NONE', #246999, #68382, #147924 ) ;
#69827=ORIENTED_EDGE ( 'NONE', *, *, #64552, .T. ) ;
#69836=DIRECTION ( 'NONE',  ( -1.000000000000000000, 0.000000000000000000, -0.000000000000000000 ) ) ;
#69842=COLOUR_RGB ( '', 0.08235294, 0.09019608, 0.10196078) ;
#69885=CARTESIAN_POINT ( 'NONE',  ( 11.60000000000006182, 66.35000000001119247, -23.62310748452479103 ) ) ;
#69937=CIRCLE ( 'NONE', #107323, 0.1999999999999987899 ) ;
#69938=AXIS2_PLACEMENT_3D ( 'NONE', #80392, #41333, #200385 ) ;
#69947=FACE_OUTER_BOUND ( 'NONE', #157673, .T. ) ;
#70025=CARTESIAN_POINT ( 'NONE',  ( 5.900000000000060751, 64.25000000001119815, -21.92310748452479174 ) ) ;
#70029=DIRECTION ( 'NONE',  ( -0.000000000000000000, 1.000000000000000000, -0.000000000000000000 ) ) ;
#70031=CARTESIAN_POINT ( 'NONE',  ( 20.95000000000005258, 65.25000000001119815, -4.423107484524790856 ) ) ;
#70066=ADVANCED_FACE ( 'NONE', ( #222627 ), #218587, .T. ) ;
#70090=EDGE_LOOP ( 'NONE', ( #127446, #117218, #235479, #130164 ) ) ;
#70093=EDGE_LOOP ( 'NONE', ( #170773, #186986, #8441, #90342 ) ) ;
#70115=ADVANCED_FACE ( 'NONE', ( #187393 ), #166562, .F. ) ;
#70127=AXIS2_PLACEMENT_3D ( 'NONE', #90083, #246596, #147507 ) ;
#70175=VECTOR ( 'NONE', #84951, 1000.000000000000000 ) ;
#70202=ADVANCED_FACE ( 'NONE', ( #209501 ), #114751, .T. ) ;
#70216=CARTESIAN_POINT ( 'NONE',  ( 13.40000000000005898, 64.35000000001120668, -23.62310748452479103 ) ) ;
#70277=LINE ( 'NONE', #136283, #692 ) ;
#70292=ADVANCED_FACE ( 'NONE', ( #76392 ), #60678, .T. ) ;
#70297=EDGE_LOOP ( 'NONE', ( #209590, #79354, #23600, #76546 ) ) ;
#70329=DIRECTION ( 'NONE',  ( 0.000000000000000000, 0.000000000000000000, -1.000000000000000000 ) ) ;
#70475=AXIS2_PLACEMENT_3D ( 'NONE', #146299, #49772, #126744 ) ;
#70478=ORIENTED_EDGE ( 'NONE', *, *, #200564, .T. ) ;
#70480=EDGE_CURVE ( 'NONE', #15261, #135372, #14876, .T. ) ;
#70501=DIRECTION ( 'NONE',  ( 1.000000000000000000, 0.000000000000000000, 0.000000000000000000 ) ) ;
#70517=ADVANCED_FACE ( 'NONE', ( #190949 ), #231351, .F. ) ;
#70539=CARTESIAN_POINT ( 'NONE',  ( 21.15000000000005187, 76.00000000001119815, -36.02310748452479316 ) ) ;
#70572=FACE_OUTER_BOUND ( 'NONE', #77109, .T. ) ;
#70576=FACE_OUTER_BOUND ( 'NONE', #126309, .T. ) ;
#70589=AXIS2_PLACEMENT_3D ( 'NONE', #59798, #115961, #58520 ) ;
#70614=FACE_OUTER_BOUND ( 'NONE', #191922, .T. ) ;
#70775=CARTESIAN_POINT ( 'NONE',  ( -21.04999999999994387, 76.00000000001119815, -31.87310748452479459 ) ) ;
#70972=ORIENTED_EDGE ( 'NONE', *, *, #236881, .F. ) ;
#70973=DIRECTION ( 'NONE',  ( 0.000000000000000000, -1.000000000000000000, 0.000000000000000000 ) ) ;
#71003=DIRECTION ( 'NONE',  ( 0.000000000000000000, -1.000000000000000000, 0.000000000000000000 ) ) ;
#71026=CARTESIAN_POINT ( 'NONE',  ( -23.39999999999994529, 77.83551161375991967, -47.52760213295649550 ) ) ;
#71073=EDGE_LOOP ( 'NONE', ( #57313, #69416, #238141, #27125 ) ) ;
#71125=EDGE_CURVE ( 'NONE', #224041, #194487, #223932, .T. ) ;
#71174=DIRECTION ( 'NONE',  ( 0.000000000000000000, 0.000000000000000000, 1.000000000000000000 ) ) ;
#71175=AXIS2_PLACEMENT_3D ( 'NONE', #197070, #231099, #18448 ) ;
#71196=EDGE_CURVE ( 'NONE', #114288, #158981, #256507, .T. ) ;
#71266=CARTESIAN_POINT ( 'NONE',  ( 11.60000000000006004, 67.75000000001118394, -23.62310748452479103 ) ) ;
#71308=ORIENTED_EDGE ( 'NONE', *, *, #142536, .F. ) ;
#71355=DIRECTION ( 'NONE',  ( 1.000000000000000000, -0.000000000000000000, -0.000000000000000000 ) ) ;
#71371=CARTESIAN_POINT ( 'NONE',  ( 23.40000000000005542, 74.16448838626247664, -47.52760213295649550 ) ) ;
#71374=ADVANCED_FACE ( 'NONE', ( #179398 ), #34769, .T. ) ;
#71431=CARTESIAN_POINT ( 'NONE',  ( -23.49999999999994316, 79.88763423575340994, -7.282924647898262549 ) ) ;
#71465=CARTESIAN_POINT ( 'NONE',  ( 21.05000000000005400, 67.65000000001118963, -25.06452884076210452 ) ) ;
#71480=EDGE_CURVE ( 'NONE', #256542, #183369, #40325, .T. ) ;
#71497=LINE ( 'NONE', #14081, #228141 ) ;
#71572=ADVANCED_FACE ( 'NONE', ( #205342 ), #207955, .F. ) ;
#71613=DIRECTION ( 'NONE',  ( 0.000000000000000000, 1.000000000000000000, 0.000000000000000000 ) ) ;
#71643=ORIENTED_EDGE ( 'NONE', *, *, #102474, .T. ) ;
#71670=AXIS2_PLACEMENT_3D ( 'NONE', #143259, #37770, #196806 ) ;
#71672=ORIENTED_EDGE ( 'NONE', *, *, #172597, .T. ) ;
#71688=CARTESIAN_POINT ( 'NONE',  ( 21.15000000000005542, 87.50449464844290048, -34.18759587077607165 ) ) ;
#71694=DIRECTION ( 'NONE',  ( -0.000000000000000000, -1.000000000000000000, -0.000000000000000000 ) ) ;
#71753=ADVANCED_FACE ( 'NONE', ( #77392 ), #186219, .T. ) ;
#71779=VECTOR ( 'NONE', #96796, 1000.000000000000000 ) ;
#71787=ADVANCED_FACE ( 'NONE', ( #213061 ), #69701, .T. ) ;
#71812=ORIENTED_EDGE ( 'NONE', *, *, #168388, .F. ) ;
#71879=CARTESIAN_POINT ( 'NONE',  ( 20.95000000000005258, 64.35000000001119247, -5.923107484524795296 ) ) ;
#71893=ORIENTED_EDGE ( 'NONE', *, *, #134753, .T. ) ;
#71954=LINE ( 'NONE', #151508, #18223 ) ;
#71966=EDGE_LOOP ( 'NONE', ( #85606, #44228, #248628 ) ) ;
#71973=CYLINDRICAL_SURFACE ( 'NONE', #153585, 0.09999999999999939493 ) ;
#72035=EDGE_CURVE ( 'NONE', #122419, #253828, #66838, .T. ) ;
#72086=CARTESIAN_POINT ( 'NONE',  ( 23.40000000000005187, 76.00000000001119815, -31.87310748452479459 ) ) ;
#72110=AXIS2_PLACEMENT_3D ( 'NONE', #16872, #96369, #117244 ) ;
#72196=DIRECTION ( 'NONE',  ( -1.000000000000000000, -0.000000000000000000, -0.000000000000000000 ) ) ;
#72218=AXIS2_PLACEMENT_3D ( 'NONE', #238089, #218510, #58155 ) ;
#72255=DIRECTION ( 'NONE',  ( 0.000000000000000000, 0.9910827722268049644, 0.1332476588733589318 ) ) ;
#72367=AXIS2_PLACEMENT_3D ( 'NONE', #245286, #189156, #66641 ) ;
#72437=CARTESIAN_POINT ( 'NONE',  ( 23.40000000000005187, 87.50449464844290048, -37.85861909827351468 ) ) ;
#72447=DIRECTION ( 'NONE',  ( -0.000000000000000000, 1.000000000000000000, -0.000000000000000000 ) ) ;
#72459=DIRECTION ( 'NONE',  ( 0.000000000000000000, 1.000000000000000000, 0.000000000000000000 ) ) ;
#72502=CARTESIAN_POINT ( 'NONE',  ( -21.14999999999994174, 84.00000000001119815, -34.86056257560453986 ) ) ;
#72506=ORIENTED_EDGE ( 'NONE', *, *, #112733, .T. ) ;
#72525=CARTESIAN_POINT ( 'NONE',  ( 13.40000000000005898, 67.75000000001118394, -21.02310748452479316 ) ) ;
#72532=AXIS2_PLACEMENT_3D ( 'NONE', #17795, #253841, #210880 ) ;
#72554=CIRCLE ( 'NONE', #118344, 0.09999999999999530098 ) ;
#72582=ORIENTED_EDGE ( 'NONE', *, *, #49799, .F. ) ;
#72583=TOROIDAL_SURFACE ( 'NONE', #138595, 0.2000000000000000111, 0.1000000000000000056 ) ;
#72627=VECTOR ( 'NONE', #31055, 1000.000000000000114 ) ;
#72653=CIRCLE ( 'NONE', #139242, 5.000000000000000888 ) ;
#72675=LINE ( 'NONE', #174364, #176230 ) ;
#72723=EDGE_CURVE ( 'NONE', #130445, #224041, #181735, .T. ) ;
#72731=CARTESIAN_POINT ( 'NONE',  ( 21.05000000000005400, 73.94408376456904364, -49.16694968567509250 ) ) ;
#72746=AXIS2_PLACEMENT_3D ( 'NONE', #202991, #81728, #40109 ) ;
#72752=DIRECTION ( 'NONE',  ( 0.000000000000000000, 0.000000000000000000, 1.000000000000000000 ) ) ;
#72791=EDGE_LOOP ( 'NONE', ( #153003, #79241, #52437, #30197 ) ) ;
#72861=DIRECTION ( 'NONE',  ( 1.000000000000000000, -0.000000000000000000, -0.000000000000000000 ) ) ;
#72903=CARTESIAN_POINT ( 'NONE',  ( -20.94999999999994600, 87.75000000001119815, -4.623107484524796362 ) ) ;
#72982=EDGE_CURVE ( 'NONE', #154033, #135761, #252815, .T. ) ;
#72996=FACE_OUTER_BOUND ( 'NONE', #233762, .T. ) ;
#73015=AXIS2_PLACEMENT_3D ( 'NONE', #209121, #229975, #250815 ) ;
#73069=CARTESIAN_POINT ( 'NONE',  ( -21.14999999999994174, 83.97335046823651794, -34.66234602115918051 ) ) ;
#73109=VERTEX_POINT ( 'NONE', #186841 ) ;
#73180=CARTESIAN_POINT ( 'NONE',  ( -23.49999999999994316, 74.94272479589878344, -3.123107484524795474 ) ) ;
#73200=ORIENTED_EDGE ( 'NONE', *, *, #239506, .T. ) ;
#73212=DIRECTION ( 'NONE',  ( 1.000000000000000000, -0.000000000000000000, -0.000000000000000000 ) ) ;
#73233=FACE_OUTER_BOUND ( 'NONE', #241154, .T. ) ;
#73316=EDGE_CURVE ( 'NONE', #39283, #23611, #119756, .T. ) ;
#73349=DIRECTION ( 'NONE',  ( 1.000000000000000000, -0.000000000000000000, 0.000000000000000000 ) ) ;
#73381=AXIS2_PLACEMENT_3D ( 'NONE', #250283, #191630, #172067 ) ;
#73412=EDGE_LOOP ( 'NONE', ( #79918, #73569, #127773, #196208 ) ) ;
#73453=ORIENTED_EDGE ( 'NONE', *, *, #190307, .T. ) ;
#73536=EDGE_CURVE ( 'NONE', #167673, #209133, #55971, .T. ) ;
#73558=EDGE_CURVE ( 'NONE', #26051, #107789, #58543, .T. ) ;
#73569=ORIENTED_EDGE ( 'NONE', *, *, #235317, .F. ) ;
#73628=LINE ( 'NONE', #153179, #224310 ) ;
#73636=ORIENTED_EDGE ( 'NONE', *, *, #73316, .T. ) ;
#73641=DIRECTION ( 'NONE',  ( 0.000000000000000000, 0.000000000000000000, -1.000000000000000000 ) ) ;
#73651=VERTEX_POINT ( 'NONE', #239774 ) ;
#73664=CARTESIAN_POINT ( 'NONE',  ( 11.60000000000006182, 67.65000000001118963, -16.98168612828748891 ) ) ;
#73694=DIRECTION ( 'NONE',  ( -0.000000000000000000, -0.9910827722268039652, 0.1332476588733665090 ) ) ;
#73776=DIRECTION ( 'NONE',  ( 1.000000000000000000, 0.000000000000000000, -0.000000000000000000 ) ) ;
#73914=ORIENTED_EDGE ( 'NONE', *, *, #146087, .T. ) ;
#73919=ORIENTED_EDGE ( 'NONE', *, *, #76213, .T. ) ;
#73922=AXIS2_PLACEMENT_3D ( 'NONE', #203186, #243599, #226585 ) ;
#73940=LINE ( 'NONE', #33546, #75824 ) ;
#73962=AXIS2_PLACEMENT_3D ( 'NONE', #205492, #223767, #85518 ) ;
#73965=CARTESIAN_POINT ( 'NONE',  ( -21.04999999999994387, 66.15000000001114699, -51.02310748452479316 ) ) ;
#74072=DIRECTION ( 'NONE',  ( -1.000000000000000000, 0.000000000000000000, -0.000000000000000000 ) ) ;
#74087=CARTESIAN_POINT ( 'NONE',  ( -23.49999999999994316, 76.00000000001119815, -36.02310748452479316 ) ) ;
#74163=DIRECTION ( 'NONE',  ( -1.000000000000000000, 0.000000000000000000, 0.000000000000000000 ) ) ;
#74170=VERTEX_POINT ( 'NONE', #111186 ) ;
#74182=EDGE_CURVE ( 'NONE', #251797, #183226, #253381, .T. ) ;
#74223=DIRECTION ( 'NONE',  ( 0.000000000000000000, 0.000000000000000000, 1.000000000000000000 ) ) ;
#74224=DIRECTION ( 'NONE',  ( 0.000000000000000000, 0.000000000000000000, 1.000000000000000000 ) ) ;
#74274=ORIENTED_EDGE ( 'NONE', *, *, #203888, .T. ) ;
#74353=FACE_OUTER_BOUND ( 'NONE', #78067, .T. ) ;
#74426=CARTESIAN_POINT ( 'NONE',  ( -21.04999999999994387, 73.58898499266442172, -51.80813886865390572 ) ) ;
#74427=DIRECTION ( 'NONE',  ( 0.000000000000000000, 0.000000000000000000, -1.000000000000000000 ) ) ;
#74434=EDGE_CURVE ( 'NONE', #64265, #104499, #120339, .T. ) ;
#74546=CARTESIAN_POINT ( 'NONE',  ( 20.95000000000005258, 65.35000000001120668, -3.023107484524792277 ) ) ;
#74569=ORIENTED_EDGE ( 'NONE', *, *, #138506, .F. ) ;
#74572=CARTESIAN_POINT ( 'NONE',  ( 20.95000000000005258, 64.25000000001119815, -5.923107484524795296 ) ) ;
#74594=DIRECTION ( 'NONE',  ( 0.000000000000000000, -0.1332476588733448597, 0.9910827722268067408 ) ) ;
#74649=ORIENTED_EDGE ( 'NONE', *, *, #229977, .T. ) ;
#74660=DIRECTION ( 'NONE',  ( 1.000000000000000000, -0.000000000000000000, 0.000000000000000000 ) ) ;
#74675=VECTOR ( 'NONE', #159414, 1000.000000000000000 ) ;
#74678=DIRECTION ( 'NONE',  ( 1.000000000000000000, 0.000000000000000000, 0.000000000000000000 ) ) ;
#74695=DIRECTION ( 'NONE',  ( 0.000000000000000000, 0.000000000000000000, 1.000000000000000000 ) ) ;
#74714=ORIENTED_EDGE ( 'NONE', *, *, #195472, .T. ) ;
#74742=ORIENTED_EDGE ( 'NONE', *, *, #140601, .T. ) ;
#74765=ADVANCED_FACE ( 'NONE', ( #35372 ), #170225, .T. ) ;
#74768=DIRECTION ( 'NONE',  ( -1.000000000000000000, 0.000000000000000000, 0.000000000000000000 ) ) ;
#74785=CARTESIAN_POINT ( 'NONE',  ( 23.40000000000005187, 77.16254490893143725, -44.02310748452479316 ) ) ;
#74787=EDGE_CURVE ( 'NONE', #65513, #84546, #237000, .T. ) ;
#74847=VERTEX_POINT ( 'NONE', #159157 ) ;
#74870=LINE ( 'NONE', #176518, #41224 ) ;
#74886=VERTEX_POINT ( 'NONE', #46862 ) ;
#74977=CARTESIAN_POINT ( 'NONE',  ( 21.05000000000005400, 64.35000000001120668, -30.12310748452479103 ) ) ;
#75040=ORIENTED_EDGE ( 'NONE', *, *, #244501, .F. ) ;
#75088=VERTEX_POINT ( 'NONE', #96258 ) ;
#75151=AXIS2_PLACEMENT_3D ( 'NONE', #247863, #208754, #167079 ) ;
#75204=CARTESIAN_POINT ( 'NONE',  ( -0.8999999999999438449, 67.75000000001118394, -5.981686128287480919 ) ) ;
#75211=DIRECTION ( 'NONE',  ( 0.000000000000000000, 0.9889818879709272315, 0.1480365673253073999 ) ) ;
#75218=AXIS2_PLACEMENT_3D ( 'NONE', #221601, #43003, #202073 ) ;
#75283=CIRCLE ( 'NONE', #12936, 0.1000000000000028644 ) ;
#75289=DIRECTION ( 'NONE',  ( -0.000000000000000000, 0.1332476588733589318, 0.9910827722268049644 ) ) ;
#75426=ORIENTED_EDGE ( 'NONE', *, *, #242302, .F. ) ;
#75435=CARTESIAN_POINT ( 'NONE',  ( 20.95000000000005258, 66.25000000001119815, -4.523107484524794053 ) ) ;
#75466=DIRECTION ( 'NONE',  ( 0.000000000000000000, 0.1332476588733589318, 0.9910827722268050755 ) ) ;
#75490=DIRECTION ( 'NONE',  ( 0.000000000000000000, 0.9875102702516471709, 0.1575546449569757979 ) ) ;
#75514=DIRECTION ( 'NONE',  ( 1.000000000000000000, 0.000000000000000000, 0.000000000000000000 ) ) ;
#75557=EDGE_CURVE ( 'NONE', #80255, #257282, #254092, .T. ) ;
#75636=EDGE_CURVE ( 'NONE', #245973, #50347, #12524, .T. ) ;
#75700=ORIENTED_EDGE ( 'NONE', *, *, #218992, .T. ) ;
#75727=DIRECTION ( 'NONE',  ( -0.000000000000000000, 1.000000000000000000, -0.000000000000000000 ) ) ;
#75764=VECTOR ( 'NONE', #72196, 1000.000000000000000 ) ;
#75799=ORIENTED_EDGE ( 'NONE', *, *, #79816, .F. ) ;
#75824=VECTOR ( 'NONE', #153500, 1000.000000000000000 ) ;
#75827=CARTESIAN_POINT ( 'NONE',  ( 21.15000000000005542, 74.16448838626247664, -47.52760213295649550 ) ) ;
#75839=CARTESIAN_POINT ( 'NONE',  ( 21.05000000000005400, 64.25000000001119815, -5.923107484524795296 ) ) ;
#75854=VERTEX_POINT ( 'NONE', #74546 ) ;
#75890=ORIENTED_EDGE ( 'NONE', *, *, #76213, .F. ) ;
#75955=CYLINDRICAL_SURFACE ( 'NONE', #2911, 0.1000000000000028644 ) ;
#76016=ORIENTED_EDGE ( 'NONE', *, *, #3443, .F. ) ;
#76020=CARTESIAN_POINT ( 'NONE',  ( -21.14999999999994174, 65.15000000001120384, -3.123107484524795474 ) ) ;
#76077=FACE_OUTER_BOUND ( 'NONE', #66074, .T. ) ;
#76098=EDGE_LOOP ( 'NONE', ( #242276, #192070, #246214, #108990 ) ) ;
#76152=DIRECTION ( 'NONE',  ( -1.000000000000000000, -0.000000000000000000, -0.000000000000000000 ) ) ;
#76213=EDGE_CURVE ( 'NONE', #30110, #59493, #235818, .T. ) ;
#76318=CARTESIAN_POINT ( 'NONE',  ( -23.49999999999994316, 83.97335046823651794, -37.38386894789040582 ) ) ;
#76387=CIRCLE ( 'NONE', #184727, 0.09999999999999939493 ) ;
#76392=FACE_OUTER_BOUND ( 'NONE', #155497, .T. ) ;
#76396=ORIENTED_EDGE ( 'NONE', *, *, #93795, .F. ) ;
#76412=VECTOR ( 'NONE', #245509, 1000.000000000000000 ) ;
#76432=VERTEX_POINT ( 'NONE', #161445 ) ;
#76436=ORIENTED_EDGE ( 'NONE', *, *, #255338, .F. ) ;
#76437=CIRCLE ( 'NONE', #226445, 3.970710678118656300 ) ;
#76483=CIRCLE ( 'NONE', #51523, 0.09999999999999939493 ) ;
#76546=ORIENTED_EDGE ( 'NONE', *, *, #168294, .T. ) ;
#76593=CARTESIAN_POINT ( 'NONE',  ( -21.04999999999994387, 67.65000000001118963, -25.49719488170504533 ) ) ;
#76604=AXIS2_PLACEMENT_3D ( 'NONE', #138076, #217603, #40315 ) ;
#76629=AXIS2_PLACEMENT_3D ( 'NONE', #66210, #145724, #27111 ) ;
#76630=ADVANCED_FACE ( 'NONE', ( #59404 ), #137677, .T. ) ;
#76634=CIRCLE ( 'NONE', #101733, 0.1999999999999987899 ) ;
#76753=EDGE_CURVE ( 'NONE', #194487, #195803, #167211, .T. ) ;
#76794=CARTESIAN_POINT ( 'NONE',  ( 11.60000000000006182, 64.35000000001120668, -18.42310748452479530 ) ) ;
#76844=ORIENTED_EDGE ( 'NONE', *, *, #138665, .T. ) ;
#76857=CARTESIAN_POINT ( 'NONE',  ( -20.94999999999994600, 65.35000000001120668, -3.123107484524795474 ) ) ;
#76861=AXIS2_PLACEMENT_3D ( 'NONE', #229998, #50075, #173931 ) ;
#76908=DIRECTION ( 'NONE',  ( 0.000000000000000000, 0.000000000000000000, -1.000000000000000000 ) ) ;
#76948=DIRECTION ( 'NONE',  ( 1.000000000000000000, 0.000000000000000000, 0.000000000000000000 ) ) ;
#76959=CARTESIAN_POINT ( 'NONE',  ( -21.14999999999994174, 74.83745509109094485, -44.02310748452479316 ) ) ;
#77036=EDGE_CURVE ( 'NONE', #297, #239496, #213075, .T. ) ;
#77109=EDGE_LOOP ( 'NONE', ( #124215, #129076, #162968, #202820 ) ) ;
#77145=FACE_OUTER_BOUND ( 'NONE', #58780, .T. ) ;
#77189=EDGE_LOOP ( 'NONE', ( #218405, #187459, #256069, #40031 ) ) ;
#77210=EDGE_CURVE ( 'NONE', #88201, #104499, #148649, .T. ) ;
#77238=LINE ( 'NONE', #201051, #172304 ) ;
#77273=EDGE_CURVE ( 'NONE', #33512, #223504, #134190, .T. ) ;
#77304=DIRECTION ( 'NONE',  ( 0.000000000000000000, 0.000000000000000000, 1.000000000000000000 ) ) ;
#77392=FACE_OUTER_BOUND ( 'NONE', #118528, .T. ) ;
#77396=ORIENTED_EDGE ( 'NONE', *, *, #244498, .T. ) ;
#77414=DIRECTION ( 'NONE',  ( 0.000000000000000000, 0.000000000000000000, -1.000000000000000000 ) ) ;
#77421=CYLINDRICAL_SURFACE ( 'NONE', #52205, 0.09999999999999939493 ) ;
#77442=ORIENTED_EDGE ( 'NONE', *, *, #233362, .T. ) ;
#77537=DIRECTION ( 'NONE',  ( 1.000000000000000000, -0.000000000000000000, -0.000000000000000000 ) ) ;
#77548=AXIS2_PLACEMENT_3D ( 'NONE', #219250, #83568, #61477 ) ;
#77549=LINE ( 'NONE', #198800, #204993 ) ;
#77552=ORIENTED_EDGE ( 'NONE', *, *, #148924, .F. ) ;
#77587=AXIS2_PLACEMENT_3D ( 'NONE', #61234, #179918, #195634 ) ;
#77610=PLANE ( 'NONE',  #175161 ) ;
#77682=AXIS2_PLACEMENT_3D ( 'NONE', #175058, #69506, #149040 ) ;
#77710=EDGE_CURVE ( 'NONE', #245973, #63115, #198999, .T. ) ;
#77713=CARTESIAN_POINT ( 'NONE',  ( -13.39999999999994529, 64.35000000001120668, -21.02310748452479316 ) ) ;
#77720=DIRECTION ( 'NONE',  ( 0.000000000000000000, 0.000000000000000000, 1.000000000000000000 ) ) ;
#77738=ORIENTED_EDGE ( 'NONE', *, *, #235317, .T. ) ;
#77785=ORIENTED_EDGE ( 'NONE', *, *, #5534, .F. ) ;
#77787=VERTEX_POINT ( 'NONE', #239416 ) ;
#77791=VERTEX_POINT ( 'NONE', #60752 ) ;
#77833=VECTOR ( 'NONE', #132039, 1000.000000000000000 ) ;
#77918=DIRECTION ( 'NONE',  ( 1.000000000000000000, -0.000000000000000000, -0.000000000000000000 ) ) ;
#77961=EDGE_CURVE ( 'NONE', #132923, #88201, #113461, .T. ) ;
#77967=VECTOR ( 'NONE', #27019, 1000.000000000000114 ) ;
#78028=VECTOR ( 'NONE', #152883, 1000.000000000000114 ) ;
#78067=EDGE_LOOP ( 'NONE', ( #21166, #186241, #1721 ) ) ;
#78097=CIRCLE ( 'NONE', #223831, 0.1000000000000021844 ) ;
#78119=ORIENTED_EDGE ( 'NONE', *, *, #20749, .T. ) ;
#78192=EDGE_CURVE ( 'NONE', #106794, #211140, #97028, .T. ) ;
#78225=ORIENTED_EDGE ( 'NONE', *, *, #230430, .T. ) ;
#78228=CARTESIAN_POINT ( 'NONE',  ( -21.14999999999994174, 77.16254490893143725, -44.02310748452479316 ) ) ;
#78263=ORIENTED_EDGE ( 'NONE', *, *, #205981, .T. ) ;
#78269=CARTESIAN_POINT ( 'NONE',  ( 20.95000000000005258, 65.35000000001120668, -4.423107484524790856 ) ) ;
#78273=ADVANCED_FACE ( 'NONE', ( #245550 ), #138725, .T. ) ;
#78292=AXIS2_PLACEMENT_3D ( 'NONE', #181553, #240240, #4169 ) ;
#78299=SURFACE_SIDE_STYLE ('',( #123877 ) ) ;
#78363=DIRECTION ( 'NONE',  ( -0.000000000000000000, 0.1480365673253065117, -0.9889818879709273425 ) ) ;
#78503=EDGE_CURVE ( 'NONE', #179524, #56891, #126478, .T. ) ;
#78514=EDGE_CURVE ( 'NONE', #97476, #80255, #38073, .T. ) ;
#78538=CARTESIAN_POINT ( 'NONE',  ( 21.05000000000005400, 65.35000000001120668, -3.023107484524792277 ) ) ;
#78555=DIRECTION ( 'NONE',  ( -0.000000000000000000, -0.9910827722268049644, -0.1332476588733589318 ) ) ;
#78640=EDGE_LOOP ( 'NONE', ( #23590, #253824, #85168 ) ) ;
#78698=CIRCLE ( 'NONE', #3897, 0.1000000000000032391 ) ;
#78707=DIRECTION ( 'NONE',  ( 1.000000000000000000, -0.000000000000000000, -0.000000000000000000 ) ) ;
#78727=EDGE_CURVE ( 'NONE', #23626, #224235, #76387, .T. ) ;
#78760=AXIS2_PLACEMENT_3D ( 'NONE', #244252, #66913, #203851 ) ;
#78786=CARTESIAN_POINT ( 'NONE',  ( 21.15000000000005542, 74.83745509109094485, -43.82310748452479743 ) ) ;
#78829=CARTESIAN_POINT ( 'NONE',  ( -23.39999999999994529, 77.85126707825561709, -47.62635315998165453 ) ) ;
#78874=DIRECTION ( 'NONE',  ( -0.000000000000000000, 1.000000000000000000, -0.000000000000000000 ) ) ;
#78938=EDGE_CURVE ( 'NONE', #53673, #98456, #202458, .T. ) ;
#79000=SPHERICAL_SURFACE ( 'NONE', #123452, 0.1000000000000000056 ) ;
#79004=SPHERICAL_SURFACE ( 'NONE', #196821, 0.1000000000000000056 ) ;
#79019=CARTESIAN_POINT ( 'NONE',  ( 13.40000000000005898, 63.75000000001119815, -21.02310748452479316 ) ) ;
#79040=LINE ( 'NONE', #781, #58345 ) ;
#79076=VECTOR ( 'NONE', #186923, 1000.000000000000000 ) ;
#79080=CIRCLE ( 'NONE', #199755, 0.09999999999999939493 ) ;
#79100=DIRECTION ( 'NONE',  ( -1.000000000000000000, 0.000000000000000000, 0.000000000000000000 ) ) ;
#79178=LINE ( 'NONE', #179603, #226272 ) ;
#79191=PLANE ( 'NONE',  #170467 ) ;
#79217=CARTESIAN_POINT ( 'NONE',  ( 5.551115123125782702E-14, 65.35000000001120668, -3.123107484524795474 ) ) ;
#79241=ORIENTED_EDGE ( 'NONE', *, *, #110636, .F. ) ;
#79349=CARTESIAN_POINT ( 'NONE',  ( -23.39999999999994529, 79.88763423575340994, -7.282924647898262549 ) ) ;
#79354=ORIENTED_EDGE ( 'NONE', *, *, #38311, .T. ) ;
#79367=LINE ( 'NONE', #98916, #195542 ) ;
#79389=DIRECTION ( 'NONE',  ( -0.000000000000000000, -1.000000000000000000, 0.000000000000000000 ) ) ;
#79425=EDGE_LOOP ( 'NONE', ( #48444, #51536, #104006, #5945 ) ) ;
#79526=FACE_OUTER_BOUND ( 'NONE', #254827, .T. ) ;
#79533=ORIENTED_EDGE ( 'NONE', *, *, #120961, .F. ) ;
#79534=CARTESIAN_POINT ( 'NONE',  ( 20.95000000000005258, 66.15000000001120384, -5.923107484524795296 ) ) ;
#79546=FACE_OUTER_BOUND ( 'NONE', #87520, .T. ) ;
#79589=CARTESIAN_POINT ( 'NONE',  ( 23.40000000000005542, 77.16254490893143725, -43.92310748452479885 ) ) ;
#79649=ORIENTED_EDGE ( 'NONE', *, *, #88526, .F. ) ;
#79679=AXIS2_PLACEMENT_3D ( 'NONE', #196180, #73694, #153238 ) ;
#79717=ORIENTED_EDGE ( 'NONE', *, *, #67450, .F. ) ;
#79735=DIRECTION ( 'NONE',  ( 0.000000000000000000, -1.156482317317873105E-15, -1.000000000000000000 ) ) ;
#79790=AXIS2_PLACEMENT_3D ( 'NONE', #78269, #178706, #59983 ) ;
#79816=EDGE_CURVE ( 'NONE', #100189, #196305, #136148, .T. ) ;
#79825=TOROIDAL_SURFACE ( 'NONE', #192853, 11.65000000000000036, 0.1000000000000000056 ) ;
#79827=EDGE_LOOP ( 'NONE', ( #165735, #206839, #155024, #139003 ) ) ;
#79918=ORIENTED_EDGE ( 'NONE', *, *, #107769, .T. ) ;
#79933=EDGE_CURVE ( 'NONE', #150745, #110468, #170933, .T. ) ;
#79947=ORIENTED_EDGE ( 'NONE', *, *, #137418, .F. ) ;
#80002=LINE ( 'NONE', #239117, #7988 ) ;
#80009=CARTESIAN_POINT ( 'NONE',  ( -21.14999999999994174, 74.16448838626247664, -47.62760213295649692 ) ) ;
#80029=ORIENTED_EDGE ( 'NONE', *, *, #106886, .T. ) ;
#80092=PLANE ( 'NONE',  #96483 ) ;
#80170=DIRECTION ( 'NONE',  ( 0.000000000000000000, 0.000000000000000000, 1.000000000000000000 ) ) ;
#80209=VERTEX_POINT ( 'NONE', #106725 ) ;
#80220=ORIENTED_EDGE ( 'NONE', *, *, #143369, .T. ) ;
#80255=VERTEX_POINT ( 'NONE', #70216 ) ;
#80270=ORIENTED_EDGE ( 'NONE', *, *, #78938, .T. ) ;
#80281=CYLINDRICAL_SURFACE ( 'NONE', #156766, 0.09999999999999939493 ) ;
#80282=DIRECTION ( 'NONE',  ( 0.000000000000000000, 1.000000000000000000, 0.000000000000000000 ) ) ;
#80288=ORIENTED_EDGE ( 'NONE', *, *, #221486, .F. ) ;
#80305=ORIENTED_EDGE ( 'NONE', *, *, #31723, .F. ) ;
#80351=EDGE_CURVE ( 'NONE', #37851, #118363, #71497, .T. ) ;
#80353=AXIS2_PLACEMENT_3D ( 'NONE', #59642, #194079, #257821 ) ;
#80379=ORIENTED_EDGE ( 'NONE', *, *, #32949, .T. ) ;
#80392=CARTESIAN_POINT ( 'NONE',  ( -21.14999999999994174, 87.50449464844290048, -34.18759587077607165 ) ) ;
#80401=DIRECTION ( 'NONE',  ( 0.000000000000000000, 0.000000000000000000, -1.000000000000000000 ) ) ;
#80404=DIRECTION ( 'NONE',  ( 0.000000000000000000, 0.000000000000000000, 1.000000000000000000 ) ) ;
#80409=EDGE_CURVE ( 'NONE', #76432, #187747, #69937, .T. ) ;
#80411=DIRECTION ( 'NONE',  ( -1.000000000000000000, 0.000000000000000000, 0.000000000000000000 ) ) ;
#80414=DIRECTION ( 'NONE',  ( 0.000000000000000000, 0.000000000000000000, 1.000000000000000000 ) ) ;
#80442=CARTESIAN_POINT ( 'NONE',  ( 21.05000000000005400, 67.85000000001119247, -3.123107484524795474 ) ) ;
#80443=AXIS2_PLACEMENT_3D ( 'NONE', #97083, #217049, #117973 ) ;
#80446=LINE ( 'NONE', #40114, #64742 ) ;
#80523=ADVANCED_FACE ( 'NONE', ( #245957 ), #142966, .T. ) ;
#80541=CIRCLE ( 'NONE', #43170, 2.600000000000000089 ) ;
#80584=EDGE_CURVE ( 'NONE', #245973, #28383, #115710, .T. ) ;
#80585=VERTEX_POINT ( 'NONE', #154286 ) ;
#80633=CIRCLE ( 'NONE', #101263, 2.599999999999998312 ) ;
#80642=CARTESIAN_POINT ( 'NONE',  ( 23.40000000000005542, 73.52684270758111040, -52.27034697567518862 ) ) ;
#80651=ORIENTED_EDGE ( 'NONE', *, *, #28595, .T. ) ;
#80758=FACE_OUTER_BOUND ( 'NONE', #39606, .T. ) ;
#80766=DIRECTION ( 'NONE',  ( 1.000000000000000000, 0.000000000000000000, 0.000000000000000000 ) ) ;
#80780=CIRCLE ( 'NONE', #101610, 0.09999999999999982514 ) ;
#80799=ORIENTED_EDGE ( 'NONE', *, *, #44106, .T. ) ;
#80802=ADVANCED_FACE ( 'NONE', ( #240203 ), #43277, .T. ) ;
#80821=CARTESIAN_POINT ( 'NONE',  ( -23.39999999999994529, 74.16448838626247664, -47.52760213295649550 ) ) ;
#80850=CARTESIAN_POINT ( 'NONE',  ( 5.900000000000060751, 64.25000000001119815, -22.12310748452479103 ) ) ;
#80858=CIRCLE ( 'NONE', #64312, 11.65000000000000036 ) ;
#80876=FACE_OUTER_BOUND ( 'NONE', #113156, .T. ) ;
#80879=VERTEX_POINT ( 'NONE', #22448 ) ;
#80934=ADVANCED_FACE ( 'NONE', ( #70572 ), #182547, .T. ) ;
#80961=VERTEX_POINT ( 'NONE', #225733 ) ;
#81012=CARTESIAN_POINT ( 'NONE',  ( -23.49999999999994316, 87.50449464844290048, -34.18759587077607165 ) ) ;
#81032=EDGE_CURVE ( 'NONE', #201937, #56611, #141032, .T. ) ;
#81095=CARTESIAN_POINT ( 'NONE',  ( -23.49999999999994316, 74.16448838626247664, -47.52760213295649550 ) ) ;
#81102=DIRECTION ( 'NONE',  ( -0.000000000000000000, 1.000000000000000000, 0.000000000000000000 ) ) ;
#81119=DIRECTION ( 'NONE',  ( -1.000000000000000000, -0.000000000000000000, -0.000000000000000000 ) ) ;
#81123=EDGE_CURVE ( 'NONE', #84546, #172317, #45330, .T. ) ;
#81158=EDGE_CURVE ( 'NONE', #139324, #88642, #165986, .T. ) ;
#81172=DIRECTION ( 'NONE',  ( 0.000000000000000000, 1.000000000000000000, 0.000000000000000000 ) ) ;
#81181=CARTESIAN_POINT ( 'NONE',  ( -23.39999999999994529, 87.51781941433023349, -34.28670414799875488 ) ) ;
#81237=DIRECTION ( 'NONE',  ( 0.000000000000000000, 0.000000000000000000, -1.000000000000000000 ) ) ;
#81245=VERTEX_POINT ( 'NONE', #97768 ) ;
#81270=CARTESIAN_POINT ( 'NONE',  ( -20.94999999999994600, 67.65000000001118963, -25.49719488170504533 ) ) ;
#81284=EDGE_LOOP ( 'NONE', ( #194373, #133005, #180703, #124345 ) ) ;
#81290=AXIS2_PLACEMENT_3D ( 'NONE', #87154, #165439, #102856 ) ;
#81314=AXIS2_PLACEMENT_3D ( 'NONE', #73069, #55999, #232118 ) ;
#81328=AXIS2_PLACEMENT_3D ( 'NONE', #84447, #25812, #201882 ) ;
#81349=AXIS2_PLACEMENT_3D ( 'NONE', #243210, #205362, #64576 ) ;
#81380=DIRECTION ( 'NONE',  ( 0.000000000000000000, -0.9910827722268049644, -0.1332476588733589318 ) ) ;
#81392=DIRECTION ( 'NONE',  ( 0.000000000000000000, 0.000000000000000000, -1.000000000000000000 ) ) ;
#81411=DIRECTION ( 'NONE',  ( 0.000000000000000000, 0.1332476588733448597, -0.9910827722268067408 ) ) ;
#81438=CIRCLE ( 'NONE', #23235, 0.1000000000000028644 ) ;
#81477=DIRECTION ( 'NONE',  ( 0.000000000000000000, 0.000000000000000000, -1.000000000000000000 ) ) ;
#81514=ADVANCED_FACE ( 'NONE', ( #156212 ), #79191, .F. ) ;
#81596=DIRECTION ( 'NONE',  ( -0.000000000000000000, 1.000000000000000000, -0.000000000000000000 ) ) ;
#81638=LINE ( 'NONE', #42541, #63415 ) ;
#81698=DIRECTION ( 'NONE',  ( 0.000000000000000000, 1.000000000000000000, 1.224646799147352961E-16 ) ) ;
#81703=AXIS2_PLACEMENT_3D ( 'NONE', #222909, #224194, #109373 ) ;
#81722=EDGE_CURVE ( 'NONE', #26416, #161732, #178833, .T. ) ;
#81728=DIRECTION ( 'NONE',  ( 0.000000000000000000, 1.000000000000000000, 0.000000000000000000 ) ) ;
#81736=ADVANCED_FACE ( 'NONE', ( #146845 ), #148149, .F. ) ;
#81755=CIRCLE ( 'NONE', #65222, 2.599999999999998312 ) ;
#81843=ORIENTED_EDGE ( 'NONE', *, *, #115538, .T. ) ;
#81962=VERTEX_POINT ( 'NONE', #256171 ) ;
#81975=ADVANCED_FACE ( 'NONE', ( #219673 ), #1900, .F. ) ;
#82001=DIRECTION ( 'NONE',  ( 1.000000000000000000, -0.000000000000000000, -3.469446951953515108E-14 ) ) ;
#82114=ORIENTED_EDGE ( 'NONE', *, *, #35563, .F. ) ;
#82157=CIRCLE ( 'NONE', #136318, 0.09999999999999530098 ) ;
#82174=EDGE_LOOP ( 'NONE', ( #251328, #59095, #37349, #119789 ) ) ;
#82223=ORIENTED_EDGE ( 'NONE', *, *, #81158, .T. ) ;
#82254=AXIS2_PLACEMENT_3D ( 'NONE', #178130, #17728, #13909 ) ;
#82259=VECTOR ( 'NONE', #133160, 1000.000000000000000 ) ;
#82314=ORIENTED_EDGE ( 'NONE', *, *, #161533, .T. ) ;
#82317=CARTESIAN_POINT ( 'NONE',  ( -0.8999999999999438449, 67.65000000001118963, -5.981686128287480919 ) ) ;
#82352=CIRCLE ( 'NONE', #69938, 0.1000000000000021844 ) ;
#82358=ORIENTED_EDGE ( 'NONE', *, *, #82603, .F. ) ;
#82361=EDGE_CURVE ( 'NONE', #77787, #177623, #253974, .T. ) ;
#82381=ORIENTED_EDGE ( 'NONE', *, *, #246668, .F. ) ;
#82386=ORIENTED_EDGE ( 'NONE', *, *, #159415, .F. ) ;
#82425=CARTESIAN_POINT ( 'NONE',  ( 21.05000000000005400, 64.35000000001120668, -36.02310748452479316 ) ) ;
#82431=VECTOR ( 'NONE', #153017, 1000.000000000000000 ) ;
#82495=VECTOR ( 'NONE', #96868, 1000.000000000000000 ) ;
#82545=DIRECTION ( 'NONE',  ( -1.000000000000000000, -0.000000000000000000, -0.000000000000000000 ) ) ;
#82569=CIRCLE ( 'NONE', #178497, 0.1999999999999987899 ) ;
#82577=AXIS2_PLACEMENT_3D ( 'NONE', #53860, #229928, #175141 ) ;
#82595=DIRECTION ( 'NONE',  ( 1.000000000000000000, 0.000000000000000000, 0.000000000000000000 ) ) ;
#82603=EDGE_CURVE ( 'NONE', #81962, #218111, #83453, .T. ) ;
#82638=ORIENTED_EDGE ( 'NONE', *, *, #74434, .F. ) ;
#82681=ORIENTED_EDGE ( 'NONE', *, *, #172597, .F. ) ;
#82762=VERTEX_POINT ( 'NONE', #215228 ) ;
#82873=CARTESIAN_POINT ( 'NONE',  ( 20.95000000000005613, 66.15000000001120384, -4.623107484524796362 ) ) ;
#82881=ORIENTED_EDGE ( 'NONE', *, *, #87371, .T. ) ;
#82975=VERTEX_POINT ( 'NONE', #149501 ) ;
#82999=EDGE_CURVE ( 'NONE', #29322, #173155, #92058, .T. ) ;
#83095=ORIENTED_EDGE ( 'NONE', *, *, #135431, .F. ) ;
#83104=CARTESIAN_POINT ( 'NONE',  ( 20.95000000000005258, 64.35000000001120668, -29.92310748452479174 ) ) ;
#83120=EDGE_CURVE ( 'NONE', #134698, #50347, #237791, .T. ) ;
#83135=AXIS2_PLACEMENT_3D ( 'NONE', #23747, #244032, #84929 ) ;
#83136=AXIS2_PLACEMENT_3D ( 'NONE', #182841, #47124, #203660 ) ;
#83139=ORIENTED_EDGE ( 'NONE', *, *, #198246, .T. ) ;
#83143=TOROIDAL_SURFACE ( 'NONE', #183166, 0.2000000000000000111, 0.1000000000000000056 ) ;
#83144=AXIS2_PLACEMENT_3D ( 'NONE', #122851, #235389, #118016 ) ;
#83199=DIRECTION ( 'NONE',  ( -0.000000000000000000, 0.1332476588733589318, 0.9910827722268050755 ) ) ;
#83230=EDGE_CURVE ( 'NONE', #24547, #38614, #129459, .T. ) ;
#83255=CARTESIAN_POINT ( 'NONE',  ( 0.9000000000000547562, 66.35000000001119247, -7.423107484524793520 ) ) ;
#83271=CARTESIAN_POINT ( 'NONE',  ( -0.8999999999999437339, 67.75000000001118394, -7.423107484524793520 ) ) ;
#83279=VECTOR ( 'NONE', #110537, 1000.000000000000000 ) ;
#83291=DIRECTION ( 'NONE',  ( 1.000000000000000000, 0.000000000000000000, -0.000000000000000000 ) ) ;
#83357=CARTESIAN_POINT ( 'NONE',  ( -20.94999999999994600, 65.15000000001120384, -4.423107484524790856 ) ) ;
#83419=FILL_AREA_STYLE ('',( #44338 ) ) ;
#83453=CIRCLE ( 'NONE', #58519, 0.1000000000000002554 ) ;
#83499=ORIENTED_EDGE ( 'NONE', *, *, #176621, .F. ) ;
#83506=FACE_OUTER_BOUND ( 'NONE', #195863, .T. ) ;
#83556=VECTOR ( 'NONE', #206041, 1000.000000000000000 ) ;
#83563=ORIENTED_EDGE ( 'NONE', *, *, #162333, .T. ) ;
#83567=DIRECTION ( 'NONE',  ( 0.000000000000000000, 0.000000000000000000, -1.000000000000000000 ) ) ;
#83568=DIRECTION ( 'NONE',  ( -1.000000000000000000, 0.000000000000000000, 0.000000000000000000 ) ) ;
#83585=DIRECTION ( 'NONE',  ( -0.000000000000000000, 1.000000000000000000, -0.000000000000000000 ) ) ;
#83628=CYLINDRICAL_SURFACE ( 'NONE', #132748, 0.09999999999999939493 ) ;
#83632=CARTESIAN_POINT ( 'NONE',  ( 21.05000000000005400, 67.82483145523551116, -25.59432346794077162 ) ) ;
#83646=CYLINDRICAL_SURFACE ( 'NONE', #236721, 4.049999999999998046 ) ;
#83671=ORIENTED_EDGE ( 'NONE', *, *, #177242, .F. ) ;
#83692=AXIS2_PLACEMENT_3D ( 'NONE', #60632, #119353, #184447 ) ;
#83695=DIRECTION ( 'NONE',  ( 0.000000000000000000, 0.000000000000000000, -1.000000000000000000 ) ) ;
#83702=AXIS2_PLACEMENT_3D ( 'NONE', #128753, #111750, #191319 ) ;
#83734=EDGE_CURVE ( 'NONE', #22457, #126736, #145623, .T. ) ;
#83809=EDGE_CURVE ( 'NONE', #3592, #36158, #12764, .T. ) ;
#83830=CARTESIAN_POINT ( 'NONE',  ( -23.49999999999994316, 64.35000000001120668, -7.323107484524790323 ) ) ;
#83837=EDGE_CURVE ( 'NONE', #255703, #88829, #4335, .T. ) ;
#83841=AXIS2_PLACEMENT_3D ( 'NONE', #214617, #681, #118095 ) ;
#83883=CIRCLE ( 'NONE', #146448, 0.09999999999999939493 ) ;
#83966=CARTESIAN_POINT ( 'NONE',  ( -23.39999999999994529, 77.83551161375991967, -47.52760213295649550 ) ) ;
#84168=EDGE_CURVE ( 'NONE', #75088, #241392, #241862, .T. ) ;
#84170=AXIS2_PLACEMENT_3D ( 'NONE', #242767, #161988, #4160 ) ;
#84197=VERTEX_POINT ( 'NONE', #178428 ) ;
#84259=EDGE_CURVE ( 'NONE', #253379, #201937, #66894, .T. ) ;
#84264=DIRECTION ( 'NONE',  ( 0.000000000000000000, 0.000000000000000000, 1.000000000000000000 ) ) ;
#84268=DIRECTION ( 'NONE',  ( 0.000000000000000000, 1.000000000000000000, 0.000000000000000000 ) ) ;
#84342=LINE ( 'NONE', #103933, #85580 ) ;
#84413=AXIS2_PLACEMENT_3D ( 'NONE', #18358, #125171, #88579 ) ;
#84432=DIRECTION ( 'NONE',  ( -0.000000000000000000, -1.000000000000000000, -0.000000000000000000 ) ) ;
#84447=CARTESIAN_POINT ( 'NONE',  ( 23.40000000000005187, 84.00000000001119815, -37.18565239344504647 ) ) ;
#84483=ORIENTED_EDGE ( 'NONE', *, *, #139837, .F. ) ;
#84501=AXIS2_PLACEMENT_3D ( 'NONE', #72086, #173795, #8569 ) ;
#84527=DIRECTION ( 'NONE',  ( 1.000000000000000000, 0.000000000000000000, 0.000000000000000000 ) ) ;
#84535=DIRECTION ( 'NONE',  ( 1.000000000000000000, 0.000000000000000000, 0.000000000000000000 ) ) ;
#84546=VERTEX_POINT ( 'NONE', #70025 ) ;
#84574=DIRECTION ( 'NONE',  ( -0.000000000000000000, 0.000000000000000000, -1.000000000000000000 ) ) ;
#84575=CIRCLE ( 'NONE', #130412, 0.1999999999999987899 ) ;
#84583=LINE ( 'NONE', #62511, #141134 ) ;
#84610=VECTOR ( 'NONE', #177685, 1000.000000000000114 ) ;
#84625=AXIS2_PLACEMENT_3D ( 'NONE', #195155, #239395, #59424 ) ;
#84678=LINE ( 'NONE', #224220, #10282 ) ;
#84725=CIRCLE ( 'NONE', #14055, 0.09999999999999939493 ) ;
#84887=CARTESIAN_POINT ( 'NONE',  ( 23.50000000000005684, 64.35000000001120668, -51.02310748452479316 ) ) ;
#84895=EDGE_LOOP ( 'NONE', ( #207144, #15912, #43072, #242907 ) ) ;
#84929=DIRECTION ( 'NONE',  ( 0.000000000000000000, 0.000000000000000000, 1.000000000000000000 ) ) ;
#84951=DIRECTION ( 'NONE',  ( -0.000000000000000000, -1.156482317317873105E-15, -1.000000000000000000 ) ) ;
#84997=CARTESIAN_POINT ( 'NONE',  ( -23.49999999999994316, 77.83551161375991967, -47.52760213295649550 ) ) ;
#85007=LINE ( 'NONE', #122893, #89591 ) ;
#85060=ORIENTED_EDGE ( 'NONE', *, *, #226498, .F. ) ;
#85092=CIRCLE ( 'NONE', #239259, 0.09999999999999939493 ) ;
#85114=DIRECTION ( 'NONE',  ( 0.000000000000000000, 0.000000000000000000, 1.000000000000000000 ) ) ;
#85150=DIRECTION ( 'NONE',  ( 1.000000000000000000, 0.000000000000000000, 0.000000000000000000 ) ) ;
#85155=FACE_OUTER_BOUND ( 'NONE', #24833, .T. ) ;
#85160=ORIENTED_EDGE ( 'NONE', *, *, #253358, .F. ) ;
#85168=ORIENTED_EDGE ( 'NONE', *, *, #76753, .F. ) ;
#85228=DIRECTION ( 'NONE',  ( 0.000000000000000000, 1.000000000000000000, 1.224646799147353207E-16 ) ) ;
#85257=CIRCLE ( 'NONE', #27061, 0.1999999999999987899 ) ;
#85304=ORIENTED_EDGE ( 'NONE', *, *, #77210, .T. ) ;
#85316=DIRECTION ( 'NONE',  ( 0.000000000000000000, 0.000000000000000000, 1.000000000000000000 ) ) ;
#85320=CARTESIAN_POINT ( 'NONE',  ( -23.39999999999994529, 77.75000000001119815, -47.64205752314703801 ) ) ;
#85337=AXIS2_PLACEMENT_3D ( 'NONE', #207031, #208331, #89628 ) ;
#85367=DIRECTION ( 'NONE',  ( -0.000000000000000000, 1.000000000000000000, -0.000000000000000000 ) ) ;
#85416=EDGE_CURVE ( 'NONE', #169843, #224621, #9189, .T. ) ;
#85438=AXIS2_PLACEMENT_3D ( 'NONE', #2003, #45001, #123255 ) ;
#85441=DIRECTION ( 'NONE',  ( 0.000000000000000000, -0.1332476588733448597, 0.9910827722268067408 ) ) ;
#85462=DIRECTION ( 'NONE',  ( 0.000000000000000000, 1.000000000000000000, 0.000000000000000000 ) ) ;
#85489=EDGE_CURVE ( 'NONE', #85754, #12539, #171711, .T. ) ;
#85518=DIRECTION ( 'NONE',  ( 1.000000000000000000, 0.000000000000000000, 0.000000000000000000 ) ) ;
#85519=FACE_OUTER_BOUND ( 'NONE', #214031, .T. ) ;
#85563=EDGE_CURVE ( 'NONE', #82975, #23626, #73940, .T. ) ;
#85580=VECTOR ( 'NONE', #160109, 1000.000000000000000 ) ;
#85603=AXIS2_PLACEMENT_3D ( 'NONE', #179988, #160443, #239959 ) ;
#85606=ORIENTED_EDGE ( 'NONE', *, *, #134753, .F. ) ;
#85655=CARTESIAN_POINT ( 'NONE',  ( -20.94999999999994600, 65.35000000001120668, -4.423107484524790856 ) ) ;
#85667=DIRECTION ( 'NONE',  ( 0.000000000000000000, -1.000000000000000000, 0.000000000000000000 ) ) ;
#85673=DIRECTION ( 'NONE',  ( 1.000000000000000000, 0.000000000000000000, 0.000000000000000000 ) ) ;
#85681=VERTEX_POINT ( 'NONE', #138977 ) ;
#85727=CARTESIAN_POINT ( 'NONE',  ( 0.9000000000000546452, 67.72071067812984779, -13.99381816264344813 ) ) ;
#85732=VECTOR ( 'NONE', #172911, 1000.000000000000000 ) ;
#85754=VERTEX_POINT ( 'NONE', #184547 ) ;
#85799=CYLINDRICAL_SURFACE ( 'NONE', #219515, 2.599999999999998312 ) ;
#85828=FACE_OUTER_BOUND ( 'NONE', #227207, .T. ) ;
#85860=CARTESIAN_POINT ( 'NONE',  ( 11.60000000000006004, 67.65000000001118963, -21.02310748452479316 ) ) ;
#85976=CYLINDRICAL_SURFACE ( 'NONE', #232676, 0.09999999999999939493 ) ;
#85979=DIRECTION ( 'NONE',  ( 0.000000000000000000, -1.000000000000000000, 0.000000000000000000 ) ) ;
#86047=VERTEX_POINT ( 'NONE', #60442 ) ;
#86068=CYLINDRICAL_SURFACE ( 'NONE', #163556, 0.1000000000000028644 ) ;
#86073=DIRECTION ( 'NONE',  ( 1.000000000000000000, -0.000000000000000000, -0.000000000000000000 ) ) ;
#86174=EDGE_LOOP ( 'NONE', ( #2010, #98315, #181234, #148435 ) ) ;
#86217=DIRECTION ( 'NONE',  ( -1.000000000000000000, -3.427148797533456523E-14, -5.467925025959484217E-15 ) ) ;
#86271=EDGE_CURVE ( 'NONE', #114442, #41849, #101256, .T. ) ;
#86290=CARTESIAN_POINT ( 'NONE',  ( 23.40000000000005187, 76.00000000001119815, -36.02310748452479316 ) ) ;
#86302=FACE_OUTER_BOUND ( 'NONE', #36187, .T. ) ;
#86318=DIRECTION ( 'NONE',  ( 1.000000000000000000, -0.000000000000000000, 0.000000000000000000 ) ) ;
#86345=CARTESIAN_POINT ( 'NONE',  ( 20.95000000000005613, 65.19115966511134275, -30.12310748452479103 ) ) ;
#86410=ORIENTED_EDGE ( 'NONE', *, *, #174597, .T. ) ;
#86458=ADVANCED_FACE ( 'NONE', ( #23302 ), #142789, .F. ) ;
#86517=CARTESIAN_POINT ( 'NONE',  ( -23.39999999999994529, 76.00000000001119815, -40.17310748452479174 ) ) ;
#86521=CIRCLE ( 'NONE', #127692, 0.09999999999999939493 ) ;
#86527=DIRECTION ( 'NONE',  ( 0.000000000000000000, -0.8164390028469705740, 0.5774316882803059992 ) ) ;
#86557=ORIENTED_EDGE ( 'NONE', *, *, #126501, .F. ) ;
#86632=CARTESIAN_POINT ( 'NONE',  ( 23.50000000000004263, 83.98667523412385094, -37.28476067066772970 ) ) ;
#86639=CYLINDRICAL_SURFACE ( 'NONE', #31767, 0.1000000000000028644 ) ;
#86663=EDGE_LOOP ( 'NONE', ( #250544, #50284, #117290 ) ) ;
#86740=ADVANCED_FACE ( 'NONE', ( #212197 ), #33593, .T. ) ;
#86742=LINE ( 'NONE', #166340, #34437 ) ;
#86764=CARTESIAN_POINT ( 'NONE',  ( -23.39999999999994529, 74.16448838626247664, -47.52760213295649550 ) ) ;
#86806=AXIS2_PLACEMENT_3D ( 'NONE', #227719, #127348, #225139 ) ;
#86833=CARTESIAN_POINT ( 'NONE',  ( 23.40000000000005542, 74.16448838626247664, -47.52760213295649550 ) ) ;
#86897=DIRECTION ( 'NONE',  ( -4.336808689942017736E-16, 0.000000000000000000, -1.000000000000000000 ) ) ;
#86917=ORIENTED_EDGE ( 'NONE', *, *, #53881, .T. ) ;
#86976=DIRECTION ( 'NONE',  ( 0.000000000000000000, 1.000000000000000000, -0.000000000000000000 ) ) ;
#86980=CARTESIAN_POINT ( 'NONE',  ( -23.39999999999994529, 87.50449464844290048, -34.18759587077607165 ) ) ;
#87045=ORIENTED_EDGE ( 'NONE', *, *, #6491, .F. ) ;
#87088=AXIS2_PLACEMENT_3D ( 'NONE', #198167, #42956, #40421 ) ;
#87096=AXIS2_PLACEMENT_3D ( 'NONE', #115679, #56949, #140358 ) ;
#87145=ADVANCED_FACE ( 'NONE', ( #16268 ), #91912, .F. ) ;
#87154=CARTESIAN_POINT ( 'NONE',  ( -23.49999999999994316, 76.00000000001119815, -36.02310748452479316 ) ) ;
#87208=CYLINDRICAL_SURFACE ( 'NONE', #170914, 0.1000000000000028644 ) ;
#87292=CIRCLE ( 'NONE', #58244, 0.1999999999999987899 ) ;
#87369=CARTESIAN_POINT ( 'NONE',  ( -20.94999999999994600, 65.25000000001119815, -4.423107484524790856 ) ) ;
#87371=EDGE_CURVE ( 'NONE', #80209, #173183, #1881, .T. ) ;
#87401=FACE_OUTER_BOUND ( 'NONE', #130332, .T. ) ;
#87520=EDGE_LOOP ( 'NONE', ( #183102, #126840, #250135, #123329 ) ) ;
#87653=CIRCLE ( 'NONE', #233446, 2.700000000000001066 ) ;
#87668=ORIENTED_EDGE ( 'NONE', *, *, #34162, .F. ) ;
#87714=CARTESIAN_POINT ( 'NONE',  ( 23.50000000000005684, 64.25000000001119815, -51.02310748452479316 ) ) ;
#87755=AXIS2_PLACEMENT_3D ( 'NONE', #66986, #202639, #104791 ) ;
#87803=DIRECTION ( 'NONE',  ( -0.000000000000000000, 0.000000000000000000, 1.000000000000000000 ) ) ;
#87836=CARTESIAN_POINT ( 'NONE',  ( -23.39999999999994529, 77.16254490893143725, -43.92310748452479885 ) ) ;
#87892=CYLINDRICAL_SURFACE ( 'NONE', #200451, 0.09999999999999939493 ) ;
#87931=CARTESIAN_POINT ( 'NONE',  ( -23.49999999999994316, 74.16448838626247664, -47.52760213295649550 ) ) ;
#88017=VERTEX_POINT ( 'NONE', #16931 ) ;
#88024=VERTEX_POINT ( 'NONE', #8584 ) ;
#88044=CARTESIAN_POINT ( 'NONE',  ( -23.49999999999994316, 74.94272479589878344, -3.023107484524792277 ) ) ;
#88056=ORIENTED_EDGE ( 'NONE', *, *, #207179, .F. ) ;
#88114=DIRECTION ( 'NONE',  ( -1.000000000000000000, 0.000000000000000000, 0.000000000000000000 ) ) ;
#88122=ORIENTED_EDGE ( 'NONE', *, *, #60527, .F. ) ;
#88129=CARTESIAN_POINT ( 'NONE',  ( -21.04999999999994387, 82.64476912853859858, -26.37791261425322986 ) ) ;
#88201=VERTEX_POINT ( 'NONE', #234036 ) ;
#88228=CYLINDRICAL_SURFACE ( 'NONE', #206633, 0.09999999999999939493 ) ;
#88239=ORIENTED_EDGE ( 'NONE', *, *, #223133, .T. ) ;
#88247=DIRECTION ( 'NONE',  ( 0.000000000000000000, 0.000000000000000000, -1.000000000000000000 ) ) ;
#88252=DIRECTION ( 'NONE',  ( 0.000000000000000000, 0.000000000000000000, -1.000000000000000000 ) ) ;
#88257=DIRECTION ( 'NONE',  ( 0.000000000000000000, -1.000000000000000000, 0.000000000000000000 ) ) ;
#88310=FACE_OUTER_BOUND ( 'NONE', #68875, .T. ) ;
#88361=ORIENTED_EDGE ( 'NONE', *, *, #223133, .F. ) ;
#88378=DIRECTION ( 'NONE',  ( 0.000000000000000000, -1.000000000000000000, -0.000000000000000000 ) ) ;
#88408=CARTESIAN_POINT ( 'NONE',  ( 21.15000000000005542, 64.35000000001120668, -3.123107484524795474 ) ) ;
#88486=ORIENTED_EDGE ( 'NONE', *, *, #83230, .T. ) ;
#88489=DIRECTION ( 'NONE',  ( -0.000000000000000000, -0.000000000000000000, -1.000000000000000000 ) ) ;
#88526=EDGE_CURVE ( 'NONE', #30427, #33613, #81438, .T. ) ;
#88574=ADVANCED_FACE ( 'NONE', ( #254554 ), #75955, .T. ) ;
#88579=DIRECTION ( 'NONE',  ( 0.000000000000000000, 0.000000000000000000, -1.000000000000000000 ) ) ;
#88583=ORIENTED_EDGE ( 'NONE', *, *, #23722, .T. ) ;
#88592=DIRECTION ( 'NONE',  ( 1.000000000000000000, 0.000000000000000000, 0.000000000000000000 ) ) ;
#88642=VERTEX_POINT ( 'NONE', #90367 ) ;
#88644=CARTESIAN_POINT ( 'NONE',  ( -23.49999999999994316, 77.83551161375991967, -47.52760213295649550 ) ) ;
#88657=DIRECTION ( 'NONE',  ( -1.000000000000000000, -0.000000000000000000, -0.000000000000000000 ) ) ;
#88688=DIRECTION ( 'NONE',  ( 1.000000000000000000, -0.000000000000000000, 0.000000000000000000 ) ) ;
#88811=CARTESIAN_POINT ( 'NONE',  ( -23.49999999999994316, 79.88763423575340994, -7.282924647898262549 ) ) ;
#88829=VERTEX_POINT ( 'NONE', #194185 ) ;
#88833=VECTOR ( 'NONE', #48940, 1000.000000000000000 ) ;
#88840=EDGE_CURVE ( 'NONE', #214650, #106794, #180496, .T. ) ;
#88842=CIRCLE ( 'NONE', #184326, 0.1999999999999996503 ) ;
#88858=CIRCLE ( 'NONE', #13870, 0.1000000000000002554 ) ;
#88898=FACE_OUTER_BOUND ( 'NONE', #18983, .T. ) ;
#88906=AXIS2_PLACEMENT_3D ( 'NONE', #199632, #41843, #219151 ) ;
#88964=ORIENTED_EDGE ( 'NONE', *, *, #65252, .T. ) ;
#88966=ORIENTED_EDGE ( 'NONE', *, *, #9637, .T. ) ;
#88999=ORIENTED_EDGE ( 'NONE', *, *, #147746, .T. ) ;
#89008=FILL_AREA_STYLE ('',( #66892 ) ) ;
#89053=CIRCLE ( 'NONE', #213974, 0.09999999999999939493 ) ;
#89074=CIRCLE ( 'NONE', #238937, 0.1000000000000002554 ) ;
#89113=ORIENTED_EDGE ( 'NONE', *, *, #78192, .T. ) ;
#89209=CARTESIAN_POINT ( 'NONE',  ( 11.60000000000006004, 64.35000000001120668, -21.02310748452479316 ) ) ;
#89228=EDGE_CURVE ( 'NONE', #82975, #92271, #5858, .T. ) ;
#89274=LINE ( 'NONE', #91855, #139618 ) ;
#89358=LINE ( 'NONE', #125920, #237733 ) ;
#89373=ADVANCED_FACE ( 'NONE', ( #177045 ), #132780, .F. ) ;
#89441=AXIS2_PLACEMENT_3D ( 'NONE', #53572, #212656, #253045 ) ;
#89464=VERTEX_POINT ( 'NONE', #80442 ) ;
#89495=ADVANCED_FACE ( 'NONE', ( #137869 ), #59606, .T. ) ;
#89591=VECTOR ( 'NONE', #184127, 1000.000000000000000 ) ;
#89600=CARTESIAN_POINT ( 'NONE',  ( -21.14999999999994174, 77.83551161375991967, -47.52760213295649550 ) ) ;
#89622=ORIENTED_EDGE ( 'NONE', *, *, #161503, .F. ) ;
#89628=DIRECTION ( 'NONE',  ( 0.000000000000000000, 0.000000000000000000, 1.000000000000000000 ) ) ;
#89632=CONICAL_SURFACE ( 'NONE', #189617, 4.000000000000000000, 0.7853981633974487231 ) ;
#89695=ORIENTED_EDGE ( 'NONE', *, *, #63929, .F. ) ;
#89809=EDGE_LOOP ( 'NONE', ( #152403, #145042, #98489, #214069 ) ) ;
#89823=LINE ( 'NONE', #92394, #62968 ) ;
#89839=ADVANCED_FACE ( 'NONE', ( #25049 ), #185378, .F. ) ;
#89860=DIRECTION ( 'NONE',  ( 0.000000000000000000, 0.1480365673253017378, -0.9889818879709282307 ) ) ;
#89883=FACE_OUTER_BOUND ( 'NONE', #165013, .T. ) ;
#89909=VERTEX_POINT ( 'NONE', #2871 ) ;
#90057=VERTEX_POINT ( 'NONE', #254314 ) ;
#90073=DIRECTION ( 'NONE',  ( 0.000000000000000000, -1.000000000000000000, 0.000000000000000000 ) ) ;
#90075=EDGE_LOOP ( 'NONE', ( #78119, #241498 ) ) ;
#90083=CARTESIAN_POINT ( 'NONE',  ( -11.59999999999994458, 67.65000000001118963, -21.02310748452479316 ) ) ;
#90100=DIRECTION ( 'NONE',  ( -1.000000000000000000, 0.000000000000000000, 0.000000000000000000 ) ) ;
#90103=VECTOR ( 'NONE', #214596, 1000.000000000000114 ) ;
#90141=DIRECTION ( 'NONE',  ( -0.000000000000000000, 1.000000000000000000, -0.000000000000000000 ) ) ;
#90143=ADVANCED_FACE ( 'NONE', ( #79526 ), #159113, .T. ) ;
#90153=CARTESIAN_POINT ( 'NONE',  ( 23.50000000000005684, 76.00000000001119815, -31.87310748452479459 ) ) ;
#90210=CIRCLE ( 'NONE', #165241, 11.75000000000000000 ) ;
#90225=ORIENTED_EDGE ( 'NONE', *, *, #242478, .T. ) ;
#90251=ORIENTED_EDGE ( 'NONE', *, *, #83230, .F. ) ;
#90253=CIRCLE ( 'NONE', #44509, 0.1000000000000002554 ) ;
#90293=VERTEX_POINT ( 'NONE', #185065 ) ;
#90342=ORIENTED_EDGE ( 'NONE', *, *, #3574, .F. ) ;
#90367=CARTESIAN_POINT ( 'NONE',  ( -21.14999999999994174, 77.26165318615413469, -44.00978271863746016 ) ) ;
#90481=DIRECTION ( 'NONE',  ( 0.000000000000000000, 1.000000000000000000, 0.000000000000000000 ) ) ;
#90507=VERTEX_POINT ( 'NONE', #15434 ) ;
#90549=DIRECTION ( 'NONE',  ( 0.000000000000000000, 0.7071067811865472397, -0.7071067811865479058 ) ) ;
#90557=DIRECTION ( 'NONE',  ( 0.000000000000000000, -0.1480365673253065117, 0.9889818879709273425 ) ) ;
#90576=DIRECTION ( 'NONE',  ( 0.000000000000000000, 0.000000000000000000, -1.000000000000000000 ) ) ;
#90650=AXIS2_PLACEMENT_3D ( 'NONE', #159167, #202121, #58723 ) ;
#90683=TOROIDAL_SURFACE ( 'NONE', #32474, 0.2000000000000000111, 0.1000000000000000056 ) ;
#90689=VECTOR ( 'NONE', #256126, 1000.000000000000114 ) ;
#90746=DIRECTION ( 'NONE',  ( 1.000000000000000000, 0.000000000000000000, -0.000000000000000000 ) ) ;
#90778=ORIENTED_EDGE ( 'NONE', *, *, #151864, .F. ) ;
#90784=ORIENTED_EDGE ( 'NONE', *, *, #108525, .F. ) ;
#90867=EDGE_CURVE ( 'NONE', #147247, #133820, #80858, .T. ) ;
#90916=ORIENTED_EDGE ( 'NONE', *, *, #110149, .F. ) ;
#90955=DIRECTION ( 'NONE',  ( -1.000000000000000000, 0.000000000000000000, 0.000000000000000000 ) ) ;
#91040=AXIS2_PLACEMENT_3D ( 'NONE', #139645, #195819, #155421 ) ;
#91044=VECTOR ( 'NONE', #201543, 1000.000000000000114 ) ;
#91083=VECTOR ( 'NONE', #107292, 1000.000000000000000 ) ;
#91137=FACE_OUTER_BOUND ( 'NONE', #230847, .T. ) ;
#91150=CARTESIAN_POINT ( 'NONE',  ( 21.05000000000005400, 74.94272479589878344, -8.023107484524793165 ) ) ;
#91151=DIRECTION ( 'NONE',  ( 0.000000000000000000, 0.9889818879709272315, 0.1480365673253073999 ) ) ;
#91162=DIRECTION ( 'NONE',  ( 0.000000000000000000, -0.9875102702516471709, 0.1575546449569757979 ) ) ;
#91215=ORIENTED_EDGE ( 'NONE', *, *, #179815, .F. ) ;
#91246=DIRECTION ( 'NONE',  ( 0.000000000000000000, 0.000000000000000000, -1.000000000000000000 ) ) ;
#91312=ORIENTED_EDGE ( 'NONE', *, *, #93795, .T. ) ;
#91318=SPHERICAL_SURFACE ( 'NONE', #237793, 0.1000000000000000056 ) ;
#91339=FACE_OUTER_BOUND ( 'NONE', #120246, .T. ) ;
#91434=CARTESIAN_POINT ( 'NONE',  ( 5.551115123125782702E-14, 64.35000000001120668, -3.123107484524795474 ) ) ;
#91606=DIRECTION ( 'NONE',  ( -0.000000000000000000, -1.000000000000000000, 0.000000000000000000 ) ) ;
#91646=DIRECTION ( 'NONE',  ( 1.000000000000000000, 0.000000000000000000, 0.000000000000000000 ) ) ;
#91655=DIRECTION ( 'NONE',  ( 0.000000000000000000, -1.000000000000000000, 0.000000000000000000 ) ) ;
#91710=CARTESIAN_POINT ( 'NONE',  ( 0.9000000000000546452, 67.75000000001118394, -14.06452884076210630 ) ) ;
#91788=EDGE_CURVE ( 'NONE', #117140, #297, #102235, .T. ) ;
#91837=CYLINDRICAL_SURFACE ( 'NONE', #183572, 0.1000000000000002554 ) ;
#91855=CARTESIAN_POINT ( 'NONE',  ( -21.04999999999994387, 85.92654454508293327, -48.30233646433089234 ) ) ;
#91879=EDGE_LOOP ( 'NONE', ( #90916, #124282, #51962, #52076 ) ) ;
#91912=CYLINDRICAL_SURFACE ( 'NONE', #159972, 0.1000000000000002554 ) ;
#91979=ADVANCED_FACE ( 'NONE', ( #155970 ), #52979, .F. ) ;
#91994=CIRCLE ( 'NONE', #71175, 0.09999999999999939493 ) ;
#92033=DIRECTION ( 'NONE',  ( 1.000000000000000000, -0.000000000000000000, 0.000000000000000000 ) ) ;
#92045=EDGE_CURVE ( 'NONE', #85754, #75088, #206337, .T. ) ;
#92058=LINE ( 'NONE', #54213, #46237 ) ;
#92060=DIRECTION ( 'NONE',  ( -0.000000000000000000, 1.000000000000000000, -0.000000000000000000 ) ) ;
#92067=CARTESIAN_POINT ( 'NONE',  ( -11.59999999999994458, 64.25000000001119815, -21.02310748452479316 ) ) ;
#92077=DIRECTION ( 'NONE',  ( 0.000000000000000000, 0.000000000000000000, -1.000000000000000000 ) ) ;
#92084=CARTESIAN_POINT ( 'NONE',  ( 5.900000000000059863, 64.75000000001119815, -25.92310748452479174 ) ) ;
#92087=CIRCLE ( 'NONE', #29585, 2.599999999999998312 ) ;
#92090=LINE ( 'NONE', #155949, #172186 ) ;
#92108=FACE_OUTER_BOUND ( 'NONE', #222910, .T. ) ;
#92143=DIRECTION ( 'NONE',  ( 0.000000000000000000, 0.000000000000000000, 1.000000000000000000 ) ) ;
#92205=PLANE ( 'NONE',  #72532 ) ;
#92245=ADVANCED_FACE ( 'NONE', ( #8429 ), #86639, .T. ) ;
#92269=CIRCLE ( 'NONE', #221248, 0.1000000000000028644 ) ;
#92271=VERTEX_POINT ( 'NONE', #147939 ) ;
#92371=DIRECTION ( 'NONE',  ( 1.000000000000000000, 0.000000000000000000, 0.000000000000000000 ) ) ;
#92394=CARTESIAN_POINT ( 'NONE',  ( 13.40000000000005898, 63.75000000001119815, -21.02310748452479316 ) ) ;
#92397=AXIS2_PLACEMENT_3D ( 'NONE', #209000, #66919, #149050 ) ;
#92423=ORIENTED_EDGE ( 'NONE', *, *, #151917, .T. ) ;
#92433=DIRECTION ( 'NONE',  ( 0.000000000000000000, 0.000000000000000000, -1.000000000000000000 ) ) ;
#92484=VECTOR ( 'NONE', #29258, 1000.000000000000000 ) ;
#92493=DIRECTION ( 'NONE',  ( 0.000000000000000000, 8.673617379884042375E-16, 1.000000000000000000 ) ) ;
#92505=ORIENTED_EDGE ( 'NONE', *, *, #21887, .T. ) ;
#92530=ORIENTED_EDGE ( 'NONE', *, *, #230793, .F. ) ;
#92569=DIRECTION ( 'NONE',  ( 0.000000000000000000, 0.000000000000000000, 1.000000000000000000 ) ) ;
#92570=ORIENTED_EDGE ( 'NONE', *, *, #216561, .F. ) ;
#92589=CARTESIAN_POINT ( 'NONE',  ( 13.40000000000005898, 67.72071067812984779, -17.05239680640613997 ) ) ;
#92593=ORIENTED_EDGE ( 'NONE', *, *, #218992, .F. ) ;
#92639=CARTESIAN_POINT ( 'NONE',  ( 20.95000000000005258, 66.15000000001120384, -6.023107484524794941 ) ) ;
#92696=ORIENTED_EDGE ( 'NONE', *, *, #164989, .F. ) ;
#92705=CARTESIAN_POINT ( 'NONE',  ( 13.40000000000005898, 67.72071067812984779, -24.99381816264344636 ) ) ;
#92795=ORIENTED_EDGE ( 'NONE', *, *, #82361, .T. ) ;
#92827=EDGE_LOOP ( 'NONE', ( #64072, #118136, #139787, #35117 ) ) ;
#92854=CIRCLE ( 'NONE', #80353, 0.09999999999999982514 ) ;
#92857=ORIENTED_EDGE ( 'NONE', *, *, #201979, .F. ) ;
#92865=ORIENTED_EDGE ( 'NONE', *, *, #134649, .F. ) ;
#92890=DIRECTION ( 'NONE',  ( 0.000000000000000000, -0.9910827722268036322, 0.1332476588733685074 ) ) ;
#92925=ADVANCED_FACE ( 'NONE', ( #204488 ), #85799, .F. ) ;
#92990=AXIS2_PLACEMENT_3D ( 'NONE', #205352, #128408, #65857 ) ;
#93010=VECTOR ( 'NONE', #241580, 1000.000000000000000 ) ;
#93094=ORIENTED_EDGE ( 'NONE', *, *, #201940, .F. ) ;
#93228=ORIENTED_EDGE ( 'NONE', *, *, #19328, .T. ) ;
#93249=CARTESIAN_POINT ( 'NONE',  ( -21.14999999999994174, 64.25000000001119815, -3.123107484524795474 ) ) ;
#93303=ORIENTED_EDGE ( 'NONE', *, *, #63228, .T. ) ;
#93305=AXIS2_PLACEMENT_3D ( 'NONE', #202584, #82595, #241709 ) ;
#93338=ORIENTED_EDGE ( 'NONE', *, *, #19244, .F. ) ;
#93374=EDGE_LOOP ( 'NONE', ( #70478, #152201, #55147, #195593 ) ) ;
#93398=DIRECTION ( 'NONE',  ( 0.000000000000000000, 0.000000000000000000, 1.000000000000000000 ) ) ;
#93408=DIRECTION ( 'NONE',  ( -1.000000000000000000, 0.000000000000000000, 0.000000000000000000 ) ) ;
#93443=CARTESIAN_POINT ( 'NONE',  ( 5.900000000000059863, 64.35000000001120668, -25.92310748452479174 ) ) ;
#93488=EDGE_LOOP ( 'NONE', ( #128630, #139031, #144850, #12036 ) ) ;
#93497=CIRCLE ( 'NONE', #118465, 11.74999999999999645 ) ;
#93539=CARTESIAN_POINT ( 'NONE',  ( -21.04999999999994387, 64.35000000001120668, -36.02310748452479316 ) ) ;
#93574=LINE ( 'NONE', #94848, #116468 ) ;
#93583=EDGE_CURVE ( 'NONE', #186109, #231870, #165756, .T. ) ;
#93616=DIRECTION ( 'NONE',  ( 0.000000000000000000, 0.000000000000000000, 1.000000000000000000 ) ) ;
#93630=CARTESIAN_POINT ( 'NONE',  ( -5.999999999999938716, 64.65000000001120384, -25.92310748452479174 ) ) ;
#93644=CIRCLE ( 'NONE', #126959, 0.1000000000000028644 ) ;
#93670=DIRECTION ( 'NONE',  ( 0.000000000000000000, 0.000000000000000000, 1.000000000000000000 ) ) ;
#93686=DIRECTION ( 'NONE',  ( -4.336808689942017736E-16, 0.000000000000000000, -1.000000000000000000 ) ) ;
#93701=DIRECTION ( 'NONE',  ( 0.000000000000000000, -1.156482317317873105E-15, -1.000000000000000000 ) ) ;
#93792=DIRECTION ( 'NONE',  ( 0.000000000000000000, -1.000000000000000000, 0.000000000000000000 ) ) ;
#93795=EDGE_CURVE ( 'NONE', #144818, #9346, #157392, .T. ) ;
#93897=ADVANCED_FACE ( 'NONE', ( #52497 ), #7714, .T. ) ;
#93946=CARTESIAN_POINT ( 'NONE',  ( 5.900000000000060751, 64.35000000001120668, -21.92310748452479174 ) ) ;
#93962=EDGE_LOOP ( 'NONE', ( #141843, #7832, #133189, #193627 ) ) ;
#94021=ADVANCED_FACE ( 'NONE', ( #253270 ), #173808, .T. ) ;
#94032=AXIS2_PLACEMENT_3D ( 'NONE', #84997, #47160, #28959 ) ;
#94084=AXIS2_PLACEMENT_3D ( 'NONE', #161, #57562, #139661 ) ;
#94129=EDGE_CURVE ( 'NONE', #144177, #169497, #236637, .T. ) ;
#94146=CARTESIAN_POINT ( 'NONE',  ( -21.14999999999994174, 64.35000000001120668, -3.123107484524795474 ) ) ;
#94163=DIRECTION ( 'NONE',  ( 0.000000000000000000, 0.000000000000000000, -1.000000000000000000 ) ) ;
#94244=FACE_OUTER_BOUND ( 'NONE', #126359, .T. ) ;
#94289=DIRECTION ( 'NONE',  ( -1.000000000000000000, -4.624352451196580357E-15, 3.439547145395922042E-14 ) ) ;
#94373=AXIS2_PLACEMENT_3D ( 'NONE', #31736, #69558, #246885 ) ;
#94405=AXIS2_PLACEMENT_3D ( 'NONE', #83966, #223512, #141419 ) ;
#94406=CARTESIAN_POINT ( 'NONE',  ( 11.60000000000006182, 63.75000000001119815, -21.02310748452479316 ) ) ;
#94412=EDGE_CURVE ( 'NONE', #225270, #133820, #28785, .T. ) ;
#94435=DIRECTION ( 'NONE',  ( 1.000000000000000000, 0.000000000000000000, 0.000000000000000000 ) ) ;
#94446=FACE_OUTER_BOUND ( 'NONE', #148993, .T. ) ;
#94461=DIRECTION ( 'NONE',  ( -3.469446951953515108E-14, 0.000000000000000000, 1.000000000000000000 ) ) ;
#94468=CARTESIAN_POINT ( 'NONE',  ( 21.05000000000005400, 67.65000000001118963, -14.06452884076210630 ) ) ;
#94475=DIRECTION ( 'NONE',  ( 0.000000000000000000, 0.000000000000000000, -1.000000000000000000 ) ) ;
#94511=DIRECTION ( 'NONE',  ( 0.000000000000000000, 1.000000000000000000, 0.000000000000000000 ) ) ;
#94528=AXIS2_PLACEMENT_3D ( 'NONE', #14715, #91655, #250717 ) ;
#94552=ADVANCED_FACE ( 'NONE', ( #129823 ), #211955, .F. ) ;
#94637=LINE ( 'NONE', #191210, #44639 ) ;
#94664=CARTESIAN_POINT ( 'NONE',  ( -21.04999999999994387, 76.00000000001119815, -36.02310748452479316 ) ) ;
#94673=EDGE_CURVE ( 'NONE', #133332, #114106, #140082, .T. ) ;
#94692=CARTESIAN_POINT ( 'NONE',  ( 20.95000000000005613, 67.75000000001118394, -25.52310748452478606 ) ) ;
#94694=CARTESIAN_POINT ( 'NONE',  ( -23.49999999999994316, 74.83745509109094485, -43.82310748452479743 ) ) ;
#94709=DIRECTION ( 'NONE',  ( 0.000000000000000000, 0.000000000000000000, -1.000000000000000000 ) ) ;
#94738=ADVANCED_FACE ( 'NONE', ( #63117 ), #219686, .F. ) ;
#94783=TOROIDAL_SURFACE ( 'NONE', #240543, 0.2000000000000000111, 0.1000000000000000056 ) ;
#94791=ADVANCED_FACE ( 'NONE', ( #146502 ), #205195, .T. ) ;
#94825=ORIENTED_EDGE ( 'NONE', *, *, #143594, .F. ) ;
#94834=DIRECTION ( 'NONE',  ( 1.000000000000000000, 0.000000000000000000, 0.000000000000000000 ) ) ;
#94848=CARTESIAN_POINT ( 'NONE',  ( -5.999999999999938716, 64.35000000001120668, -26.02310748452479316 ) ) ;
#94855=EDGE_CURVE ( 'NONE', #112788, #221278, #57362, .T. ) ;
#94882=ADVANCED_FACE ( 'NONE', ( #142648 ), #123118, .T. ) ;
#94978=VECTOR ( 'NONE', #118861, 1000.000000000000000 ) ;
#95003=CIRCLE ( 'NONE', #65960, 0.09999999999999982514 ) ;
#95004=DIRECTION ( 'NONE',  ( -1.000000000000000000, -3.427148797533456523E-14, -5.467925025959484217E-15 ) ) ;
#95215=CARTESIAN_POINT ( 'NONE',  ( -23.39999999999994529, 64.25000000001119815, -51.02310748452479316 ) ) ;
#95227=CARTESIAN_POINT ( 'NONE',  ( -0.8999999999999437339, 64.35000000001120668, -10.02310748452479139 ) ) ;
#95292=CARTESIAN_POINT ( 'NONE',  ( -13.39999999999994351, 66.35000000001119247, -23.62310748452479103 ) ) ;
#95301=CIRCLE ( 'NONE', #141651, 2.599999999999998312 ) ;
#95330=ORIENTED_EDGE ( 'NONE', *, *, #109112, .F. ) ;
#95358=ORIENTED_EDGE ( 'NONE', *, *, #59944, .T. ) ;
#95437=LINE ( 'NONE', #253219, #78028 ) ;
#95441=EDGE_LOOP ( 'NONE', ( #2667, #127763, #3941, #241634 ) ) ;
#95448=ORIENTED_EDGE ( 'NONE', *, *, #64134, .T. ) ;
#95500=CARTESIAN_POINT ( 'NONE',  ( -21.14999999999994174, 79.88763423575340994, -7.282924647898262549 ) ) ;
#95561=EDGE_CURVE ( 'NONE', #57819, #59493, #128482, .T. ) ;
#95566=CARTESIAN_POINT ( 'NONE',  ( 21.15000000000005187, 87.50449464844290048, -37.85861909827351468 ) ) ;
#95644=ADVANCED_FACE ( 'NONE', ( #6397 ), #66120, .T. ) ;
#95802=DIRECTION ( 'NONE',  ( 0.000000000000000000, -0.000000000000000000, -1.000000000000000000 ) ) ;
#95865=LINE ( 'NONE', #124132, #70175 ) ;
#95872=AXIS2_PLACEMENT_3D ( 'NONE', #102038, #220729, #180323 ) ;
#95876=DIRECTION ( 'NONE',  ( 0.000000000000000000, -1.000000000000000000, 0.000000000000000000 ) ) ;
#95879=DIRECTION ( 'NONE',  ( 0.000000000000000000, 0.000000000000000000, 1.000000000000000000 ) ) ;
#95909=DIRECTION ( 'NONE',  ( 0.000000000000000000, 0.9875102702516471709, 0.1575546449569757979 ) ) ;
#95979=ORIENTED_EDGE ( 'NONE', *, *, #225434, .F. ) ;
#96062=CARTESIAN_POINT ( 'NONE',  ( 20.95000000000005258, 66.15000000001120384, -4.523107484524794053 ) ) ;
#96065=ORIENTED_EDGE ( 'NONE', *, *, #77036, .T. ) ;
#96099=EDGE_LOOP ( 'NONE', ( #41877, #22102, #82681, #26266 ) ) ;
#96124=DIRECTION ( 'NONE',  ( 1.000000000000000000, 0.000000000000000000, 0.000000000000000000 ) ) ;
#96129=CIRCLE ( 'NONE', #129475, 0.1000000000000028644 ) ;
#96131=ORIENTED_EDGE ( 'NONE', *, *, #67848, .T. ) ;
#96171=CARTESIAN_POINT ( 'NONE',  ( -21.14999999999994174, 77.73640333653723644, -47.54092689884382850 ) ) ;
#96200=TOROIDAL_SURFACE ( 'NONE', #12851, 11.65000000000000036, 0.1000000000000000056 ) ;
#96213=AXIS2_PLACEMENT_3D ( 'NONE', #161245, #221188, #24311 ) ;
#96233=DIRECTION ( 'NONE',  ( -0.000000000000000000, 0.4856429311786307768, 0.8741572761215385956 ) ) ;
#96248=CARTESIAN_POINT ( 'NONE',  ( -13.39999999999994529, 64.25000000001119815, -21.02310748452479316 ) ) ;
#96258=CARTESIAN_POINT ( 'NONE',  ( -23.49999999999994316, 77.36076146337680370, -43.99645795275012006 ) ) ;
#96318=CYLINDRICAL_SURFACE ( 'NONE', #235560, 0.09999999999999939493 ) ;
#96327=DIRECTION ( 'NONE',  ( 0.000000000000000000, -1.000000000000000000, 8.673617379884042375E-16 ) ) ;
#96349=CARTESIAN_POINT ( 'NONE',  ( -23.49999999999994316, 84.00000000001119815, -37.18565239344504647 ) ) ;
#96358=CARTESIAN_POINT ( 'NONE',  ( 23.40000000000005542, 83.90000000001120384, -37.18565239344504647 ) ) ;
#96366=DIRECTION ( 'NONE',  ( -1.000000000000000000, 0.000000000000000000, 0.000000000000000000 ) ) ;
#96369=DIRECTION ( 'NONE',  ( 1.000000000000000000, 0.000000000000000000, 0.000000000000000000 ) ) ;
#96414=DIRECTION ( 'NONE',  ( -1.000000000000000000, 0.000000000000000000, 0.000000000000000000 ) ) ;
#96483=AXIS2_PLACEMENT_3D ( 'NONE', #103530, #81380, #99668 ) ;
#96512=CIRCLE ( 'NONE', #242270, 4.049999999999998046 ) ;
#96537=ORIENTED_EDGE ( 'NONE', *, *, #215398, .F. ) ;
#96599=CARTESIAN_POINT ( 'NONE',  ( -5.899999999999938183, 64.25000000001119815, -25.92310748452479174 ) ) ;
#96629=EDGE_CURVE ( 'NONE', #173155, #252143, #207312, .T. ) ;
#96662=ORIENTED_EDGE ( 'NONE', *, *, #218031, .T. ) ;
#96666=DIRECTION ( 'NONE',  ( 0.000000000000000000, 0.000000000000000000, -1.000000000000000000 ) ) ;
#96694=LINE ( 'NONE', #137146, #16826 ) ;
#96702=CIRCLE ( 'NONE', #125765, 0.09999999999999939493 ) ;
#96768=CARTESIAN_POINT ( 'NONE',  ( 21.05000000000005400, 65.36599112033563586, -30.02023607076051803 ) ) ;
#96796=DIRECTION ( 'NONE',  ( 1.000000000000000000, 0.000000000000000000, -0.000000000000000000 ) ) ;
#96858=ADVANCED_FACE ( 'NONE', ( #256627 ), #129219, .T. ) ;
#96868=DIRECTION ( 'NONE',  ( -0.000000000000000000, 1.000000000000000000, -0.000000000000000000 ) ) ;
#96904=VERTEX_POINT ( 'NONE', #196704 ) ;
#96927=ORIENTED_EDGE ( 'NONE', *, *, #2289, .F. ) ;
#96934=DIRECTION ( 'NONE',  ( 0.000000000000000000, 0.000000000000000000, -1.000000000000000000 ) ) ;
#96953=EDGE_CURVE ( 'NONE', #211183, #195803, #237127, .T. ) ;
#96973=ORIENTED_EDGE ( 'NONE', *, *, #55824, .F. ) ;
#97028=CIRCLE ( 'NONE', #242817, 5.000000000000000888 ) ;
#97050=VECTOR ( 'NONE', #107844, 1000.000000000000000 ) ;
#97083=CARTESIAN_POINT ( 'NONE',  ( -20.94999999999994600, 64.25000000001119815, -30.12310748452479103 ) ) ;
#97173=DIRECTION ( 'NONE',  ( 1.000000000000000000, 0.000000000000000000, 0.000000000000000000 ) ) ;
#97207=CARTESIAN_POINT ( 'NONE',  ( 23.50000000000005684, 83.80000000001119531, -51.02310748452479316 ) ) ;
#97289=ADVANCED_FACE ( 'NONE', ( #44728 ), #42164, .T. ) ;
#97292=EDGE_CURVE ( 'NONE', #113568, #60596, #179952, .T. ) ;
#97298=EDGE_LOOP ( 'NONE', ( #101591, #129840, #152793 ) ) ;
#97363=VERTEX_POINT ( 'NONE', #69436 ) ;
#97408=CARTESIAN_POINT ( 'NONE',  ( -23.49999999999994316, 84.00000000001119815, -37.18565239344504647 ) ) ;
#97428=ORIENTED_EDGE ( 'NONE', *, *, #71125, .F. ) ;
#97447=LINE ( 'NONE', #236998, #237132 ) ;
#97466=ORIENTED_EDGE ( 'NONE', *, *, #150092, .F. ) ;
#97476=VERTEX_POINT ( 'NONE', #232366 ) ;
#97491=EDGE_LOOP ( 'NONE', ( #104144, #197029, #32296, #172115 ) ) ;
#97507=ORIENTED_EDGE ( 'NONE', *, *, #188694, .T. ) ;
#97515=CIRCLE ( 'NONE', #105895, 0.09999999999999530098 ) ;
#97570=CARTESIAN_POINT ( 'NONE',  ( -21.14999999999994174, 67.85000000001119247, -3.023107484524792277 ) ) ;
#97604=ORIENTED_EDGE ( 'NONE', *, *, #208286, .F. ) ;
#97646=AXIS2_PLACEMENT_3D ( 'NONE', #71371, #209581, #171767 ) ;
#97648=VECTOR ( 'NONE', #78555, 1000.000000000000114 ) ;
#97664=EDGE_CURVE ( 'NONE', #65513, #81245, #230189, .T. ) ;
#97690=ORIENTED_EDGE ( 'NONE', *, *, #237074, .T. ) ;
#97696=FACE_OUTER_BOUND ( 'NONE', #203434, .T. ) ;
#97713=EDGE_CURVE ( 'NONE', #227850, #116777, #122688, .T. ) ;
#97719=ADVANCED_FACE ( 'NONE', ( #169540 ), #86068, .T. ) ;
#97768=CARTESIAN_POINT ( 'NONE',  ( 6.000000000000061284, 64.35000000001120668, -22.12310748452479103 ) ) ;
#97771=DIRECTION ( 'NONE',  ( -0.000000000000000000, 1.000000000000000000, -8.673617379884045333E-16 ) ) ;
#97779=DIRECTION ( 'NONE',  ( 0.000000000000000000, 0.000000000000000000, -1.000000000000000000 ) ) ;
#97785=VECTOR ( 'NONE', #163639, 1000.000000000000000 ) ;
#97787=ORIENTED_EDGE ( 'NONE', *, *, #116022, .F. ) ;
#97803=CARTESIAN_POINT ( 'NONE',  ( 13.40000000000005898, 66.35000000001119247, -23.62310748452479103 ) ) ;
#97841=CIRCLE ( 'NONE', #243617, 0.1000000000000016709 ) ;
#97846=DIRECTION ( 'NONE',  ( -0.000000000000000000, 1.000000000000000000, -0.000000000000000000 ) ) ;
#97859=CYLINDRICAL_SURFACE ( 'NONE', #209362, 0.1000000000000028644 ) ;
#97865=VECTOR ( 'NONE', #192552, 999.9999999999998863 ) ;
#97903=AXIS2_PLACEMENT_3D ( 'NONE', #51599, #90746, #54194 ) ;
#97906=CARTESIAN_POINT ( 'NONE',  ( 11.60000000000006004, 67.65000000001118963, -25.06452884076210097 ) ) ;
#97934=EDGE_LOOP ( 'NONE', ( #138646, #50732, #241177, #34751 ) ) ;
#97944=CYLINDRICAL_SURFACE ( 'NONE', #32636, 0.09999999999999982514 ) ;
#97946=ADVANCED_FACE ( 'NONE', ( #72996 ), #252870, .F. ) ;
#97999=DIRECTION ( 'NONE',  ( 0.000000000000000000, 1.000000000000000000, 0.000000000000000000 ) ) ;
#98035=FACE_OUTER_BOUND ( 'NONE', #71073, .T. ) ;
#98079=CARTESIAN_POINT ( 'NONE',  ( 21.15000000000005187, 77.75000000001119815, -47.64205752314703801 ) ) ;
#98085=ORIENTED_EDGE ( 'NONE', *, *, #91788, .T. ) ;
#98124=EDGE_LOOP ( 'NONE', ( #93228, #11093, #234433, #9479 ) ) ;
#98133=DIRECTION ( 'NONE',  ( -1.000000000000000000, -0.000000000000000000, -0.000000000000000000 ) ) ;
#98141=AXIS2_PLACEMENT_3D ( 'NONE', #85655, #222615, #218774 ) ;
#98177=VECTOR ( 'NONE', #153552, 1000.000000000000000 ) ;
#98219=EDGE_LOOP ( 'NONE', ( #55918, #214532, #225337, #168650 ) ) ;
#98263=ORIENTED_EDGE ( 'NONE', *, *, #42241, .T. ) ;
#98305=EDGE_CURVE ( 'NONE', #50040, #88829, #72675, .T. ) ;
#98315=ORIENTED_EDGE ( 'NONE', *, *, #157477, .T. ) ;
#98346=EDGE_CURVE ( 'NONE', #69129, #103163, #191342, .T. ) ;
#98391=ADVANCED_FACE ( 'NONE', ( #210873 ), #196234, .T. ) ;
#98456=VERTEX_POINT ( 'NONE', #179467 ) ;
#98458=CARTESIAN_POINT ( 'NONE',  ( -21.14999999999994174, 77.83551161375991967, -47.52760213295649550 ) ) ;
#98489=ORIENTED_EDGE ( 'NONE', *, *, #82361, .F. ) ;
#98493=ORIENTED_EDGE ( 'NONE', *, *, #106482, .T. ) ;
#98533=EDGE_LOOP ( 'NONE', ( #20395, #120585, #197360, #63076 ) ) ;
#98551=DIRECTION ( 'NONE',  ( 0.000000000000000000, -1.000000000000000000, 0.000000000000000000 ) ) ;
#98590=CARTESIAN_POINT ( 'NONE',  ( 23.40000000000005187, 76.00000000001119815, -36.02310748452479316 ) ) ;
#98610=VECTOR ( 'NONE', #71694, 1000.000000000000000 ) ;
#98636=ORIENTED_EDGE ( 'NONE', *, *, #94412, .F. ) ;
#98668=DIRECTION ( 'NONE',  ( 0.000000000000000000, -1.000000000000000000, 0.000000000000000000 ) ) ;
#98672=DIRECTION ( 'NONE',  ( -0.000000000000000000, 0.000000000000000000, -1.000000000000000000 ) ) ;
#98713=DIRECTION ( 'NONE',  ( 0.000000000000000000, 0.000000000000000000, 1.000000000000000000 ) ) ;
#98729=CIRCLE ( 'NONE', #232072, 4.900000000000001243 ) ;
#98734=DIRECTION ( 'NONE',  ( -0.000000000000000000, -0.9910827722268049644, -0.1332476588733589318 ) ) ;
#98754=ADVANCED_FACE ( 'NONE', ( #35800 ), #254775, .T. ) ;
#98761=CYLINDRICAL_SURFACE ( 'NONE', #196911, 0.09999999999999982514 ) ;
#98773=EDGE_CURVE ( 'NONE', #195816, #86047, #113035, .T. ) ;
#98777=CARTESIAN_POINT ( 'NONE',  ( 20.95000000000005613, 67.65000000001118963, -3.123107484524795474 ) ) ;
#98849=ORIENTED_EDGE ( 'NONE', *, *, #154169, .T. ) ;
#98857=DIRECTION ( 'NONE',  ( 0.000000000000000000, -0.000000000000000000, 1.000000000000000000 ) ) ;
#98864=CARTESIAN_POINT ( 'NONE',  ( -6.099999999999939249, 64.35000000001120668, -22.12310748452479103 ) ) ;
#98865=ORIENTED_EDGE ( 'NONE', *, *, #210203, .F. ) ;
#98916=CARTESIAN_POINT ( 'NONE',  ( -23.49999999999994316, 74.14873292176677921, -47.62635315998165453 ) ) ;
#98956=ORIENTED_EDGE ( 'NONE', *, *, #125405, .T. ) ;
#98960=EDGE_LOOP ( 'NONE', ( #141300, #122578, #82114, #131957 ) ) ;
#99107=ADVANCED_FACE ( 'NONE', ( #57264 ), #216357, .T. ) ;
#99120=ADVANCED_FACE ( 'NONE', ( #69489 ), #15633, .F. ) ;
#99145=CARTESIAN_POINT ( 'NONE',  ( 23.40000000000005187, 74.83745509109094485, -44.02310748452479316 ) ) ;
#99157=VECTOR ( 'NONE', #47991, 1000.000000000000114 ) ;
#99163=ORIENTED_EDGE ( 'NONE', *, *, #99728, .F. ) ;
#99178=AXIS2_PLACEMENT_3D ( 'NONE', #168396, #247875, #151366 ) ;
#99221=EDGE_LOOP ( 'NONE', ( #161087, #36219, #16530, #32338 ) ) ;
#99269=ORIENTED_EDGE ( 'NONE', *, *, #67848, .F. ) ;
#99338=VERTEX_POINT ( 'NONE', #230489 ) ;
#99349=CARTESIAN_POINT ( 'NONE',  ( -23.49999999999994316, 82.72707916847673459, -26.51159310135756897 ) ) ;
#99428=ORIENTED_EDGE ( 'NONE', *, *, #105488, .F. ) ;
#99439=EDGE_CURVE ( 'NONE', #26416, #179524, #156112, .T. ) ;
#99474=DIRECTION ( 'NONE',  ( -1.000000000000000000, 0.000000000000000000, 0.000000000000000000 ) ) ;
#99574=CARTESIAN_POINT ( 'NONE',  ( -21.14999999999994174, 74.94272479589878344, -8.023107484524793165 ) ) ;
#99607=CIRCLE ( 'NONE', #203867, 0.09999999999999939493 ) ;
#99616=DIRECTION ( 'NONE',  ( -1.000000000000000000, -0.000000000000000000, -0.000000000000000000 ) ) ;
#99644=EDGE_CURVE ( 'NONE', #116777, #32708, #257682, .T. ) ;
#99660=CARTESIAN_POINT ( 'NONE',  ( -23.49999999999994316, 73.94408376456904364, -49.16694968567509250 ) ) ;
#99668=DIRECTION ( 'NONE',  ( 0.000000000000000000, 0.1332476588733589318, -0.9910827722268049644 ) ) ;
#99706=CARTESIAN_POINT ( 'NONE',  ( -23.49999999999994316, 84.00000000001119815, -34.86056257560453986 ) ) ;
#99715=ORIENTED_EDGE ( 'NONE', *, *, #239154, .F. ) ;
#99728=EDGE_CURVE ( 'NONE', #50347, #109860, #89358, .T. ) ;
#99739=CIRCLE ( 'NONE', #187095, 0.09999999999999939493 ) ;
#99818=CARTESIAN_POINT ( 'NONE',  ( 5.900000000000059863, 64.35000000001120668, -26.02310748452479316 ) ) ;
#99821=ORIENTED_EDGE ( 'NONE', *, *, #65252, .F. ) ;
#99842=VERTEX_POINT ( 'NONE', #74977 ) ;
#99862=EDGE_CURVE ( 'NONE', #30250, #23611, #21285, .T. ) ;
#99881=DIRECTION ( 'NONE',  ( -1.000000000000000000, -0.000000000000000000, -0.000000000000000000 ) ) ;
#99929=CIRCLE ( 'NONE', #182815, 0.09999999999999939493 ) ;
#99980=EDGE_CURVE ( 'NONE', #116777, #105984, #4835, .T. ) ;
#99990=PLANE ( 'NONE',  #170621 ) ;
#100030=CARTESIAN_POINT ( 'NONE',  ( -21.14999999999994174, 87.50449464844290048, -34.18759587077607165 ) ) ;
#100065=ORIENTED_EDGE ( 'NONE', *, *, #45799, .T. ) ;
#100143=DIRECTION ( 'NONE',  ( 0.000000000000000000, -1.000000000000000000, 0.000000000000000000 ) ) ;
#100161=LINE ( 'NONE', #179745, #43334 ) ;
#100172=ORIENTED_EDGE ( 'NONE', *, *, #35004, .F. ) ;
#100189=VERTEX_POINT ( 'NONE', #108634 ) ;
#100201=ADVANCED_FACE ( 'NONE', ( #107342 ), #233997, .F. ) ;
#100217=DIRECTION ( 'NONE',  ( -5.778696049164428005E-16, -0.1332476588733650935, 0.9910827722268042983 ) ) ;
#100220=ORIENTED_EDGE ( 'NONE', *, *, #187011, .F. ) ;
#100311=ORIENTED_EDGE ( 'NONE', *, *, #164789, .F. ) ;
#100375=DIRECTION ( 'NONE',  ( -1.000000000000000000, 0.000000000000000000, 0.000000000000000000 ) ) ;
#100382=CARTESIAN_POINT ( 'NONE',  ( 21.05000000000005400, 65.25000000001119815, -3.123107484524795474 ) ) ;
#100415=CARTESIAN_POINT ( 'NONE',  ( -20.94999999999994600, 65.35000000001120668, -4.423107484524790856 ) ) ;
#100424=CARTESIAN_POINT ( 'NONE',  ( -21.14999999999994174, 79.78873604695631627, -7.297728304630792806 ) ) ;
#100434=AXIS2_PLACEMENT_3D ( 'NONE', #253317, #51243, #169986 ) ;
#100522=DIRECTION ( 'NONE',  ( 0.000000000000000000, 0.000000000000000000, 1.000000000000000000 ) ) ;
#100536=ORIENTED_EDGE ( 'NONE', *, *, #255632, .T. ) ;
#100553=ADVANCED_FACE ( 'NONE', ( #80758 ), #203296, .T. ) ;
#100690=ADVANCED_FACE ( 'NONE', ( #169019 ), #221692, .F. ) ;
#100694=ORIENTED_EDGE ( 'NONE', *, *, #122302, .F. ) ;
#100708=DIRECTION ( 'NONE',  ( -1.000000000000000000, 0.000000000000000000, 0.000000000000000000 ) ) ;
#100739=CYLINDRICAL_SURFACE ( 'NONE', #231118, 0.1000000000000002554 ) ;
#100773=CIRCLE ( 'NONE', #254877, 0.1000000000000032391 ) ;
#100788=ORIENTED_EDGE ( 'NONE', *, *, #60527, .T. ) ;
#100832=DIRECTION ( 'NONE',  ( 1.000000000000000000, 0.000000000000000000, 0.000000000000000000 ) ) ;
#100834=CARTESIAN_POINT ( 'NONE',  ( -23.39999999999994529, 79.78873604695631627, -7.297728304630792806 ) ) ;
#100852=ADVANCED_FACE ( 'NONE', ( #120582 ), #159200, .T. ) ;
#100935=EDGE_CURVE ( 'NONE', #250992, #173183, #176138, .T. ) ;
#100939=CARTESIAN_POINT ( 'NONE',  ( -11.59999999999994458, 64.35000000001120668, -21.02310748452479316 ) ) ;
#100981=ORIENTED_EDGE ( 'NONE', *, *, #65270, .F. ) ;
#101000=ORIENTED_EDGE ( 'NONE', *, *, #126415, .T. ) ;
#101028=VERTEX_POINT ( 'NONE', #91710 ) ;
#101048=AXIS2_PLACEMENT_3D ( 'NONE', #138784, #39761, #179269 ) ;
#101059=ADVANCED_FACE ( 'NONE', ( #69595 ), #217782, .T. ) ;
#101118=DIRECTION ( 'NONE',  ( 0.000000000000000000, -0.000000000000000000, 1.000000000000000000 ) ) ;
#101123=ADVANCED_FACE ( 'NONE', ( #134659 ), #158149, .T. ) ;
#101148=DIRECTION ( 'NONE',  ( 1.000000000000000000, 0.000000000000000000, 0.000000000000000000 ) ) ;
#101200=DIRECTION ( 'NONE',  ( 0.000000000000000000, 0.9910827722268049644, 0.1332476588733589318 ) ) ;
#101231=DIRECTION ( 'NONE',  ( 0.000000000000000000, 0.000000000000000000, -1.000000000000000000 ) ) ;
#101234=LINE ( 'NONE', #180836, #21517 ) ;
#101256=CIRCLE ( 'NONE', #72110, 0.1999999999999987899 ) ;
#101263=AXIS2_PLACEMENT_3D ( 'NONE', #13672, #228876, #233996 ) ;
#101275=VECTOR ( 'NONE', #228943, 1000.000000000000000 ) ;
#101305=DIRECTION ( 'NONE',  ( 0.000000000000000000, -0.000000000000000000, -1.000000000000000000 ) ) ;
#101311=DIRECTION ( 'NONE',  ( 0.000000000000000000, -0.4856429311786307768, -0.8741572761215384846 ) ) ;
#101324=ORIENTED_EDGE ( 'NONE', *, *, #95561, .T. ) ;
#101328=VECTOR ( 'NONE', #109443, 1000.000000000000114 ) ;
#101365=ORIENTED_EDGE ( 'NONE', *, *, #177242, .T. ) ;
#101387=DIRECTION ( 'NONE',  ( 1.000000000000000000, -0.000000000000000000, -0.000000000000000000 ) ) ;
#101397=EDGE_CURVE ( 'NONE', #103754, #139562, #249202, .T. ) ;
#101460=DIRECTION ( 'NONE',  ( 0.000000000000000000, -1.000000000000000000, 0.000000000000000000 ) ) ;
#101513=LINE ( 'NONE', #181113, #146691 ) ;
#101546=FACE_OUTER_BOUND ( 'NONE', #22425, .T. ) ;
#101565=EDGE_LOOP ( 'NONE', ( #69111, #33665, #127561, #251170 ) ) ;
#101591=ORIENTED_EDGE ( 'NONE', *, *, #169316, .T. ) ;
#101609=DIRECTION ( 'NONE',  ( 0.000000000000000000, 0.000000000000000000, -1.000000000000000000 ) ) ;
#101610=AXIS2_PLACEMENT_3D ( 'NONE', #76857, #134254, #57278 ) ;
#101664=TOROIDAL_SURFACE ( 'NONE', #51585, 0.2000000000000000111, 0.1000000000000000056 ) ;
#101697=ADVANCED_FACE ( 'NONE', ( #22153 ), #59948, .F. ) ;
#101699=FACE_OUTER_BOUND ( 'NONE', #126801, .T. ) ;
#101713=CIRCLE ( 'NONE', #226632, 0.1000000000000028644 ) ;
#101733=AXIS2_PLACEMENT_3D ( 'NONE', #235227, #161819, #77414 ) ;
#101824=ORIENTED_EDGE ( 'NONE', *, *, #50686, .T. ) ;
#101828=EDGE_LOOP ( 'NONE', ( #54299, #101824, #99428 ) ) ;
#101837=DIRECTION ( 'NONE',  ( -1.000000000000000000, 0.000000000000000000, 0.000000000000000000 ) ) ;
#101885=AXIS2_PLACEMENT_3D ( 'NONE', #220550, #241406, #199723 ) ;
#101942=ORIENTED_EDGE ( 'NONE', *, *, #1673, .F. ) ;
#101954=DIRECTION ( 'NONE',  ( -1.000000000000000000, -0.000000000000000000, -0.000000000000000000 ) ) ;
#101958=ADVANCED_FACE ( 'NONE', ( #191509 ), #22385, .T. ) ;
#102020=CARTESIAN_POINT ( 'NONE',  ( -5.899999999999938183, 64.65000000001120384, -25.92310748452479174 ) ) ;
#102038=CARTESIAN_POINT ( 'NONE',  ( 13.40000000000005898, 64.35000000001120668, -23.72310748452479601 ) ) ;
#102045=LINE ( 'NONE', #163342, #101328 ) ;
#102231=ADVANCED_FACE ( 'NONE', ( #149490 ), #188583, .F. ) ;
#102235=CIRCLE ( 'NONE', #98141, 0.1000000000000002554 ) ;
#102242=CARTESIAN_POINT ( 'NONE',  ( 20.95000000000005613, 67.85000000001119247, -3.023107484524792277 ) ) ;
#102247=AXIS2_PLACEMENT_3D ( 'NONE', #147697, #142541, #181691 ) ;
#102390=AXIS2_PLACEMENT_3D ( 'NONE', #189178, #110915, #11846 ) ;
#102407=AXIS2_PLACEMENT_3D ( 'NONE', #10351, #169449, #91151 ) ;
#102439=DIRECTION ( 'NONE',  ( -0.000000000000000000, 1.000000000000000000, 1.734723475976757554E-14 ) ) ;
#102446=EDGE_LOOP ( 'NONE', ( #50820, #77442, #238761, #122430 ) ) ;
#102461=CIRCLE ( 'NONE', #248256, 0.1000000000000021844 ) ;
#102463=FACE_OUTER_BOUND ( 'NONE', #10610, .T. ) ;
#102474=EDGE_CURVE ( 'NONE', #90293, #230635, #126955, .T. ) ;
#102516=ORIENTED_EDGE ( 'NONE', *, *, #228592, .F. ) ;
#102544=CARTESIAN_POINT ( 'NONE',  ( 13.40000000000005898, 67.72071067812984779, -21.02310748452479316 ) ) ;
#102700=CARTESIAN_POINT ( 'NONE',  ( -40.23850191057533010, 65.35000000001120668, -4.423107484524790856 ) ) ;
#102703=TOROIDAL_SURFACE ( 'NONE', #94528, 2.699999999999999734, 0.1000000000000000056 ) ;
#102749=CIRCLE ( 'NONE', #181891, 0.09999999999999939493 ) ;
#102767=LINE ( 'NONE', #243588, #103412 ) ;
#102856=DIRECTION ( 'NONE',  ( 0.000000000000000000, 0.000000000000000000, -1.000000000000000000 ) ) ;
#102864=AXIS2_PLACEMENT_3D ( 'NONE', #33018, #192061, #172530 ) ;
#102907=AXIS2_PLACEMENT_3D ( 'NONE', #81270, #180406, #23924 ) ;
#102929=AXIS2_PLACEMENT_3D ( 'NONE', #102700, #44044, #165269 ) ;
#102971=CARTESIAN_POINT ( 'NONE',  ( 23.40000000000005187, 82.84256550613280012, -26.34830530078816935 ) ) ;
#103000=AXIS2_PLACEMENT_3D ( 'NONE', #157667, #179768, #177217 ) ;
#103008=CARTESIAN_POINT ( 'NONE',  ( 21.15000000000005542, 83.90000000001120384, -34.86056257560453986 ) ) ;
#103014=ORIENTED_EDGE ( 'NONE', *, *, #23722, .F. ) ;
#103057=EDGE_LOOP ( 'NONE', ( #133067, #219748, #209063, #27561 ) ) ;
#103076=ORIENTED_EDGE ( 'NONE', *, *, #1262, .T. ) ;
#103083=ORIENTED_EDGE ( 'NONE', *, *, #256079, .F. ) ;
#103123=EDGE_CURVE ( 'NONE', #253828, #224235, #135314, .T. ) ;
#103124=VECTOR ( 'NONE', #73212, 1000.000000000000000 ) ;
#103153=VECTOR ( 'NONE', #158993, 1000.000000000000000 ) ;
#103160=AXIS2_PLACEMENT_3D ( 'NONE', #22750, #124404, #167400 ) ;
#103163=VERTEX_POINT ( 'NONE', #235761 ) ;
#103180=SPHERICAL_SURFACE ( 'NONE', #12240, 0.1000000000000000056 ) ;
#103257=ORIENTED_EDGE ( 'NONE', *, *, #71125, .T. ) ;
#103283=EDGE_CURVE ( 'NONE', #202553, #184620, #84342, .T. ) ;
#103403=LINE ( 'NONE', #182983, #15464 ) ;
#103408=AXIS2_PLACEMENT_3D ( 'NONE', #179955, #2571, #216495 ) ;
#103412=VECTOR ( 'NONE', #147039, 1000.000000000000000 ) ;
#103436=CARTESIAN_POINT ( 'NONE',  ( -23.39999999999994529, 64.35000000001120668, -36.02310748452479316 ) ) ;
#103437=ORIENTED_EDGE ( 'NONE', *, *, #234884, .T. ) ;
#103481=LINE ( 'NONE', #185612, #124472 ) ;
#103500=AXIS2_PLACEMENT_3D ( 'NONE', #35094, #115876, #75490 ) ;
#103517=DIRECTION ( 'NONE',  ( 0.000000000000000000, 0.000000000000000000, -1.000000000000000000 ) ) ;
#103530=CARTESIAN_POINT ( 'NONE',  ( -23.49999999999994316, 77.75000000001119815, -47.64205752314703801 ) ) ;
#103597=DIRECTION ( 'NONE',  ( 0.000000000000000000, 0.000000000000000000, -1.000000000000000000 ) ) ;
#103616=CIRCLE ( 'NONE', #61957, 0.1000000000000032391 ) ;
#103703=CARTESIAN_POINT ( 'NONE',  ( 11.60000000000006182, 67.75000000001118394, -23.62310748452479103 ) ) ;
#103749=VECTOR ( 'NONE', #232837, 1000.000000000000000 ) ;
#103754=VERTEX_POINT ( 'NONE', #120678 ) ;
#103767=EDGE_LOOP ( 'NONE', ( #175686, #195418, #96065, #109492 ) ) ;
#103781=CARTESIAN_POINT ( 'NONE',  ( 23.40000000000005542, 82.64476912853859858, -26.37791261425322986 ) ) ;
#103784=DIRECTION ( 'NONE',  ( 0.000000000000000000, 0.000000000000000000, 1.000000000000000000 ) ) ;
#103919=ADVANCED_FACE ( 'NONE', ( #76077 ), #12281, .F. ) ;
#103920=CARTESIAN_POINT ( 'NONE',  ( 23.50000000000005684, 74.83745509109094485, -44.02310748452479316 ) ) ;
#103933=CARTESIAN_POINT ( 'NONE',  ( -21.04999999999994387, 65.25000000001119815, -3.123107484524795474 ) ) ;
#103942=CARTESIAN_POINT ( 'NONE',  ( -0.8999999999999437339, 67.65000000001118963, -10.02310748452479139 ) ) ;
#104006=ORIENTED_EDGE ( 'NONE', *, *, #228592, .T. ) ;
#104035=CYLINDRICAL_SURFACE ( 'NONE', #247782, 11.74999999999999645 ) ;
#104090=EDGE_LOOP ( 'NONE', ( #256509, #218447, #174574, #215189 ) ) ;
#104103=LINE ( 'NONE', #183678, #228028 ) ;
#104142=EDGE_CURVE ( 'NONE', #249282, #144177, #114287, .T. ) ;
#104144=ORIENTED_EDGE ( 'NONE', *, *, #205065, .F. ) ;
#104184=CARTESIAN_POINT ( 'NONE',  ( 21.15000000000005187, 74.16448838626247664, -47.62760213295649692 ) ) ;
#104194=CARTESIAN_POINT ( 'NONE',  ( -21.14999999999994174, 83.98667523412385094, -37.28476067066772970 ) ) ;
#104196=VECTOR ( 'NONE', #97771, 1000.000000000000000 ) ;
#104351=VERTEX_POINT ( 'NONE', #37338 ) ;
#104356=DIRECTION ( 'NONE',  ( -0.000000000000000000, -0.000000000000000000, -1.000000000000000000 ) ) ;
#104462=DIRECTION ( 'NONE',  ( 0.000000000000000000, -0.9910827722268049644, -0.1332476588733589318 ) ) ;
#104486=DIRECTION ( 'NONE',  ( 1.000000000000000000, 0.000000000000000000, 0.000000000000000000 ) ) ;
#104496=DIRECTION ( 'NONE',  ( 0.000000000000000000, -0.000000000000000000, 1.000000000000000000 ) ) ;
#104499=VERTEX_POINT ( 'NONE', #45025 ) ;
#104595=CARTESIAN_POINT ( 'NONE',  ( 13.40000000000005898, 67.65000000001120384, -16.98168612828748891 ) ) ;
#104698=CIRCLE ( 'NONE', #167311, 0.09999999999999939493 ) ;
#104705=CARTESIAN_POINT ( 'NONE',  ( 23.40000000000005542, 83.98667523412385094, -34.76145429838185663 ) ) ;
#104775=EDGE_LOOP ( 'NONE', ( #176952, #122705, #197281, #23643 ) ) ;
#104791=DIRECTION ( 'NONE',  ( 0.000000000000000000, 0.000000000000000000, 1.000000000000000000 ) ) ;
#104825=FACE_OUTER_BOUND ( 'NONE', #130930, .T. ) ;
#104887=CYLINDRICAL_SURFACE ( 'NONE', #217531, 0.1000000000000021844 ) ;
#104892=CARTESIAN_POINT ( 'NONE',  ( -21.14999999999994174, 87.60324567546805952, -37.87437456276921210 ) ) ;
#104894=ORIENTED_EDGE ( 'NONE', *, *, #247672, .T. ) ;
#104899=ORIENTED_EDGE ( 'NONE', *, *, #197515, .F. ) ;
#104901=CARTESIAN_POINT ( 'NONE',  ( 21.15000000000005542, 65.15000000001120384, -3.123107484524795474 ) ) ;
#104996=CYLINDRICAL_SURFACE ( 'NONE', #62235, 0.1000000000000021844 ) ;
#105077=DIRECTION ( 'NONE',  ( 0.000000000000000000, 0.9910827722268049644, -0.1332476588733589318 ) ) ;
#105081=LINE ( 'NONE', #8596, #129560 ) ;
#105110=AXIS2_PLACEMENT_3D ( 'NONE', #109364, #53268, #93670 ) ;
#105117=CARTESIAN_POINT ( 'NONE',  ( 23.50000000000005684, 74.63923853664559260, -43.99645795275012006 ) ) ;
#105236=VECTOR ( 'NONE', #251514, 1000.000000000000000 ) ;
#105270=AXIS2_PLACEMENT_3D ( 'NONE', #132903, #212445, #36386 ) ;
#105281=ORIENTED_EDGE ( 'NONE', *, *, #63228, .F. ) ;
#105304=FACE_OUTER_BOUND ( 'NONE', #118201, .T. ) ;
#105374=CARTESIAN_POINT ( 'NONE',  ( 23.50000000000005684, 66.40137734081807253, -35.02137779515522453 ) ) ;
#105468=VECTOR ( 'NONE', #130940, 1000.000000000000000 ) ;
#105488=EDGE_CURVE ( 'NONE', #161116, #113073, #27931, .T. ) ;
#105514=ORIENTED_EDGE ( 'NONE', *, *, #212514, .F. ) ;
#105529=DIRECTION ( 'NONE',  ( 1.000000000000000000, -0.000000000000000000, 0.000000000000000000 ) ) ;
#105649=CIRCLE ( 'NONE', #76629, 0.1000000000000028644 ) ;
#105737=CARTESIAN_POINT ( 'NONE',  ( -21.14999999999994174, 74.16448838626247664, -47.52760213295649550 ) ) ;
#105775=EDGE_CURVE ( 'NONE', #119358, #121523, #252928, .T. ) ;
#105807=CYLINDRICAL_SURFACE ( 'NONE', #84170, 0.09999999999999939493 ) ;
#105895=AXIS2_PLACEMENT_3D ( 'NONE', #29728, #229188, #130061 ) ;
#105945=EDGE_LOOP ( 'NONE', ( #228120, #165357, #2337, #121881 ) ) ;
#105962=CARTESIAN_POINT ( 'NONE',  ( -21.14999999999994174, 76.00000000001119815, -36.02310748452479316 ) ) ;
#105984=VERTEX_POINT ( 'NONE', #232412 ) ;
#105986=FACE_OUTER_BOUND ( 'NONE', #49258, .T. ) ;
#105988=CIRCLE ( 'NONE', #189233, 0.09999999999999939493 ) ;
#106018=CARTESIAN_POINT ( 'NONE',  ( 21.05000000000005400, 67.75000000001118394, -3.123107484524795474 ) ) ;
#106064=DIRECTION ( 'NONE',  ( 0.000000000000000000, 0.000000000000000000, 1.000000000000000000 ) ) ;
#106099=DIRECTION ( 'NONE',  ( 0.000000000000000000, -1.000000000000000000, 0.000000000000000000 ) ) ;
#106277=LINE ( 'NONE', #25495, #91044 ) ;
#106288=CARTESIAN_POINT ( 'NONE',  ( -23.49999999999994316, 76.00000000001119815, -36.02310748452479316 ) ) ;
#106353=CARTESIAN_POINT ( 'NONE',  ( -21.04999999999994387, 65.35000000001120668, -4.423107484524790856 ) ) ;
#106412=CIRCLE ( 'NONE', #193938, 0.09999999999999530098 ) ;
#106416=CARTESIAN_POINT ( 'NONE',  ( 20.95000000000005258, 66.15000000001120384, -4.623107484524796362 ) ) ;
#106482=EDGE_CURVE ( 'NONE', #134658, #115551, #144952, .T. ) ;
#106582=CARTESIAN_POINT ( 'NONE',  ( -21.04999999999994387, 82.72707916847673459, -26.51159310135756897 ) ) ;
#106594=ORIENTED_EDGE ( 'NONE', *, *, #153983, .T. ) ;
#106718=DIRECTION ( 'NONE',  ( 1.000000000000000000, -0.000000000000000000, -0.000000000000000000 ) ) ;
#106725=CARTESIAN_POINT ( 'NONE',  ( -21.14999999999994174, 82.78482233730476025, -26.42994920107286916 ) ) ;
#106728=EDGE_CURVE ( 'NONE', #56891, #89909, #171840, .T. ) ;
#106733=DIRECTION ( 'NONE',  ( -1.000000000000000000, 0.000000000000000000, 0.000000000000000000 ) ) ;
#106776=DIRECTION ( 'NONE',  ( 0.000000000000000000, 0.000000000000000000, 1.000000000000000000 ) ) ;
#106794=VERTEX_POINT ( 'NONE', #14023 ) ;
#106796=VERTEX_POINT ( 'NONE', #93539 ) ;
#106851=( NAMED_UNIT ( * ) PLANE_ANGLE_UNIT ( ) SI_UNIT ( $, .RADIAN. ) );
#106866=CARTESIAN_POINT ( 'NONE',  ( -20.94999999999994600, 65.19115966511134275, -29.92310748452479174 ) ) ;
#106876=DIRECTION ( 'NONE',  ( 0.000000000000000000, -1.000000000000000000, 0.000000000000000000 ) ) ;
#106886=EDGE_CURVE ( 'NONE', #6487, #249282, #186860, .T. ) ;
#106897=ORIENTED_EDGE ( 'NONE', *, *, #151172, .T. ) ;
#106900=ORIENTED_EDGE ( 'NONE', *, *, #256781, .F. ) ;
#106914=ORIENTED_EDGE ( 'NONE', *, *, #115178, .T. ) ;
#106977=ORIENTED_EDGE ( 'NONE', *, *, #163938, .F. ) ;
#107047=ORIENTED_EDGE ( 'NONE', *, *, #155750, .F. ) ;
#107182=ORIENTED_EDGE ( 'NONE', *, *, #79816, .T. ) ;
#107241=DIRECTION ( 'NONE',  ( -1.000000000000000000, -0.000000000000000000, 0.000000000000000000 ) ) ;
#107252=DIRECTION ( 'NONE',  ( 0.000000000000000000, 0.000000000000000000, 1.000000000000000000 ) ) ;
#107280=EDGE_CURVE ( 'NONE', #119288, #62069, #45779, .T. ) ;
#107292=DIRECTION ( 'NONE',  ( 0.000000000000000000, -1.000000000000000000, -0.000000000000000000 ) ) ;
#107323=AXIS2_PLACEMENT_3D ( 'NONE', #160016, #80411, #37494 ) ;
#107342=FACE_OUTER_BOUND ( 'NONE', #39793, .T. ) ;
#107412=DIRECTION ( 'NONE',  ( 0.000000000000000000, 1.000000000000000000, -0.000000000000000000 ) ) ;
#107420=CARTESIAN_POINT ( 'NONE',  ( 21.15000000000005542, 83.80000000001119531, -37.18565239344504647 ) ) ;
#107438=ORIENTED_EDGE ( 'NONE', *, *, #98305, .T. ) ;
#107494=FACE_OUTER_BOUND ( 'NONE', #152561, .T. ) ;
#107500=CIRCLE ( 'NONE', #157623, 0.1999999999999987899 ) ;
#107562=ORIENTED_EDGE ( 'NONE', *, *, #86271, .F. ) ;
#107579=EDGE_CURVE ( 'NONE', #226270, #80879, #126225, .T. ) ;
#107632=LINE ( 'NONE', #88044, #88833 ) ;
#107651=VERTEX_POINT ( 'NONE', #144490 ) ;
#107698=DIRECTION ( 'NONE',  ( -0.000000000000000000, -0.9875102702516472819, 0.1575546449569748542 ) ) ;
#107723=DIRECTION ( 'NONE',  ( 0.000000000000000000, 0.000000000000000000, 1.000000000000000000 ) ) ;
#107731=AXIS2_PLACEMENT_3D ( 'NONE', #182155, #124748, #123459 ) ;
#107745=CARTESIAN_POINT ( 'NONE',  ( -21.14999999999994174, 87.51781941433023349, -34.28670414799875488 ) ) ;
#107748=CARTESIAN_POINT ( 'NONE',  ( -23.39999999999994529, 64.35000000001120668, -3.123107484524795474 ) ) ;
#107769=EDGE_CURVE ( 'NONE', #80585, #74170, #75283, .T. ) ;
#107780=UNCERTAINTY_MEASURE_WITH_UNIT (LENGTH_MEASURE( 1.000000000000000082E-05 ), #44766, 'distance_accuracy_value', 'NONE');
#107789=VERTEX_POINT ( 'NONE', #230475 ) ;
#107798=DIRECTION ( 'NONE',  ( 0.000000000000000000, -1.000000000000000000, 0.000000000000000000 ) ) ;
#107814=ORIENTED_EDGE ( 'NONE', *, *, #48843, .F. ) ;
#107837=ORIENTED_EDGE ( 'NONE', *, *, #189678, .F. ) ;
#107844=DIRECTION ( 'NONE',  ( -1.000000000000000000, -0.000000000000000000, -0.000000000000000000 ) ) ;
#107871=VECTOR ( 'NONE', #243934, 1000.000000000000000 ) ;
#107902=CARTESIAN_POINT ( 'NONE',  ( -23.39999999999994529, 77.83551161375991967, -47.52760213295649550 ) ) ;
#107974=LINE ( 'NONE', #6284, #128119 ) ;
#108027=CYLINDRICAL_SURFACE ( 'NONE', #81290, 4.049999999999998046 ) ;
#108093=CARTESIAN_POINT ( 'NONE',  ( 21.15000000000005187, 64.35000000001120668, -36.02310748452479316 ) ) ;
#108159=VERTEX_POINT ( 'NONE', #254800 ) ;
#108189=EDGE_CURVE ( 'NONE', #186109, #135540, #23717, .T. ) ;
#108207=AXIS2_PLACEMENT_3D ( 'NONE', #102242, #591, #158441 ) ;
#108239=ORIENTED_EDGE ( 'NONE', *, *, #118295, .T. ) ;
#108291=CARTESIAN_POINT ( 'NONE',  ( 11.60000000000006004, 67.65000000001118963, -16.98168612828748891 ) ) ;
#108437=FACE_OUTER_BOUND ( 'NONE', #213665, .T. ) ;
#108439=ORIENTED_EDGE ( 'NONE', *, *, #134347, .F. ) ;
#108446=EDGE_CURVE ( 'NONE', #53024, #253379, #249434, .T. ) ;
#108448=DIRECTION ( 'NONE',  ( 0.000000000000000000, 0.000000000000000000, 1.000000000000000000 ) ) ;
#108461=CARTESIAN_POINT ( 'NONE',  ( -5.899999999999938183, 64.35000000001120668, -26.12310748452479103 ) ) ;
#108478=CARTESIAN_POINT ( 'NONE',  ( -23.49999999999994316, 87.50449464844290048, -34.18759587077607165 ) ) ;
#108525=EDGE_CURVE ( 'NONE', #133332, #39283, #215224, .T. ) ;
#108534=ORIENTED_EDGE ( 'NONE', *, *, #140601, .F. ) ;
#108578=AXIS2_PLACEMENT_3D ( 'NONE', #154759, #109169, #233012 ) ;
#108588=PRESENTATION_STYLE_ASSIGNMENT (( #46036 ) ) ;
#108597=DIRECTION ( 'NONE',  ( 0.000000000000000000, 0.000000000000000000, 1.000000000000000000 ) ) ;
#108634=CARTESIAN_POINT ( 'NONE',  ( 13.40000000000005898, 64.35000000001120668, -18.42310748452479530 ) ) ;
#108748=CARTESIAN_POINT ( 'NONE',  ( 21.05000000000005400, 64.35000000001119247, -6.023107484524794941 ) ) ;
#108751=EDGE_CURVE ( 'NONE', #139562, #231379, #136256, .T. ) ;
#108761=ADVANCED_FACE ( 'NONE', ( #184970 ), #165416, .T. ) ;
#108766=DIRECTION ( 'NONE',  ( 0.000000000000000000, 0.000000000000000000, -1.000000000000000000 ) ) ;
#108816=DIRECTION ( 'NONE',  ( -0.000000000000000000, 1.000000000000000000, -0.000000000000000000 ) ) ;
#108837=CARTESIAN_POINT ( 'NONE',  ( 13.40000000000005898, 67.75000000001118394, -23.62310748452479103 ) ) ;
#108845=ORIENTED_EDGE ( 'NONE', *, *, #204047, .F. ) ;
#108850=ADVANCED_FACE ( 'NONE', ( #54436 ), #195266, .T. ) ;
#108924=TOROIDAL_SURFACE ( 'NONE', #188058, 4.900000000000000355, 0.1000000000000000056 ) ;
#108943=ORIENTED_EDGE ( 'NONE', *, *, #144705, .F. ) ;
#108946=DIRECTION ( 'NONE',  ( 1.000000000000000000, 0.000000000000000000, 0.000000000000000000 ) ) ;
#108951=DIRECTION ( 'NONE',  ( 0.000000000000000000, 0.9910827722268055195, -0.1332476588733540468 ) ) ;
#108972=ORIENTED_EDGE ( 'NONE', *, *, #204974, .T. ) ;
#108990=ORIENTED_EDGE ( 'NONE', *, *, #40549, .F. ) ;
#109039=VERTEX_POINT ( 'NONE', #3438 ) ;
#109060=DIRECTION ( 'NONE',  ( 0.000000000000000000, 0.000000000000000000, -1.000000000000000000 ) ) ;
#109112=EDGE_CURVE ( 'NONE', #99842, #107651, #169841, .T. ) ;
#109169=DIRECTION ( 'NONE',  ( 0.000000000000000000, 1.000000000000000000, -0.000000000000000000 ) ) ;
#109225=DIRECTION ( 'NONE',  ( 0.000000000000000000, 0.000000000000000000, -1.000000000000000000 ) ) ;
#109234=VERTEX_POINT ( 'NONE', #93249 ) ;
#109247=FACE_OUTER_BOUND ( 'NONE', #41167, .T. ) ;
#109257=CARTESIAN_POINT ( 'NONE',  ( 0.9000000000000547562, 66.35000000001119247, -10.02310748452479139 ) ) ;
#109262=DIRECTION ( 'NONE',  ( -1.000000000000000000, 0.000000000000000000, 0.000000000000000000 ) ) ;
#109291=TOROIDAL_SURFACE ( 'NONE', #254976, 0.2000000000000000111, 0.1000000000000000056 ) ;
#109357=AXIS2_PLACEMENT_3D ( 'NONE', #45146, #105077, #184649 ) ;
#109364=CARTESIAN_POINT ( 'NONE',  ( 11.60000000000006004, 67.75000000001118394, -21.02310748452479316 ) ) ;
#109373=DIRECTION ( 'NONE',  ( 0.000000000000000000, 0.000000000000000000, 1.000000000000000000 ) ) ;
#109376=LINE ( 'NONE', #188937, #237339 ) ;
#109379=AXIS2_PLACEMENT_3D ( 'NONE', #190251, #93701, #195399 ) ;
#109400=CIRCLE ( 'NONE', #67908, 0.1000000000000016709 ) ;
#109417=CARTESIAN_POINT ( 'NONE',  ( -5.899999999999938183, 64.35000000001120668, -22.12310748452479103 ) ) ;
#109422=AXIS2_PLACEMENT_3D ( 'NONE', #17859, #218622, #846 ) ;
#109443=DIRECTION ( 'NONE',  ( -0.000000000000000000, -0.1332476588733589318, 0.9910827722268049644 ) ) ;
#109492=ORIENTED_EDGE ( 'NONE', *, *, #199839, .T. ) ;
#109600=VECTOR ( 'NONE', #85673, 1000.000000000000000 ) ;
#109651=DIRECTION ( 'NONE',  ( 0.000000000000000000, 0.000000000000000000, 1.000000000000000000 ) ) ;
#109761=DIRECTION ( 'NONE',  ( 0.000000000000000000, -0.9910827722268055195, -0.1332476588733540468 ) ) ;
#109797=VERTEX_POINT ( 'NONE', #96768 ) ;
#109839=AXIS2_PLACEMENT_3D ( 'NONE', #16389, #136285, #60617 ) ;
#109841=AXIS2_PLACEMENT_3D ( 'NONE', #108461, #238006, #47174 ) ;
#109860=VERTEX_POINT ( 'NONE', #204872 ) ;
#109969=DIRECTION ( 'NONE',  ( 0.000000000000000000, 0.9910827722268049644, 0.1332476588733589318 ) ) ;
#110027=ORIENTED_EDGE ( 'NONE', *, *, #256458, .T. ) ;
#110057=AXIS2_PLACEMENT_3D ( 'NONE', #179332, #37248, #197575 ) ;
#110082=DIRECTION ( 'NONE',  ( 0.000000000000000000, 0.000000000000000000, -1.000000000000000000 ) ) ;
#110121=CARTESIAN_POINT ( 'NONE',  ( 21.05000000000005400, 64.35000000001120668, -3.123107484524795474 ) ) ;
#110149=EDGE_CURVE ( 'NONE', #161732, #144437, #84583, .T. ) ;
#110166=DIRECTION ( 'NONE',  ( 0.000000000000000000, -1.000000000000000000, 0.000000000000000000 ) ) ;
#110203=ORIENTED_EDGE ( 'NONE', *, *, #55209, .T. ) ;
#110240=ORIENTED_EDGE ( 'NONE', *, *, #116945, .F. ) ;
#110365=CARTESIAN_POINT ( 'NONE',  ( -21.04999999999994387, 87.50449464844290048, -37.85861909827351468 ) ) ;
#110382=DIRECTION ( 'NONE',  ( -1.000000000000000000, -0.000000000000000000, -0.000000000000000000 ) ) ;
#110395=CARTESIAN_POINT ( 'NONE',  ( -20.94999999999994600, 64.25000000001119815, -29.92310748452479174 ) ) ;
#110413=CARTESIAN_POINT ( 'NONE',  ( 20.95000000000005258, 64.35000000001120668, -30.12310748452479103 ) ) ;
#110468=VERTEX_POINT ( 'NONE', #116712 ) ;
#110481=ORIENTED_EDGE ( 'NONE', *, *, #67024, .T. ) ;
#110490=DIRECTION ( 'NONE',  ( 0.000000000000000000, 0.000000000000000000, 1.000000000000000000 ) ) ;
#110537=DIRECTION ( 'NONE',  ( 1.284434275755705296E-16, -0.7071067811865471286, 0.7071067811865479058 ) ) ;
#110568=DIRECTION ( 'NONE',  ( -0.000000000000000000, 0.000000000000000000, 1.000000000000000000 ) ) ;
#110636=EDGE_CURVE ( 'NONE', #238440, #99338, #16426, .T. ) ;
#110660=CIRCLE ( 'NONE', #94084, 0.1000000000000028644 ) ;
#110669=CARTESIAN_POINT ( 'NONE',  ( -23.39999999999994529, 64.35000000001120668, -3.123107484524795474 ) ) ;
#110701=CARTESIAN_POINT ( 'NONE',  ( 5.900000000000055422, 64.75000000001119815, -36.02310748452479316 ) ) ;
#110745=DIRECTION ( 'NONE',  ( -0.000000000000000000, 1.000000000000000000, 0.000000000000000000 ) ) ;
#110783=DIRECTION ( 'NONE',  ( -0.000000000000000000, -1.000000000000000000, -0.000000000000000000 ) ) ;
#110789=ORIENTED_EDGE ( 'NONE', *, *, #202074, .T. ) ;
#110915=DIRECTION ( 'NONE',  ( 1.000000000000000000, -0.000000000000000000, 0.000000000000000000 ) ) ;
#110979=DIRECTION ( 'NONE',  ( 0.000000000000000000, 0.000000000000000000, -1.000000000000000000 ) ) ;
#111028=DIRECTION ( 'NONE',  ( 1.000000000000000000, 0.000000000000000000, -0.000000000000000000 ) ) ;
#111054=EDGE_LOOP ( 'NONE', ( #86410, #31566, #141797, #184359 ) ) ;
#111057=CARTESIAN_POINT ( 'NONE',  ( 21.15000000000005542, 78.47315729244128590, -52.27034697567518862 ) ) ;
#111099=CARTESIAN_POINT ( 'NONE',  ( -21.14999999999994174, 76.00000000001119815, -40.07310748452479032 ) ) ;
#111175=CARTESIAN_POINT ( 'NONE',  ( 20.95000000000005258, 65.25000000001119815, -4.523107484524794053 ) ) ;
#111186=CARTESIAN_POINT ( 'NONE',  ( -23.39999999999994529, 83.98667523412385094, -34.76145429838185663 ) ) ;
#111213=EDGE_LOOP ( 'NONE', ( #78263, #224290, #34545, #29901 ) ) ;
#111241=DIRECTION ( 'NONE',  ( -1.000000000000000000, -0.000000000000000000, 0.000000000000000000 ) ) ;
#111268=FACE_OUTER_BOUND ( 'NONE', #51638, .T. ) ;
#111301=CARTESIAN_POINT ( 'NONE',  ( -21.04999999999994387, 64.35000000001120668, -51.02310748452479316 ) ) ;
#111384=ORIENTED_EDGE ( 'NONE', *, *, #242263, .F. ) ;
#111420=LINE ( 'NONE', #108837, #211289 ) ;
#111553=AXIS2_PLACEMENT_3D ( 'NONE', #123009, #185541, #163416 ) ;
#111573=AXIS2_PLACEMENT_3D ( 'NONE', #241728, #61814, #141344 ) ;
#111648=ORIENTED_EDGE ( 'NONE', *, *, #25012, .F. ) ;
#111673=CARTESIAN_POINT ( 'NONE',  ( -23.49999999999994316, 64.35000000001120668, -18.32310748452479388 ) ) ;
#111710=CIRCLE ( 'NONE', #11792, 4.150000000000001243 ) ;
#111750=DIRECTION ( 'NONE',  ( 0.000000000000000000, 0.9910827722268042983, 0.1332476588733650935 ) ) ;
#111764=SPHERICAL_SURFACE ( 'NONE', #97646, 0.1000000000000000056 ) ;
#111817=CARTESIAN_POINT ( 'NONE',  ( -21.04999999999994387, 65.19115966511134275, -29.92310748452479174 ) ) ;
#111842=ORIENTED_EDGE ( 'NONE', *, *, #6491, .T. ) ;
#111848=VECTOR ( 'NONE', #81119, 1000.000000000000000 ) ;
#111921=VERTEX_POINT ( 'NONE', #69512 ) ;
#111941=DIRECTION ( 'NONE',  ( -0.000000000000000000, 0.1332476588733642331, -0.9910827722268044093 ) ) ;
#111962=VERTEX_POINT ( 'NONE', #211576 ) ;
#111988=AXIS2_PLACEMENT_3D ( 'NONE', #26285, #86217, #114802 ) ;
#112026=ORIENTED_EDGE ( 'NONE', *, *, #27624, .T. ) ;
#112028=EDGE_CURVE ( 'NONE', #81962, #238821, #229847, .T. ) ;
#112062=ORIENTED_EDGE ( 'NONE', *, *, #187011, .T. ) ;
#112068=DIRECTION ( 'NONE',  ( 0.000000000000000000, -0.000000000000000000, -1.000000000000000000 ) ) ;
#112154=ORIENTED_EDGE ( 'NONE', *, *, #171652, .F. ) ;
#112157=FACE_OUTER_BOUND ( 'NONE', #111213, .T. ) ;
#112232=DIRECTION ( 'NONE',  ( -0.000000000000000000, -0.000000000000000000, -1.000000000000000000 ) ) ;
#112274=EDGE_CURVE ( 'NONE', #110468, #147247, #79080, .T. ) ;
#112280=DIRECTION ( 'NONE',  ( -1.000000000000000000, 0.000000000000000000, -0.000000000000000000 ) ) ;
#112352=ADVANCED_FACE ( 'NONE', ( #190443 ), #31387, .F. ) ;
#112359=FACE_OUTER_BOUND ( 'NONE', #40765, .T. ) ;
#112500=ORIENTED_EDGE ( 'NONE', *, *, #246975, .F. ) ;
#112507=CARTESIAN_POINT ( 'NONE',  ( -23.49999999999994316, 77.83551161375991967, -47.62760213295649692 ) ) ;
#112566=CARTESIAN_POINT ( 'NONE',  ( 21.05000000000005400, 77.83551161375991967, -47.52760213295648839 ) ) ;
#112580=CARTESIAN_POINT ( 'NONE',  ( 20.95000000000005258, 87.75000000001122658, -30.02310748452481448 ) ) ;
#112621=EDGE_LOOP ( 'NONE', ( #98085, #28919, #6932, #191662 ) ) ;
#112626=CARTESIAN_POINT ( 'NONE',  ( -20.94999999999994245, 67.85000000001119247, -3.123107484524795474 ) ) ;
#112668=CARTESIAN_POINT ( 'NONE',  ( -23.49999999999994316, 77.73640333653723644, -47.54092689884382850 ) ) ;
#112733=EDGE_CURVE ( 'NONE', #43374, #49193, #229333, .T. ) ;
#112734=EDGE_CURVE ( 'NONE', #61669, #227850, #8561, .T. ) ;
#112766=DIRECTION ( 'NONE',  ( 0.000000000000000000, 1.000000000000000000, -0.000000000000000000 ) ) ;
#112788=VERTEX_POINT ( 'NONE', #236933 ) ;
#112857=CARTESIAN_POINT ( 'NONE',  ( 0.9000000000000547562, 67.75000000001118394, -10.02310748452479139 ) ) ;
#112959=CIRCLE ( 'NONE', #121376, 11.75000000000000000 ) ;
#112973=ORIENTED_EDGE ( 'NONE', *, *, #182245, .F. ) ;
#112980=VECTOR ( 'NONE', #26603, 1000.000000000000000 ) ;
#113016=ORIENTED_EDGE ( 'NONE', *, *, #83734, .T. ) ;
#113035=CIRCLE ( 'NONE', #146341, 0.09999999999999635569 ) ;
#113053=EDGE_CURVE ( 'NONE', #113629, #178868, #105081, .T. ) ;
#113054=ORIENTED_EDGE ( 'NONE', *, *, #105488, .T. ) ;
#113073=VERTEX_POINT ( 'NONE', #129812 ) ;
#113087=ORIENTED_EDGE ( 'NONE', *, *, #253496, .T. ) ;
#113129=DIRECTION ( 'NONE',  ( 0.000000000000000000, 1.000000000000000000, 0.000000000000000000 ) ) ;
#113156=EDGE_LOOP ( 'NONE', ( #170129, #34584, #192109, #165615 ) ) ;
#113160=DIRECTION ( 'NONE',  ( 0.000000000000000000, 0.000000000000000000, -1.000000000000000000 ) ) ;
#113240=ORIENTED_EDGE ( 'NONE', *, *, #35004, .T. ) ;
#113307=DIRECTION ( 'NONE',  ( -0.000000000000000000, -1.000000000000000000, 0.000000000000000000 ) ) ;
#113308=CARTESIAN_POINT ( 'NONE',  ( 21.05000000000005400, 65.19115966511134275, -29.92310748452479174 ) ) ;
#113360=ORIENTED_EDGE ( 'NONE', *, *, #61009, .T. ) ;
#113365=ORIENTED_EDGE ( 'NONE', *, *, #113581, .F. ) ;
#113408=ADVANCED_FACE ( 'NONE', ( #148776 ), #9244, .T. ) ;
#113461=CIRCLE ( 'NONE', #17759, 2.599999999999998312 ) ;
#113470=CARTESIAN_POINT ( 'NONE',  ( 13.40000000000005898, 67.65000000001118963, -25.06452884076209742 ) ) ;
#113474=FACE_OUTER_BOUND ( 'NONE', #42569, .T. ) ;
#113494=LINE ( 'NONE', #95215, #54836 ) ;
#113508=CARTESIAN_POINT ( 'NONE',  ( -23.39999999999994529, 74.73834681386826162, -44.00978271863746016 ) ) ;
#113520=LINE ( 'NONE', #35309, #237315 ) ;
#113548=DIRECTION ( 'NONE',  ( 0.000000000000000000, 0.000000000000000000, -1.000000000000000000 ) ) ;
#113563=EDGE_CURVE ( 'NONE', #210574, #57819, #167351, .T. ) ;
#113568=VERTEX_POINT ( 'NONE', #116069 ) ;
#113581=EDGE_CURVE ( 'NONE', #177623, #184620, #196354, .T. ) ;
#113604=ADVANCED_FACE ( 'NONE', ( #204569 ), #179896, .T. ) ;
#113629=VERTEX_POINT ( 'NONE', #23405 ) ;
#113689=AXIS2_PLACEMENT_3D ( 'NONE', #200850, #40531, #120057 ) ;
#113710=AXIS2_PLACEMENT_3D ( 'NONE', #192845, #255313, #91162 ) ;
#113713=TOROIDAL_SURFACE ( 'NONE', #184434, 4.150000000000000355, 0.1000000000000000056 ) ;
#113843=AXIS2_PLACEMENT_3D ( 'NONE', #126310, #125047, #27258 ) ;
#113855=VERTEX_POINT ( 'NONE', #50617 ) ;
#113860=ORIENTED_EDGE ( 'NONE', *, *, #10581, .F. ) ;
#113870=ORIENTED_EDGE ( 'NONE', *, *, #94129, .T. ) ;
#113895=CIRCLE ( 'NONE', #84625, 11.75000000000000000 ) ;
#113920=CARTESIAN_POINT ( 'NONE',  ( -11.59999999999994458, 67.65000000001118963, -16.98168612828748536 ) ) ;
#113963=ORIENTED_EDGE ( 'NONE', *, *, #115090, .F. ) ;
#113971=CARTESIAN_POINT ( 'NONE',  ( -20.94999999999994600, 87.75000000001119815, -4.523107484524794053 ) ) ;
#114106=VERTEX_POINT ( 'NONE', #25630 ) ;
#114134=AXIS2_PLACEMENT_3D ( 'NONE', #254292, #213899, #35308 ) ;
#114164=VECTOR ( 'NONE', #142419, 1000.000000000000000 ) ;
#114172=EDGE_CURVE ( 'NONE', #146220, #249282, #40090, .T. ) ;
#114266=CARTESIAN_POINT ( 'NONE',  ( -21.14999999999994174, 64.35000000001120668, -5.923107484524795296 ) ) ;
#114287=LINE ( 'NONE', #249953, #97865 ) ;
#114288=VERTEX_POINT ( 'NONE', #184688 ) ;
#114372=ORIENTED_EDGE ( 'NONE', *, *, #162810, .F. ) ;
#114389=AXIS2_PLACEMENT_3D ( 'NONE', #81012, #200986, #83567 ) ;
#114442=VERTEX_POINT ( 'NONE', #252357 ) ;
#114460=ORIENTED_EDGE ( 'NONE', *, *, #186080, .T. ) ;
#114503=ADVANCED_FACE ( 'NONE', ( #20197 ), #192643, .T. ) ;
#114542=CARTESIAN_POINT ( 'NONE',  ( -20.94999999999994600, 65.35000000001120668, -4.523107484524794053 ) ) ;
#114549=DIRECTION ( 'NONE',  ( 0.000000000000000000, 0.000000000000000000, -1.000000000000000000 ) ) ;
#114575=VERTEX_POINT ( 'NONE', #155331 ) ;
#114607=CIRCLE ( 'NONE', #64528, 11.65000000000000036 ) ;
#114608=ORIENTED_EDGE ( 'NONE', *, *, #234616, .T. ) ;
#114634=FACE_OUTER_BOUND ( 'NONE', #210527, .T. ) ;
#114691=VECTOR ( 'NONE', #15572, 1000.000000000000000 ) ;
#114730=CARTESIAN_POINT ( 'NONE',  ( 0.9000000000000547562, 64.25000000001119815, -7.323107484524790323 ) ) ;
#114751=TOROIDAL_SURFACE ( 'NONE', #64665, 0.2000000000000000111, 0.1000000000000000056 ) ;
#114783=DIRECTION ( 'NONE',  ( -0.000000000000000000, -0.1575546449569685259, 0.9875102702516485031 ) ) ;
#114802=DIRECTION ( 'NONE',  ( 3.469446951953515108E-14, -1.000000000000000000, 0.000000000000000000 ) ) ;
#114894=CIRCLE ( 'NONE', #252236, 0.1000000000000021844 ) ;
#114958=EDGE_CURVE ( 'NONE', #514, #122992, #230231, .T. ) ;
#114964=FACE_OUTER_BOUND ( 'NONE', #216225, .T. ) ;
#115024=CARTESIAN_POINT ( 'NONE',  ( 23.50000000000005684, 76.00000000001119815, -40.17310748452479174 ) ) ;
#115044=ORIENTED_EDGE ( 'NONE', *, *, #246345, .F. ) ;
#115050=ORIENTED_EDGE ( 'NONE', *, *, #183615, .T. ) ;
#115063=DIRECTION ( 'NONE',  ( 1.000000000000000000, 0.000000000000000000, -0.000000000000000000 ) ) ;
#115074=VECTOR ( 'NONE', #230772, 1000.000000000000000 ) ;
#115083=AXIS2_PLACEMENT_3D ( 'NONE', #899, #24374, #84264 ) ;
#115090=EDGE_CURVE ( 'NONE', #68335, #29322, #238802, .T. ) ;
#115158=ORIENTED_EDGE ( 'NONE', *, *, #228458, .T. ) ;
#115178=EDGE_CURVE ( 'NONE', #26247, #179805, #6163, .T. ) ;
#115192=LINE ( 'NONE', #19958, #82495 ) ;
#115237=VECTOR ( 'NONE', #85150, 1000.000000000000000 ) ;
#115238=ORIENTED_EDGE ( 'NONE', *, *, #151885, .F. ) ;
#115248=DIRECTION ( 'NONE',  ( 1.000000000000000000, 0.000000000000000000, 0.000000000000000000 ) ) ;
#115303=CYLINDRICAL_SURFACE ( 'NONE', #66519, 0.09999999999999648059 ) ;
#115407=CARTESIAN_POINT ( 'NONE',  ( -21.04999999999994387, 67.82483145523551116, -25.59432346794077162 ) ) ;
#115445=CARTESIAN_POINT ( 'NONE',  ( 20.95000000000005258, 66.25000000001119815, -5.923107484524795296 ) ) ;
#115455=DIRECTION ( 'NONE',  ( -0.000000000000000000, -0.9910827722268049644, -0.1332476588733589318 ) ) ;
#115515=ORIENTED_EDGE ( 'NONE', *, *, #168710, .T. ) ;
#115521=DIRECTION ( 'NONE',  ( 0.000000000000000000, 0.000000000000000000, 1.000000000000000000 ) ) ;
#115538=EDGE_CURVE ( 'NONE', #59396, #6487, #71954, .T. ) ;
#115540=DIRECTION ( 'NONE',  ( 0.000000000000000000, -0.000000000000000000, -1.000000000000000000 ) ) ;
#115551=VERTEX_POINT ( 'NONE', #146329 ) ;
#115644=DIRECTION ( 'NONE',  ( 0.000000000000000000, -0.9910827722268050755, 0.1332476588733589318 ) ) ;
#115646=AXIS2_PLACEMENT_3D ( 'NONE', #202638, #163520, #243048 ) ;
#115679=CARTESIAN_POINT ( 'NONE',  ( 20.95000000000005258, 65.15000000001120384, -3.123107484524795474 ) ) ;
#115710=CIRCLE ( 'NONE', #3251, 3.970710678118653636 ) ;
#115725=ORIENTED_EDGE ( 'NONE', *, *, #35042, .T. ) ;
#115736=DIRECTION ( 'NONE',  ( 3.469446951953515108E-14, 1.000000000000000000, 0.000000000000000000 ) ) ;
#115780=DIRECTION ( 'NONE',  ( 0.000000000000000000, 0.9889818879709274535, 0.1480365673253065395 ) ) ;
#115785=DIRECTION ( 'NONE',  ( -1.000000000000000000, 0.000000000000000000, 0.000000000000000000 ) ) ;
#115846=AXIS2_PLACEMENT_3D ( 'NONE', #233734, #138441, #135880 ) ;
#115856=CARTESIAN_POINT ( 'NONE',  ( 21.15000000000005187, 87.60324567546805952, -34.17184040628037422 ) ) ;
#115876=DIRECTION ( 'NONE',  ( -2.141321560717106639E-14, 0.1575546449569727447, -0.9875102702516477260 ) ) ;
#115889=ADVANCED_FACE ( 'NONE', ( #10391 ), #46913, .F. ) ;
#115922=ORIENTED_EDGE ( 'NONE', *, *, #103283, .F. ) ;
#115961=DIRECTION ( 'NONE',  ( -2.141321560717181029E-15, 0.1575546449569727447, 0.9875102702516478370 ) ) ;
#115966=DIRECTION ( 'NONE',  ( -0.000000000000000000, -0.000000000000000000, 1.000000000000000000 ) ) ;
#115967=AXIS2_PLACEMENT_3D ( 'NONE', #67075, #209142, #108766 ) ;
#115979=FACE_OUTER_BOUND ( 'NONE', #250204, .T. ) ;
#116022=EDGE_CURVE ( 'NONE', #178868, #211462, #47041, .T. ) ;
#116023=CARTESIAN_POINT ( 'NONE',  ( 21.15000000000005542, 67.85000000001119247, -3.023107484524792277 ) ) ;
#116069=CARTESIAN_POINT ( 'NONE',  ( -23.49999999999994316, 82.64476912853859858, -26.37791261425322986 ) ) ;
#116091=EDGE_LOOP ( 'NONE', ( #3565, #217661, #234028, #173957 ) ) ;
#116182=CARTESIAN_POINT ( 'NONE',  ( 20.95000000000005258, 66.15000000001120384, -4.623107484524796362 ) ) ;
#116188=DIRECTION ( 'NONE',  ( 0.000000000000000000, 0.000000000000000000, 1.000000000000000000 ) ) ;
#116243=CARTESIAN_POINT ( 'NONE',  ( -21.04999999999994387, 74.94272479589878344, -3.123107484524795474 ) ) ;
#116245=DIRECTION ( 'NONE',  ( 0.000000000000000000, 0.000000000000000000, 1.000000000000000000 ) ) ;
#116279=VERTEX_POINT ( 'NONE', #25780 ) ;
#116343=VECTOR ( 'NONE', #130843, 1000.000000000000000 ) ;
#116375=AXIS2_PLACEMENT_3D ( 'NONE', #161846, #242629, #100522 ) ;
#116468=VECTOR ( 'NONE', #250091, 1000.000000000000000 ) ;
#116532=VECTOR ( 'NONE', #189446, 1000.000000000000000 ) ;
#116553=ORIENTED_EDGE ( 'NONE', *, *, #30190, .T. ) ;
#116586=ORIENTED_EDGE ( 'NONE', *, *, #61513, .T. ) ;
#116595=TOROIDAL_SURFACE ( 'NONE', #4165, 0.2000000000000000111, 0.1000000000000000056 ) ;
#116617=CARTESIAN_POINT ( 'NONE',  ( 23.40000000000005187, 76.00000000001119815, -40.07310748452479032 ) ) ;
#116712=CARTESIAN_POINT ( 'NONE',  ( 23.40000000000005187, 64.25000000001119815, -36.02310748452479316 ) ) ;
#116762=DIRECTION ( 'NONE',  ( -0.000000000000000000, -1.000000000000000000, 0.000000000000000000 ) ) ;
#116764=ORIENTED_EDGE ( 'NONE', *, *, #213005, .T. ) ;
#116772=DIRECTION ( 'NONE',  ( 0.000000000000000000, -1.000000000000000000, 0.000000000000000000 ) ) ;
#116777=VERTEX_POINT ( 'NONE', #189684 ) ;
#116879=FACE_OUTER_BOUND ( 'NONE', #101828, .T. ) ;
#116907=DIRECTION ( 'NONE',  ( 0.000000000000000000, 0.000000000000000000, -1.000000000000000000 ) ) ;
#116917=FACE_OUTER_BOUND ( 'NONE', #198954, .T. ) ;
#116945=EDGE_CURVE ( 'NONE', #12197, #129355, #76634, .T. ) ;
#116976=AXIS2_PLACEMENT_3D ( 'NONE', #15498, #238360, #216224 ) ;
#117002=CARTESIAN_POINT ( 'NONE',  ( -13.39999999999994351, 67.75000000001118394, -23.62310748452479103 ) ) ;
#117070=DIRECTION ( 'NONE',  ( 0.000000000000000000, 0.000000000000000000, -1.000000000000000000 ) ) ;
#117092=DIRECTION ( 'NONE',  ( -1.000000000000000000, 0.000000000000000000, 0.000000000000000000 ) ) ;
#117100=LINE ( 'NONE', #119672, #194383 ) ;
#117109=CYLINDRICAL_SURFACE ( 'NONE', #48419, 0.1000000000000028644 ) ;
#117135=DIRECTION ( 'NONE',  ( 1.000000000000000000, 0.000000000000000000, 0.000000000000000000 ) ) ;
#117140=VERTEX_POINT ( 'NONE', #87369 ) ;
#117148=CARTESIAN_POINT ( 'NONE',  ( 21.15000000000005187, 77.83551161375991967, -47.52760213295649550 ) ) ;
#117157=EDGE_LOOP ( 'NONE', ( #189956, #6577, #207391, #224857 ) ) ;
#117185=EDGE_LOOP ( 'NONE', ( #42109, #152279, #96537, #34000 ) ) ;
#117209=DIRECTION ( 'NONE',  ( 1.000000000000000000, -3.469446951953635646E-14, 0.000000000000000000 ) ) ;
#117218=ORIENTED_EDGE ( 'NONE', *, *, #235505, .F. ) ;
#117230=DIRECTION ( 'NONE',  ( -1.000000000000000000, -3.439547145395919517E-14, -4.624352451196577991E-15 ) ) ;
#117244=DIRECTION ( 'NONE',  ( 0.000000000000000000, 0.000000000000000000, -1.000000000000000000 ) ) ;
#117257=AXIS2_PLACEMENT_3D ( 'NONE', #38235, #61639, #141179 ) ;
#117266=AXIS2_PLACEMENT_3D ( 'NONE', #243702, #62506, #41671 ) ;
#117267=AXIS2_PLACEMENT_3D ( 'NONE', #11227, #187306, #68635 ) ;
#117272=CARTESIAN_POINT ( 'NONE',  ( 23.40000000000005542, 64.35000000001120668, -3.123107484524795474 ) ) ;
#117290=ORIENTED_EDGE ( 'NONE', *, *, #174597, .F. ) ;
#117299=AXIS2_PLACEMENT_3D ( 'NONE', #239372, #58135, #138943 ) ;
#117310=EDGE_CURVE ( 'NONE', #134771, #74886, #122640, .T. ) ;
#117319=EDGE_CURVE ( 'NONE', #98456, #88017, #173397, .T. ) ;
#117373=FACE_OUTER_BOUND ( 'NONE', #1303, .T. ) ;
#117374=CARTESIAN_POINT ( 'NONE',  ( 21.05000000000005400, 87.75000000001122658, -30.12310748452481235 ) ) ;
#117588=VECTOR ( 'NONE', #26045, 1000.000000000000000 ) ;
#117615=FACE_OUTER_BOUND ( 'NONE', #197759, .T. ) ;
#117628=CARTESIAN_POINT ( 'NONE',  ( -21.14999999999994174, 64.35000000001120668, -3.123107484524795474 ) ) ;
#117682=VERTEX_POINT ( 'NONE', #191346 ) ;
#117709=CARTESIAN_POINT ( 'NONE',  ( -23.49999999999994316, 76.00000000001119815, -31.97310748452479601 ) ) ;
#117786=DIRECTION ( 'NONE',  ( 0.000000000000000000, 0.000000000000000000, 1.000000000000000000 ) ) ;
#117834=EDGE_CURVE ( 'NONE', #35839, #9389, #237413, .T. ) ;
#117874=EDGE_CURVE ( 'NONE', #52328, #189336, #208394, .T. ) ;
#117888=ADVANCED_FACE ( 'NONE', ( #7211 ), #104996, .T. ) ;
#117973=DIRECTION ( 'NONE',  ( 0.000000000000000000, 0.000000000000000000, -1.000000000000000000 ) ) ;
#118016=DIRECTION ( 'NONE',  ( 0.000000000000000000, 0.000000000000000000, -1.000000000000000000 ) ) ;
#118055=VECTOR ( 'NONE', #224618, 1000.000000000000000 ) ;
#118095=DIRECTION ( 'NONE',  ( 0.000000000000000000, 0.000000000000000000, -1.000000000000000000 ) ) ;
#118136=ORIENTED_EDGE ( 'NONE', *, *, #218913, .F. ) ;
#118161=ADVANCED_FACE ( 'NONE', ( #86302 ), #47182, .T. ) ;
#118201=EDGE_LOOP ( 'NONE', ( #19480, #138196, #9586, #143983 ) ) ;
#118259=VERTEX_POINT ( 'NONE', #233356 ) ;
#118260=VECTOR ( 'NONE', #247924, 1000.000000000000114 ) ;
#118295=EDGE_CURVE ( 'NONE', #20544, #225270, #79367, .T. ) ;
#118305=CYLINDRICAL_SURFACE ( 'NONE', #225526, 0.1000000000000028644 ) ;
#118344=AXIS2_PLACEMENT_3D ( 'NONE', #196411, #38633, #137706 ) ;
#118363=VERTEX_POINT ( 'NONE', #59796 ) ;
#118373=CARTESIAN_POINT ( 'NONE',  ( -21.04999999999994387, 64.35000000001120668, -51.02310748452479316 ) ) ;
#118395=CARTESIAN_POINT ( 'NONE',  ( -21.04999999999994387, 83.97335046823651794, -34.66234602115918051 ) ) ;
#118396=DIRECTION ( 'NONE',  ( 0.000000000000000000, 0.000000000000000000, -1.000000000000000000 ) ) ;
#118397=CARTESIAN_POINT ( 'NONE',  ( -21.14999999999994174, 76.00000000001119815, -36.02310748452479316 ) ) ;
#118458=ORIENTED_EDGE ( 'NONE', *, *, #164619, .F. ) ;
#118465=AXIS2_PLACEMENT_3D ( 'NONE', #243504, #29630, #67434 ) ;
#118468=AXIS2_PLACEMENT_3D ( 'NONE', #28239, #167743, #247236 ) ;
#118499=AXIS2_PLACEMENT_3D ( 'NONE', #104901, #68392, #29300 ) ;
#118528=EDGE_LOOP ( 'NONE', ( #206903, #183107, #2592, #123087 ) ) ;
#118561=CARTESIAN_POINT ( 'NONE',  ( -23.49999999999994316, 74.14873292176677921, -47.62635315998165453 ) ) ;
#118623=ADVANCED_FACE ( 'NONE', ( #55300 ), #115303, .T. ) ;
#118707=DIRECTION ( 'NONE',  ( 1.000000000000000000, 0.000000000000000000, 0.000000000000000000 ) ) ;
#118761=DIRECTION ( 'NONE',  ( 0.000000000000000000, 0.000000000000000000, 1.000000000000000000 ) ) ;
#118811=AXIS2_PLACEMENT_3D ( 'NONE', #74785, #36941, #155605 ) ;
#118861=DIRECTION ( 'NONE',  ( 4.336808689942017736E-16, -0.000000000000000000, 1.000000000000000000 ) ) ;
#118882=CARTESIAN_POINT ( 'NONE',  ( -0.8999999999999437339, 67.75000000001118394, -12.62310748452478926 ) ) ;
#118898=EDGE_CURVE ( 'NONE', #80585, #192885, #134551, .T. ) ;
#118902=CARTESIAN_POINT ( 'NONE',  ( -20.94999999999994600, 64.25000000001119815, -6.123107484524794586 ) ) ;
#118910=VECTOR ( 'NONE', #62721, 1000.000000000000000 ) ;
#118912=EDGE_CURVE ( 'NONE', #139130, #183226, #96694, .T. ) ;
#118917=ORIENTED_EDGE ( 'NONE', *, *, #256458, .F. ) ;
#119107=CARTESIAN_POINT ( 'NONE',  ( -5.899999999999938183, 64.25000000001119815, -26.12310748452479103 ) ) ;
#119127=DIRECTION ( 'NONE',  ( 0.000000000000000000, 1.000000000000000000, 0.000000000000000000 ) ) ;
#119231=DIRECTION ( 'NONE',  ( -0.000000000000000000, -0.000000000000000000, 1.000000000000000000 ) ) ;
#119288=VERTEX_POINT ( 'NONE', #155158 ) ;
#119353=DIRECTION ( 'NONE',  ( 0.000000000000000000, -1.000000000000000000, 0.000000000000000000 ) ) ;
#119358=VERTEX_POINT ( 'NONE', #19470 ) ;
#119496=DIRECTION ( 'NONE',  ( 0.000000000000000000, 0.000000000000000000, -1.000000000000000000 ) ) ;
#119536=ORIENTED_EDGE ( 'NONE', *, *, #17368, .F. ) ;
#119578=FACE_OUTER_BOUND ( 'NONE', #79425, .T. ) ;
#119620=CARTESIAN_POINT ( 'NONE',  ( -23.39999999999994529, 82.84256550613280012, -26.34830530078816935 ) ) ;
#119670=CARTESIAN_POINT ( 'NONE',  ( -0.8999999999999438449, 67.75000000001118394, -14.06452884076210275 ) ) ;
#119672=CARTESIAN_POINT ( 'NONE',  ( -20.94999999999994600, 61.64150943397345372, -36.51839050339276582 ) ) ;
#119718=ADVANCED_FACE ( 'NONE', ( #255136 ), #150965, .T. ) ;
#119756=CIRCLE ( 'NONE', #61487, 0.1000000000000028644 ) ;
#119766=EDGE_CURVE ( 'NONE', #80961, #134698, #202919, .T. ) ;
#119785=CARTESIAN_POINT ( 'NONE',  ( -0.8999999999999437339, 67.72071067812984779, -10.02310748452479139 ) ) ;
#119789=ORIENTED_EDGE ( 'NONE', *, *, #184155, .F. ) ;
#119819=ORIENTED_EDGE ( 'NONE', *, *, #131741, .T. ) ;
#119822=FACE_BOUND ( 'NONE', #117157, .T. ) ;
#119834=ADVANCED_FACE ( 'NONE', ( #58262 ), #108924, .T. ) ;
#119836=CARTESIAN_POINT ( 'NONE',  ( -0.8999999999999435119, 66.35000000001119247, -12.62310748452479281 ) ) ;
#119867=EDGE_LOOP ( 'NONE', ( #146308, #71308, #166653, #1489 ) ) ;
#119893=DIRECTION ( 'NONE',  ( 1.000000000000000000, 0.000000000000000000, 0.000000000000000000 ) ) ;
#120045=ORIENTED_EDGE ( 'NONE', *, *, #142070, .F. ) ;
#120057=DIRECTION ( 'NONE',  ( 0.000000000000000000, 0.9910827722268055195, -0.1332476588733540468 ) ) ;
#120140=DIRECTION ( 'NONE',  ( -0.000000000000000000, -1.000000000000000000, 0.000000000000000000 ) ) ;
#120188=EDGE_LOOP ( 'NONE', ( #223704, #112026, #200357, #76396 ) ) ;
#120200=FACE_OUTER_BOUND ( 'NONE', #30358, .T. ) ;
#120227=AXIS2_PLACEMENT_3D ( 'NONE', #129133, #252918, #130403 ) ;
#120231=DIRECTION ( 'NONE',  ( 0.000000000000000000, 0.000000000000000000, 1.000000000000000000 ) ) ;
#120246=EDGE_LOOP ( 'NONE', ( #9798, #30372, #92857, #32575 ) ) ;
#120339=CIRCLE ( 'NONE', #178589, 3.970710678118657189 ) ;
#120350=CARTESIAN_POINT ( 'NONE',  ( -13.39999999999994529, 66.35000000001119247, -21.02310748452479316 ) ) ;
#120352=AXIS2_PLACEMENT_3D ( 'NONE', #133681, #72447, #32046 ) ;
#120386=AXIS2_PLACEMENT_3D ( 'NONE', #140113, #196251, #81411 ) ;
#120492=EDGE_LOOP ( 'NONE', ( #120781, #56210, #202897, #62657 ) ) ;
#120510=EDGE_LOOP ( 'NONE', ( #204931, #158724, #149244, #132003 ) ) ;
#120573=EDGE_CURVE ( 'NONE', #60123, #231379, #59013, .T. ) ;
#120582=FACE_OUTER_BOUND ( 'NONE', #66218, .T. ) ;
#120585=ORIENTED_EDGE ( 'NONE', *, *, #90867, .F. ) ;
#120636=ADVANCED_FACE ( 'NONE', ( #46751 ), #230547, .T. ) ;
#120678=CARTESIAN_POINT ( 'NONE',  ( 21.05000000000005400, 64.35000000001120668, -5.923107484524795296 ) ) ;
#120715=ORIENTED_EDGE ( 'NONE', *, *, #223332, .T. ) ;
#120736=DIRECTION ( 'NONE',  ( 1.000000000000000000, -0.000000000000000000, -0.000000000000000000 ) ) ;
#120746=CIRCLE ( 'NONE', #149787, 0.09999999999999939493 ) ;
#120758=DIRECTION ( 'NONE',  ( 0.000000000000000000, 1.000000000000000000, 0.000000000000000000 ) ) ;
#120774=DIRECTION ( 'NONE',  ( 0.000000000000000000, 0.000000000000000000, 1.000000000000000000 ) ) ;
#120775=ORIENTED_EDGE ( 'NONE', *, *, #250769, .T. ) ;
#120781=ORIENTED_EDGE ( 'NONE', *, *, #71196, .T. ) ;
#120841=DIRECTION ( 'NONE',  ( 1.284012543211123464E-15, 0.1480365673253023762, -0.9889818879709281196 ) ) ;
#120858=ADVANCED_FACE ( 'NONE', ( #877 ), #109291, .T. ) ;
#120930=DIRECTION ( 'NONE',  ( 0.000000000000000000, 0.000000000000000000, 1.000000000000000000 ) ) ;
#120937=CIRCLE ( 'NONE', #16873, 0.1000000000000028644 ) ;
#120961=EDGE_CURVE ( 'NONE', #56891, #251948, #167590, .T. ) ;
#120971=ORIENTED_EDGE ( 'NONE', *, *, #137954, .F. ) ;
#121095=AXIS2_PLACEMENT_3D ( 'NONE', #117148, #95004, #173319 ) ;
#121144=VERTEX_POINT ( 'NONE', #115407 ) ;
#121209=AXIS2_PLACEMENT_3D ( 'NONE', #193141, #97846, #15809 ) ;
#121247=EDGE_CURVE ( 'NONE', #253379, #249805, #234380, .T. ) ;
#121280=CIRCLE ( 'NONE', #17202, 0.09999999999999982514 ) ;
#121327=ORIENTED_EDGE ( 'NONE', *, *, #41876, .T. ) ;
#121358=ADVANCED_FACE ( 'NONE', ( #129553 ), #186977, .T. ) ;
#121376=AXIS2_PLACEMENT_3D ( 'NONE', #239648, #139227, #140524 ) ;
#121439=EDGE_LOOP ( 'NONE', ( #233278, #178938, #220434, #141693 ) ) ;
#121440=CARTESIAN_POINT ( 'NONE',  ( -21.04999999999994387, 77.16254490893143725, -44.02310748452479316 ) ) ;
#121478=CYLINDRICAL_SURFACE ( 'NONE', #114389, 0.1000000000000028644 ) ;
#121523=VERTEX_POINT ( 'NONE', #14764 ) ;
#121640=EDGE_LOOP ( 'NONE', ( #135753, #20423, #77738, #154415 ) ) ;
#121729=CARTESIAN_POINT ( 'NONE',  ( -5.899999999999938183, 64.25000000001119815, -21.92310748452479174 ) ) ;
#121734=ADVANCED_FACE ( 'NONE', ( #179323 ), #222248, .T. ) ;
#121842=CARTESIAN_POINT ( 'NONE',  ( -13.39999999999994529, 67.75000000001118394, -21.02310748452479316 ) ) ;
#121881=ORIENTED_EDGE ( 'NONE', *, *, #118912, .F. ) ;
#121955=DIRECTION ( 'NONE',  ( 0.000000000000000000, 0.000000000000000000, 1.000000000000000000 ) ) ;
#121967=CARTESIAN_POINT ( 'NONE',  ( 23.40000000000005542, 74.83745509109094485, -43.92310748452479885 ) ) ;
#121989=EDGE_LOOP ( 'NONE', ( #56513, #128044, #20297, #88361 ) ) ;
#122097=CARTESIAN_POINT ( 'NONE',  ( -40.23850191057533010, 66.15000000001120384, -4.623107484524796362 ) ) ;
#122109=CARTESIAN_POINT ( 'NONE',  ( 13.40000000000005898, 67.75000000001118394, -25.06452884076209742 ) ) ;
#122157=ORIENTED_EDGE ( 'NONE', *, *, #150092, .T. ) ;
#122187=DIRECTION ( 'NONE',  ( 0.000000000000000000, -1.000000000000000000, 0.000000000000000000 ) ) ;
#122203=ORIENTED_EDGE ( 'NONE', *, *, #134649, .T. ) ;
#122204=LINE ( 'NONE', #4787, #22429 ) ;
#122228=AXIS2_PLACEMENT_3D ( 'NONE', #174656, #37681, #153809 ) ;
#122281=DIRECTION ( 'NONE',  ( 1.000000000000000000, 0.000000000000000000, 0.000000000000000000 ) ) ;
#122290=CARTESIAN_POINT ( 'NONE',  ( 21.15000000000005542, 74.94272479589878344, -3.123107484524795474 ) ) ;
#122294=CARTESIAN_POINT ( 'NONE',  ( 13.40000000000005898, 67.75000000001118394, -25.06452884076209742 ) ) ;
#122302=EDGE_CURVE ( 'NONE', #63115, #40557, #226526, .T. ) ;
#122319=DIRECTION ( 'NONE',  ( 0.000000000000000000, -1.000000000000000000, 0.000000000000000000 ) ) ;
#122405=LINE ( 'NONE', #237220, #103153 ) ;
#122419=VERTEX_POINT ( 'NONE', #195713 ) ;
#122427=VECTOR ( 'NONE', #174626, 1000.000000000000000 ) ;
#122430=ORIENTED_EDGE ( 'NONE', *, *, #226784, .T. ) ;
#122436=CIRCLE ( 'NONE', #43141, 0.09999999999999939493 ) ;
#122461=LINE ( 'NONE', #3786, #222972 ) ;
#122474=FACE_OUTER_BOUND ( 'NONE', #72791, .T. ) ;
#122515=AXIS2_PLACEMENT_3D ( 'NONE', #60163, #223093, #238819 ) ;
#122531=VECTOR ( 'NONE', #232304, 1000.000000000000114 ) ;
#122553=CARTESIAN_POINT ( 'NONE',  ( -21.14999999999994174, 83.80000000001119531, -34.86056257560453986 ) ) ;
#122554=EDGE_LOOP ( 'NONE', ( #227314, #38019, #196420, #97690 ) ) ;
#122571=EDGE_CURVE ( 'NONE', #45940, #130445, #84678, .T. ) ;
#122578=ORIENTED_EDGE ( 'NONE', *, *, #245727, .T. ) ;
#122592=CARTESIAN_POINT ( 'NONE',  ( -11.59999999999994458, 67.75000000001118394, -18.42310748452479174 ) ) ;
#122640=CIRCLE ( 'NONE', #39446, 0.1000000000000021844 ) ;
#122679=ADVANCED_FACE ( 'NONE', ( #91137 ), #149851, .T. ) ;
#122682=CIRCLE ( 'NONE', #76861, 0.1000000000000002554 ) ;
#122688=LINE ( 'NONE', #23604, #188496 ) ;
#122705=ORIENTED_EDGE ( 'NONE', *, *, #217003, .T. ) ;
#122715=CARTESIAN_POINT ( 'NONE',  ( 5.900000000000060751, 64.65000000001120384, -22.02310748452479316 ) ) ;
#122786=AXIS2_PLACEMENT_3D ( 'NONE', #211896, #33283, #128492 ) ;
#122805=VECTOR ( 'NONE', #207814, 1000.000000000000114 ) ;
#122839=CARTESIAN_POINT ( 'NONE',  ( 21.15000000000005187, 77.25000000001119815, -43.92310748452479885 ) ) ;
#122851=CARTESIAN_POINT ( 'NONE',  ( -21.14999999999994174, 76.00000000001119815, -36.02310748452479316 ) ) ;
#122864=DIRECTION ( 'NONE',  ( 1.000000000000000000, -0.000000000000000000, -0.000000000000000000 ) ) ;
#122884=COLOUR_RGB ( '', 0.08235294, 0.09019608, 0.10196078) ;
#122892=DIRECTION ( 'NONE',  ( 1.000000000000000000, -0.000000000000000000, -0.000000000000000000 ) ) ;
#122893=CARTESIAN_POINT ( 'NONE',  ( 21.05000000000003979, 83.90000000001120384, -37.18565239344504647 ) ) ;
#122898=VECTOR ( 'NONE', #166955, 1000.000000000000000 ) ;
#122932=CARTESIAN_POINT ( 'NONE',  ( -21.14999999999994174, 77.83551161375991967, -47.52760213295649550 ) ) ;
#122992=VERTEX_POINT ( 'NONE', #104892 ) ;
#122996=CIRCLE ( 'NONE', #206191, 0.1999999999999987899 ) ;
#123009=CARTESIAN_POINT ( 'NONE',  ( 23.40000000000005542, 77.83551161375991967, -47.52760213295649550 ) ) ;
#123048=CIRCLE ( 'NONE', #152296, 0.1000000000000028644 ) ;
#123069=AXIS2_PLACEMENT_3D ( 'NONE', #197968, #41493, #40218 ) ;
#123076=CIRCLE ( 'NONE', #6726, 0.09999999999999939493 ) ;
#123087=ORIENTED_EDGE ( 'NONE', *, *, #250244, .T. ) ;
#123118=CYLINDRICAL_SURFACE ( 'NONE', #115646, 11.74999999999999645 ) ;
#123157=FACE_OUTER_BOUND ( 'NONE', #19504, .T. ) ;
#123228=CYLINDRICAL_SURFACE ( 'NONE', #143059, 0.09999999999999530098 ) ;
#123255=DIRECTION ( 'NONE',  ( 0.000000000000000000, 0.000000000000000000, 1.000000000000000000 ) ) ;
#123305=PLANE ( 'NONE',  #15198 ) ;
#123306=CARTESIAN_POINT ( 'NONE',  ( -21.14999999999994174, 64.35000000001120668, -51.02310748452479316 ) ) ;
#123329=ORIENTED_EDGE ( 'NONE', *, *, #97713, .T. ) ;
#123360=VERTEX_POINT ( 'NONE', #9371 ) ;
#123429=PLANE ( 'NONE',  #198235 ) ;
#123439=CARTESIAN_POINT ( 'NONE',  ( 21.15000000000005187, 76.00000000001119815, -40.17310748452479174 ) ) ;
#123451=CARTESIAN_POINT ( 'NONE',  ( 0.9000000000000547562, 67.75000000001118394, -10.02310748452479139 ) ) ;
#123452=AXIS2_PLACEMENT_3D ( 'NONE', #158597, #120758, #239398 ) ;
#123459=DIRECTION ( 'NONE',  ( 1.000000000000000000, 0.000000000000000000, 0.000000000000000000 ) ) ;
#123626=DIRECTION ( 'NONE',  ( 0.000000000000000000, 0.000000000000000000, -1.000000000000000000 ) ) ;
#123655=CARTESIAN_POINT ( 'NONE',  ( -0.8999999999999437339, 64.25000000001119815, -10.02310748452479139 ) ) ;
#123693=CARTESIAN_POINT ( 'NONE',  ( -23.39999999999994529, 74.83745509109094485, -44.02310748452479316 ) ) ;
#123745=DIRECTION ( 'NONE',  ( 0.000000000000000000, 1.000000000000000000, -0.000000000000000000 ) ) ;
#123787=AXIS2_PLACEMENT_3D ( 'NONE', #127508, #115644, #256367 ) ;
#123791=CARTESIAN_POINT ( 'NONE',  ( -13.39999999999994351, 63.75000000001119815, -21.02310748452479316 ) ) ;
#123805=ADVANCED_FACE ( 'NONE', ( #89883 ), #48198, .F. ) ;
#123853=VERTEX_POINT ( 'NONE', #230707 ) ;
#123877=SURFACE_STYLE_FILL_AREA ( #83419 ) ;
#124070=CARTESIAN_POINT ( 'NONE',  ( -23.49999999999994316, 77.75000000001119815, -47.64205752314703801 ) ) ;
#124132=CARTESIAN_POINT ( 'NONE',  ( 21.05000000000005400, 66.15000000001120384, -6.023107484524798494 ) ) ;
#124133=FACE_OUTER_BOUND ( 'NONE', #232944, .T. ) ;
#124215=ORIENTED_EDGE ( 'NONE', *, *, #21985, .T. ) ;
#124247=CARTESIAN_POINT ( 'NONE',  ( 21.05000000000005400, 76.00000000001119815, -36.02310748452479316 ) ) ;
#124249=ORIENTED_EDGE ( 'NONE', *, *, #234340, .T. ) ;
#124282=ORIENTED_EDGE ( 'NONE', *, *, #81722, .F. ) ;
#124322=DIRECTION ( 'NONE',  ( 0.000000000000000000, 1.000000000000000000, 0.000000000000000000 ) ) ;
#124325=LINE ( 'NONE', #225949, #115237 ) ;
#124345=ORIENTED_EDGE ( 'NONE', *, *, #77961, .F. ) ;
#124355=CARTESIAN_POINT ( 'NONE',  ( 5.900000000000060751, 64.35000000001120668, -22.12310748452479103 ) ) ;
#124404=DIRECTION ( 'NONE',  ( -0.000000000000000000, 1.000000000000000000, -0.000000000000000000 ) ) ;
#124472=VECTOR ( 'NONE', #183057, 1000.000000000000114 ) ;
#124487=DIRECTION ( 'NONE',  ( 1.000000000000000000, -0.000000000000000000, -0.000000000000000000 ) ) ;
#124509=EDGE_CURVE ( 'NONE', #255132, #150150, #123048, .T. ) ;
#124639=DIRECTION ( 'NONE',  ( -1.000000000000000000, -0.000000000000000000, -0.000000000000000000 ) ) ;
#124674=PLANE ( 'NONE',  #213263 ) ;
#124697=DIRECTION ( 'NONE',  ( -1.000000000000000000, 0.000000000000000000, 0.000000000000000000 ) ) ;
#124727=CIRCLE ( 'NONE', #70589, 0.1000000000000032391 ) ;
#124748=DIRECTION ( 'NONE',  ( 0.000000000000000000, 1.000000000000000000, 0.000000000000000000 ) ) ;
#124844=DIRECTION ( 'NONE',  ( 0.000000000000000000, 0.000000000000000000, -1.000000000000000000 ) ) ;
#124913=CARTESIAN_POINT ( 'NONE',  ( -21.14999999999994174, 87.50449464844290048, -34.18759587077607165 ) ) ;
#124920=ORIENTED_EDGE ( 'NONE', *, *, #89228, .T. ) ;
#124961=DIRECTION ( 'NONE',  ( 0.000000000000000000, 0.000000000000000000, 1.000000000000000000 ) ) ;
#124962=CIRCLE ( 'NONE', #108207, 0.1999999999999987899 ) ;
#125016=AXIS2_PLACEMENT_3D ( 'NONE', #76020, #17344, #214257 ) ;
#125047=DIRECTION ( 'NONE',  ( -1.000000000000000000, 0.000000000000000000, 0.000000000000000000 ) ) ;
#125058=EDGE_LOOP ( 'NONE', ( #257231, #64217, #148639, #43914 ) ) ;
#125084=VECTOR ( 'NONE', #61829, 1000.000000000000000 ) ;
#125171=DIRECTION ( 'NONE',  ( 1.000000000000000000, 0.000000000000000000, 0.000000000000000000 ) ) ;
#125175=AXIS2_PLACEMENT_3D ( 'NONE', #134421, #18351, #116188 ) ;
#125203=ADVANCED_FACE ( 'NONE', ( #69947 ), #188579, .T. ) ;
#125219=ORIENTED_EDGE ( 'NONE', *, *, #62349, .T. ) ;
#125230=ORIENTED_EDGE ( 'NONE', *, *, #54126, .T. ) ;
#125306=FACE_OUTER_BOUND ( 'NONE', #71966, .T. ) ;
#125369=VECTOR ( 'NONE', #101954, 1000.000000000000000 ) ;
#125404=FACE_OUTER_BOUND ( 'NONE', #179500, .T. ) ;
#125405=EDGE_CURVE ( 'NONE', #209133, #135761, #187920, .T. ) ;
#125499=ORIENTED_EDGE ( 'NONE', *, *, #117319, .F. ) ;
#125537=DIRECTION ( 'NONE',  ( -0.000000000000000000, 1.000000000000000000, 0.000000000000000000 ) ) ;
#125578=EDGE_CURVE ( 'NONE', #148744, #39283, #174813, .T. ) ;
#125646=ADVANCED_FACE ( 'NONE', ( #176077 ), #177612, .T. ) ;
#125665=CARTESIAN_POINT ( 'NONE',  ( -5.999999999999938716, 64.75000000001119815, -26.02310748452479316 ) ) ;
#125689=ORIENTED_EDGE ( 'NONE', *, *, #52095, .T. ) ;
#125700=EDGE_LOOP ( 'NONE', ( #211438, #228678, #25552, #34360 ) ) ;
#125748=FACE_OUTER_BOUND ( 'NONE', #137645, .T. ) ;
#125765=AXIS2_PLACEMENT_3D ( 'NONE', #126305, #106733, #186302 ) ;
#125766=DIRECTION ( 'NONE',  ( 1.000000000000000000, 0.000000000000000000, 0.000000000000000000 ) ) ;
#125802=CIRCLE ( 'NONE', #71670, 0.1000000000000032391 ) ;
#125920=CARTESIAN_POINT ( 'NONE',  ( 11.60000000000006004, 67.75000000001118394, -16.98168612828748891 ) ) ;
#125990=CIRCLE ( 'NONE', #67745, 11.65000000000000036 ) ;
#125993=ORIENTED_EDGE ( 'NONE', *, *, #163016, .F. ) ;
#126012=ADVANCED_FACE ( 'NONE', ( #20203 ), #63153, .F. ) ;
#126025=ORIENTED_EDGE ( 'NONE', *, *, #174167, .F. ) ;
#126045=UNCERTAINTY_MEASURE_WITH_UNIT (LENGTH_MEASURE( 1.000000000000000082E-05 ), #164287, 'distance_accuracy_value', 'NONE');
#126051=AXIS2_PLACEMENT_3D ( 'NONE', #86980, #206962, #92143 ) ;
#126085=ORIENTED_EDGE ( 'NONE', *, *, #114172, .T. ) ;
#126109=CARTESIAN_POINT ( 'NONE',  ( -6.099999999999939249, 64.25000000001119815, -25.92310748452479174 ) ) ;
#126120=ORIENTED_EDGE ( 'NONE', *, *, #199533, .T. ) ;
#126225=LINE ( 'NONE', #165369, #50293 ) ;
#126282=EDGE_CURVE ( 'NONE', #103754, #187553, #65498, .T. ) ;
#126305=CARTESIAN_POINT ( 'NONE',  ( 11.60000000000006004, 64.35000000001120668, -23.72310748452479601 ) ) ;
#126309=EDGE_LOOP ( 'NONE', ( #163816, #125993, #20764, #100220 ) ) ;
#126310=CARTESIAN_POINT ( 'NONE',  ( 5.551115123125782702E-14, 67.65000000001118963, -3.123107484524795474 ) ) ;
#126339=CARTESIAN_POINT ( 'NONE',  ( -23.39999999999994529, 76.00000000001119815, -3.023107484524792277 ) ) ;
#126359=EDGE_LOOP ( 'NONE', ( #226542, #53455, #233100, #9290 ) ) ;
#126415=EDGE_CURVE ( 'NONE', #60636, #113073, #247912, .T. ) ;
#126449=EDGE_LOOP ( 'NONE', ( #227189, #249340, #225928, #210869 ) ) ;
#126478=CIRCLE ( 'NONE', #55519, 0.09999999999999530098 ) ;
#126501=EDGE_CURVE ( 'NONE', #176509, #148744, #15765, .T. ) ;
#126620=CARTESIAN_POINT ( 'NONE',  ( 20.95000000000005969, 65.36599112033563586, -30.02023607076051803 ) ) ;
#126625=FACE_OUTER_BOUND ( 'NONE', #200899, .T. ) ;
#126657=CARTESIAN_POINT ( 'NONE',  ( 21.15000000000005542, 83.80000000001119531, -34.86056257560453986 ) ) ;
#126736=VERTEX_POINT ( 'NONE', #142085 ) ;
#126744=DIRECTION ( 'NONE',  ( 4.336808689942017736E-16, 0.000000000000000000, 1.000000000000000000 ) ) ;
#126755=CYLINDRICAL_SURFACE ( 'NONE', #172638, 0.1000000000000028644 ) ;
#126764=DIRECTION ( 'NONE',  ( 0.000000000000000000, 0.000000000000000000, -1.000000000000000000 ) ) ;
#126799=DIRECTION ( 'NONE',  ( -1.000000000000000000, 0.000000000000000000, 0.000000000000000000 ) ) ;
#126801=EDGE_LOOP ( 'NONE', ( #48210, #171409, #95979, #44384 ) ) ;
#126840=ORIENTED_EDGE ( 'NONE', *, *, #138199, .T. ) ;
#126952=CARTESIAN_POINT ( 'NONE',  ( -23.49999999999994316, 87.51781941433023349, -37.75951082105083145 ) ) ;
#126955=CIRCLE ( 'NONE', #51918, 0.1000000000000028644 ) ;
#126959=AXIS2_PLACEMENT_3D ( 'NONE', #72502, #152047, #229003 ) ;
#126983=DIRECTION ( 'NONE',  ( 0.000000000000000000, 0.000000000000000000, -1.000000000000000000 ) ) ;
#127014=AXIS2_PLACEMENT_3D ( 'NONE', #51657, #187361, #145634 ) ;
#127041=DIRECTION ( 'NONE',  ( 1.000000000000000000, -0.000000000000000000, -0.000000000000000000 ) ) ;
#127061=ORIENTED_EDGE ( 'NONE', *, *, #45799, .F. ) ;
#127099=FACE_OUTER_BOUND ( 'NONE', #70297, .T. ) ;
#127104=ORIENTED_EDGE ( 'NONE', *, *, #79933, .T. ) ;
#127117=FACE_OUTER_BOUND ( 'NONE', #181819, .T. ) ;
#127118=DIRECTION ( 'NONE',  ( 1.000000000000000000, -0.000000000000000000, 0.000000000000000000 ) ) ;
#127203=LINE ( 'NONE', #205434, #225934 ) ;
#127220=ORIENTED_EDGE ( 'NONE', *, *, #84259, .T. ) ;
#127255=PLANE ( 'NONE',  #109357 ) ;
#127292=CARTESIAN_POINT ( 'NONE',  ( 21.05000000000005400, 66.15000000001120384, -4.623107484524796362 ) ) ;
#127295=EDGE_CURVE ( 'NONE', #56611, #249805, #199831, .T. ) ;
#127336=CARTESIAN_POINT ( 'NONE',  ( 5.900000000000059863, 64.65000000001120384, -26.02310748452479316 ) ) ;
#127348=DIRECTION ( 'NONE',  ( 0.000000000000000000, 0.1332476588733589318, -0.9910827722268050755 ) ) ;
#127439=ADVANCED_FACE ( 'NONE', ( #195051 ), #116595, .T. ) ;
#127446=ORIENTED_EDGE ( 'NONE', *, *, #68912, .T. ) ;
#127459=CARTESIAN_POINT ( 'NONE',  ( -13.39999999999994529, 67.75000000001118394, -25.06452884076210452 ) ) ;
#127463=DIRECTION ( 'NONE',  ( 0.000000000000000000, 0.000000000000000000, 1.000000000000000000 ) ) ;
#127495=DIRECTION ( 'NONE',  ( 0.000000000000000000, 0.000000000000000000, -1.000000000000000000 ) ) ;
#127508=CARTESIAN_POINT ( 'NONE',  ( -23.39999999999994529, 83.88667523412387084, -37.37221576174746929 ) ) ;
#127535=FACE_OUTER_BOUND ( 'NONE', #185659, .T. ) ;
#127537=DIRECTION ( 'NONE',  ( -0.000000000000000000, 1.000000000000000000, -0.000000000000000000 ) ) ;
#127561=ORIENTED_EDGE ( 'NONE', *, *, #151917, .F. ) ;
#127566=CIRCLE ( 'NONE', #256484, 4.150000000000001243 ) ;
#127577=DIRECTION ( 'NONE',  ( -3.756152431956878006E-15, -0.9910827722268042983, 0.1332476588733650935 ) ) ;
#127595=SPHERICAL_SURFACE ( 'NONE', #142165, 0.1000000000000000056 ) ;
#127605=EDGE_CURVE ( 'NONE', #225270, #110468, #236348, .T. ) ;
#127692=AXIS2_PLACEMENT_3D ( 'NONE', #257385, #218295, #201324 ) ;
#127725=PRESENTATION_STYLE_ASSIGNMENT (( #45615 ) ) ;
#127763=ORIENTED_EDGE ( 'NONE', *, *, #255989, .T. ) ;
#127773=ORIENTED_EDGE ( 'NONE', *, *, #157477, .F. ) ;
#127800=FACE_OUTER_BOUND ( 'NONE', #164757, .T. ) ;
#127838=DIRECTION ( 'NONE',  ( 0.000000000000000000, -0.1332476588733448597, 0.9910827722268067408 ) ) ;
#127877=DIRECTION ( 'NONE',  ( 0.000000000000000000, -0.000000000000000000, -1.000000000000000000 ) ) ;
#127920=DIRECTION ( 'NONE',  ( -1.000000000000000000, 0.000000000000000000, 0.000000000000000000 ) ) ;
#127970=ADVANCED_FACE ( 'NONE', ( #132860 ), #230672, .F. ) ;
#128044=ORIENTED_EDGE ( 'NONE', *, *, #251225, .F. ) ;
#128053=EDGE_LOOP ( 'NONE', ( #26124, #57017, #133893 ) ) ;
#128110=CARTESIAN_POINT ( 'NONE',  ( -23.39999999999994529, 76.00000000001119815, -36.02310748452479316 ) ) ;
#128119=VECTOR ( 'NONE', #88378, 1000.000000000000000 ) ;
#128131=VERTEX_POINT ( 'NONE', #42721 ) ;
#128152=VERTEX_POINT ( 'NONE', #180960 ) ;
#128194=CARTESIAN_POINT ( 'NONE',  ( -23.39999999999994529, 74.63923853664559260, -43.99645795275012006 ) ) ;
#128206=DIRECTION ( 'NONE',  ( 0.000000000000000000, 0.000000000000000000, 1.000000000000000000 ) ) ;
#128209=CARTESIAN_POINT ( 'NONE',  ( -21.14999999999994174, 76.00000000001119815, -36.02310748452479316 ) ) ;
#128347=DIRECTION ( 'NONE',  ( 0.000000000000000000, 0.000000000000000000, 1.000000000000000000 ) ) ;
#128351=CARTESIAN_POINT ( 'NONE',  ( -11.59999999999994458, 66.35000000001119247, -23.62310748452479103 ) ) ;
#128367=ORIENTED_EDGE ( 'NONE', *, *, #29198, .F. ) ;
#128376=ORIENTED_EDGE ( 'NONE', *, *, #61072, .T. ) ;
#128383=CARTESIAN_POINT ( 'NONE',  ( 23.50000000000005684, 83.97335046823651794, -34.66234602115918051 ) ) ;
#128408=DIRECTION ( 'NONE',  ( 1.000000000000000000, -0.000000000000000000, 0.000000000000000000 ) ) ;
#128431=ORIENTED_EDGE ( 'NONE', *, *, #116022, .T. ) ;
#128467=ORIENTED_EDGE ( 'NONE', *, *, #42522, .F. ) ;
#128482=CIRCLE ( 'NONE', #170231, 0.1999999999999987899 ) ;
#128490=DIRECTION ( 'NONE',  ( 1.000000000000000000, -0.000000000000000000, -0.000000000000000000 ) ) ;
#128492=DIRECTION ( 'NONE',  ( 0.000000000000000000, 0.1332476588733589318, 0.9910827722268049644 ) ) ;
#128540=EDGE_CURVE ( 'NONE', #139130, #234836, #257489, .T. ) ;
#128554=ADVANCED_FACE ( 'NONE', ( #223469 ), #66976, .T. ) ;
#128574=EDGE_LOOP ( 'NONE', ( #201223, #97507, #156649, #225793 ) ) ;
#128606=DIRECTION ( 'NONE',  ( 0.000000000000000000, -0.1332476588733645106, -0.9910827722268042983 ) ) ;
#128630=ORIENTED_EDGE ( 'NONE', *, *, #76753, .T. ) ;
#128637=EDGE_LOOP ( 'NONE', ( #174883, #197321, #187163, #64694 ) ) ;
#128674=ORIENTED_EDGE ( 'NONE', *, *, #67987, .T. ) ;
#128753=CARTESIAN_POINT ( 'NONE',  ( -23.39999999999994529, 83.97335046823651794, -34.66234602115918051 ) ) ;
#128775=ORIENTED_EDGE ( 'NONE', *, *, #169667, .F. ) ;
#128814=CYLINDRICAL_SURFACE ( 'NONE', #31619, 0.09999999999999939493 ) ;
#128854=ORIENTED_EDGE ( 'NONE', *, *, #59147, .F. ) ;
#128911=CARTESIAN_POINT ( 'NONE',  ( 23.40000000000005187, 79.88763423575340994, -7.282924647898262549 ) ) ;
#128932=AXIS2_PLACEMENT_3D ( 'NONE', #183728, #24675, #61204 ) ;
#128968=VECTOR ( 'NONE', #101305, 1000.000000000000000 ) ;
#128991=VECTOR ( 'NONE', #108946, 1000.000000000000000 ) ;
#129007=ORIENTED_EDGE ( 'NONE', *, *, #114172, .F. ) ;
#129008=FACE_OUTER_BOUND ( 'NONE', #247980, .T. ) ;
#129030=DIRECTION ( 'NONE',  ( 0.000000000000000000, 0.000000000000000000, -1.000000000000000000 ) ) ;
#129044=EDGE_LOOP ( 'NONE', ( #9898, #91215, #134661, #97466 ) ) ;
#129076=ORIENTED_EDGE ( 'NONE', *, *, #229977, .F. ) ;
#129131=EDGE_CURVE ( 'NONE', #53024, #96904, #141217, .T. ) ;
#129133=CARTESIAN_POINT ( 'NONE',  ( 21.15000000000004476, 84.00000000001119815, -34.86056257560453986 ) ) ;
#129219=TOROIDAL_SURFACE ( 'NONE', #133490, 11.65000000000000036, 0.1000000000000000056 ) ;
#129295=DIRECTION ( 'NONE',  ( 1.000000000000000000, -3.427148797533456523E-14, 5.467925025959484217E-15 ) ) ;
#129310=DIRECTION ( 'NONE',  ( 0.000000000000000000, 0.000000000000000000, 1.000000000000000000 ) ) ;
#129355=VERTEX_POINT ( 'NONE', #106582 ) ;
#129436=( NAMED_UNIT ( * ) PLANE_ANGLE_UNIT ( ) SI_UNIT ( $, .RADIAN. ) );
#129459=CIRCLE ( 'NONE', #233709, 11.75000000000000000 ) ;
#129462=AXIS2_PLACEMENT_3D ( 'NONE', #237244, #19487, #139400 ) ;
#129475=AXIS2_PLACEMENT_3D ( 'NONE', #57680, #178971, #38153 ) ;
#129484=EDGE_LOOP ( 'NONE', ( #183958, #135489, #256769, #204927 ) ) ;
#129524=FACE_OUTER_BOUND ( 'NONE', #254763, .T. ) ;
#129534=AXIS2_PLACEMENT_3D ( 'NONE', #30206, #189276, #164576 ) ;
#129553=FACE_OUTER_BOUND ( 'NONE', #121640, .T. ) ;
#129559=CIRCLE ( 'NONE', #121209, 0.1000000000000002554 ) ;
#129560=VECTOR ( 'NONE', #124697, 1000.000000000000000 ) ;
#129564=CARTESIAN_POINT ( 'NONE',  ( -20.94999999999994600, 66.15000000001120384, -5.923107484524795296 ) ) ;
#129650=CARTESIAN_POINT ( 'NONE',  ( 5.551115123125782702E-14, 64.35000000001120668, -3.023107484524792277 ) ) ;
#129651=EDGE_LOOP ( 'NONE', ( #160383, #255872, #21325, #199353 ) ) ;
#129698=CARTESIAN_POINT ( 'NONE',  ( 11.60000000000006004, 63.75000000001119815, -21.02310748452479316 ) ) ;
#129806=ORIENTED_EDGE ( 'NONE', *, *, #198246, .F. ) ;
#129812=CARTESIAN_POINT ( 'NONE',  ( 23.40000000000005542, 87.51781941433023349, -34.28670414799875488 ) ) ;
#129823=FACE_OUTER_BOUND ( 'NONE', #14601, .T. ) ;
#129840=ORIENTED_EDGE ( 'NONE', *, *, #249137, .T. ) ;
#129872=AXIS2_PLACEMENT_3D ( 'NONE', #3588, #27044, #201787 ) ;
#129892=TOROIDAL_SURFACE ( 'NONE', #885, 2.699999999999999734, 0.1000000000000000056 ) ;
#129921=CARTESIAN_POINT ( 'NONE',  ( -21.14999999999994174, 83.90000000001120384, -37.27310748452479316 ) ) ;
#129953=CARTESIAN_POINT ( 'NONE',  ( 0.9000000000000547562, 64.25000000001119815, -10.02310748452479139 ) ) ;
#129994=DIRECTION ( 'NONE',  ( 0.000000000000000000, -1.000000000000000000, 0.000000000000000000 ) ) ;
#130002=CARTESIAN_POINT ( 'NONE',  ( -23.39999999999994529, 76.00000000001119815, -36.02310748452479316 ) ) ;
#130061=DIRECTION ( 'NONE',  ( 0.000000000000000000, 0.9910827722268055195, -0.1332476588733540468 ) ) ;
#130064=ORIENTED_EDGE ( 'NONE', *, *, #55824, .T. ) ;
#130089=LINE ( 'NONE', #71431, #213443 ) ;
#130164=ORIENTED_EDGE ( 'NONE', *, *, #246286, .F. ) ;
#130192=EDGE_LOOP ( 'NONE', ( #234917, #150534, #186658, #45442 ) ) ;
#130204=ORIENTED_EDGE ( 'NONE', *, *, #79933, .F. ) ;
#130237=DIRECTION ( 'NONE',  ( -2.889348024582214003E-15, -0.9910827722268042983, -0.1332476588733650935 ) ) ;
#130248=LINE ( 'NONE', #110701, #250956 ) ;
#130267=DIRECTION ( 'NONE',  ( 0.000000000000000000, 0.000000000000000000, -1.000000000000000000 ) ) ;
#130332=EDGE_LOOP ( 'NONE', ( #49265, #212830, #27350, #219305 ) ) ;
#130403=DIRECTION ( 'NONE',  ( 0.000000000000000000, 0.000000000000000000, 1.000000000000000000 ) ) ;
#130412=AXIS2_PLACEMENT_3D ( 'NONE', #37314, #93408, #232955 ) ;
#130420=VECTOR ( 'NONE', #67103, 1000.000000000000000 ) ;
#130445=VERTEX_POINT ( 'NONE', #122715 ) ;
#130521=CARTESIAN_POINT ( 'NONE',  ( -6.099999999999939249, 64.35000000001120668, -25.92310748452479174 ) ) ;
#130540=ORIENTED_EDGE ( 'NONE', *, *, #142766, .F. ) ;
#130547=CARTESIAN_POINT ( 'NONE',  ( 20.95000000000005258, 64.35000000001119247, -6.123107484524794586 ) ) ;
#130573=ORIENTED_EDGE ( 'NONE', *, *, #126282, .F. ) ;
#130579=LINE ( 'NONE', #211417, #234760 ) ;
#130584=ORIENTED_EDGE ( 'NONE', *, *, #127295, .F. ) ;
#130662=FACE_OUTER_BOUND ( 'NONE', #249969, .T. ) ;
#130669=ORIENTED_EDGE ( 'NONE', *, *, #201013, .F. ) ;
#130718=TOROIDAL_SURFACE ( 'NONE', #26702, 2.699999999999999734, 0.1000000000000000056 ) ;
#130741=DIRECTION ( 'NONE',  ( 0.000000000000000000, -1.000000000000000000, 0.000000000000000000 ) ) ;
#130788=ORIENTED_EDGE ( 'NONE', *, *, #201013, .T. ) ;
#130841=CARTESIAN_POINT ( 'NONE',  ( -20.94999999999994600, 66.15000000001120384, -4.523107484524794053 ) ) ;
#130843=DIRECTION ( 'NONE',  ( 0.000000000000000000, -1.000000000000000000, 8.673617379884042375E-16 ) ) ;
#130916=AXIS2_PLACEMENT_3D ( 'NONE', #50417, #27060, #146955 ) ;
#130930=EDGE_LOOP ( 'NONE', ( #140157, #244323, #97787, #138343 ) ) ;
#130940=DIRECTION ( 'NONE',  ( 1.000000000000000000, 0.000000000000000000, 0.000000000000000000 ) ) ;
#130942=AXIS2_PLACEMENT_3D ( 'NONE', #99145, #58, #39222 ) ;
#130972=ORIENTED_EDGE ( 'NONE', *, *, #34730, .F. ) ;
#131028=DIRECTION ( 'NONE',  ( -1.000000000000000000, 5.467925025959462129E-15, -3.427148797533442008E-14 ) ) ;
#131131=ORIENTED_EDGE ( 'NONE', *, *, #77273, .T. ) ;
#131132=AXIS2_PLACEMENT_3D ( 'NONE', #111057, #134451, #109761 ) ;
#131144=LINE ( 'NONE', #172893, #103749 ) ;
#131202=FACE_OUTER_BOUND ( 'NONE', #136425, .T. ) ;
#131232=( GEOMETRIC_REPRESENTATION_CONTEXT ( 3 ) GLOBAL_UNCERTAINTY_ASSIGNED_CONTEXT ( ( #225138 ) ) GLOBAL_UNIT_ASSIGNED_CONTEXT ( ( #185556, #129436, #30352 ) ) REPRESENTATION_CONTEXT ( 'NONE', 'WORKASPACE' ) );
#131310=AXIS2_PLACEMENT_3D ( 'NONE', #1363, #237431, #40555 ) ;
#131342=LINE ( 'NONE', #214727, #141074 ) ;
#131459=VERTEX_POINT ( 'NONE', #192018 ) ;
#131474=DIRECTION ( 'NONE',  ( -1.000000000000000000, 0.000000000000000000, -0.000000000000000000 ) ) ;
#131637=DIRECTION ( 'NONE',  ( -0.000000000000000000, -0.4856429311786365499, -0.8741572761215353760 ) ) ;
#131721=ORIENTED_EDGE ( 'NONE', *, *, #94673, .T. ) ;
#131741=EDGE_CURVE ( 'NONE', #76432, #61312, #154443, .T. ) ;
#131837=ADVANCED_FACE ( 'NONE', ( #74353 ), #91318, .T. ) ;
#131851=VERTEX_POINT ( 'NONE', #114730 ) ;
#131879=CARTESIAN_POINT ( 'NONE',  ( 21.15000000000003055, 77.16254490893143725, -44.02310748452479316 ) ) ;
#131916=ORIENTED_EDGE ( 'NONE', *, *, #256781, .T. ) ;
#131957=ORIENTED_EDGE ( 'NONE', *, *, #73558, .F. ) ;
#131958=ADVANCED_FACE ( 'NONE', ( #97696 ), #40365, .T. ) ;
#131988=CIRCLE ( 'NONE', #156959, 0.1000000000000028644 ) ;
#132003=ORIENTED_EDGE ( 'NONE', *, *, #96629, .F. ) ;
#132013=CARTESIAN_POINT ( 'NONE',  ( 21.15000000000005542, 74.63923853664559260, -43.99645795275012006 ) ) ;
#132029=AXIS2_PLACEMENT_3D ( 'NONE', #46019, #61740, #85114 ) ;
#132039=DIRECTION ( 'NONE',  ( -1.000000000000000000, 0.000000000000000000, 0.000000000000000000 ) ) ;
#132056=LINE ( 'NONE', #112507, #79076 ) ;
#132124=EDGE_LOOP ( 'NONE', ( #181170, #173238, #136308, #209853 ) ) ;
#132142=DIRECTION ( 'NONE',  ( 0.000000000000000000, -0.000000000000000000, -1.000000000000000000 ) ) ;
#132161=PRODUCT_DEFINITION_FORMATION_WITH_SPECIFIED_SOURCE ( 'ANY', '', #247102, .NOT_KNOWN. ) ;
#132197=AXIS2_PLACEMENT_3D ( 'NONE', #44141, #79389, #158977 ) ;
#132198=AXIS2_PLACEMENT_3D ( 'NONE', #71465, #50567, #32348 ) ;
#132225=TOROIDAL_SURFACE ( 'NONE', #19822, 0.2000000000000000111, 0.1000000000000000056 ) ;
#132304=DIRECTION ( 'NONE',  ( 0.000000000000000000, 0.000000000000000000, 1.000000000000000000 ) ) ;
#132468=CARTESIAN_POINT ( 'NONE',  ( -0.8999999999999430678, 67.65000000001118963, -5.981686128287480919 ) ) ;
#132487=DIRECTION ( 'NONE',  ( 0.000000000000000000, 0.000000000000000000, -1.000000000000000000 ) ) ;
#132692=DIRECTION ( 'NONE',  ( 1.000000000000000000, -0.000000000000000000, -0.000000000000000000 ) ) ;
#132748=AXIS2_PLACEMENT_3D ( 'NONE', #224453, #246585, #104486 ) ;
#132758=EDGE_CURVE ( 'NONE', #89464, #186471, #188090, .T. ) ;
#132780=CYLINDRICAL_SURFACE ( 'NONE', #180670, 0.09999999999999939493 ) ;
#132788=ORIENTED_EDGE ( 'NONE', *, *, #32906, .T. ) ;
#132825=CYLINDRICAL_SURFACE ( 'NONE', #41539, 2.600000000000000089 ) ;
#132835=ORIENTED_EDGE ( 'NONE', *, *, #207734, .F. ) ;
#132860=FACE_OUTER_BOUND ( 'NONE', #117185, .T. ) ;
#132887=LINE ( 'NONE', #134143, #122427 ) ;
#132903=CARTESIAN_POINT ( 'NONE',  ( -23.39999999999994529, 77.83551161375991967, -47.52760213295649550 ) ) ;
#132921=ORIENTED_EDGE ( 'NONE', *, *, #143594, .T. ) ;
#132923=VERTEX_POINT ( 'NONE', #95292 ) ;
#132927=CARTESIAN_POINT ( 'NONE',  ( -20.94999999999994600, 67.82483145523551116, -25.59432346794077162 ) ) ;
#132990=EDGE_LOOP ( 'NONE', ( #45972, #133712, #93094, #243670 ) ) ;
#133005=ORIENTED_EDGE ( 'NONE', *, *, #74434, .T. ) ;
#133067=ORIENTED_EDGE ( 'NONE', *, *, #224720, .T. ) ;
#133117=ORIENTED_EDGE ( 'NONE', *, *, #25457, .T. ) ;
#133160=DIRECTION ( 'NONE',  ( -0.000000000000000000, 0.000000000000000000, 1.000000000000000000 ) ) ;
#133164=PLANE ( 'NONE',  #255798 ) ;
#133173=DIRECTION ( 'NONE',  ( 0.000000000000000000, 0.000000000000000000, 1.000000000000000000 ) ) ;
#133189=ORIENTED_EDGE ( 'NONE', *, *, #29307, .T. ) ;
#133191=AXIS2_PLACEMENT_3D ( 'NONE', #99706, #41075, #155886 ) ;
#133203=ORIENTED_EDGE ( 'NONE', *, *, #209906, .F. ) ;
#133213=ORIENTED_EDGE ( 'NONE', *, *, #134347, .T. ) ;
#133307=DIRECTION ( 'NONE',  ( 0.000000000000000000, 0.000000000000000000, -1.000000000000000000 ) ) ;
#133332=VERTEX_POINT ( 'NONE', #175824 ) ;
#133479=DIRECTION ( 'NONE',  ( 0.000000000000000000, 0.000000000000000000, -1.000000000000000000 ) ) ;
#133490=AXIS2_PLACEMENT_3D ( 'NONE', #239698, #58457, #37663 ) ;
#133526=DIRECTION ( 'NONE',  ( -0.000000000000000000, -0.000000000000000000, -1.000000000000000000 ) ) ;
#133560=SHAPE_REPRESENTATION ( 'Moving End Attachment Flange', ( #2425 ), #197867 ) ;
#133681=CARTESIAN_POINT ( 'NONE',  ( 13.40000000000005898, 67.75000000001118394, -21.02310748452479316 ) ) ;
#133712=ORIENTED_EDGE ( 'NONE', *, *, #115090, .T. ) ;
#133723=ORIENTED_EDGE ( 'NONE', *, *, #116945, .T. ) ;
#133725=AXIS2_PLACEMENT_3D ( 'NONE', #41109, #116762, #80170 ) ;
#133750=EDGE_CURVE ( 'NONE', #231870, #186109, #17931, .T. ) ;
#133767=VERTEX_POINT ( 'NONE', #236733 ) ;
#133772=CYLINDRICAL_SURFACE ( 'NONE', #255677, 0.09999999999999939493 ) ;
#133811=CARTESIAN_POINT ( 'NONE',  ( 23.40000000000005187, 84.00000000001119815, -34.86056257560453986 ) ) ;
#133820=VERTEX_POINT ( 'NONE', #240602 ) ;
#133848=CARTESIAN_POINT ( 'NONE',  ( 20.95000000000005258, 65.15000000001120384, -3.023107484524792277 ) ) ;
#133877=AXIS2_PLACEMENT_3D ( 'NONE', #123791, #200755, #65093 ) ;
#133893=ORIENTED_EDGE ( 'NONE', *, *, #164203, .F. ) ;
#134004=CIRCLE ( 'NONE', #117267, 11.65000000000000036 ) ;
#134006=ORIENTED_EDGE ( 'NONE', *, *, #159555, .T. ) ;
#134079=DIRECTION ( 'NONE',  ( -0.000000000000000000, 1.156482317317873105E-15, 1.000000000000000000 ) ) ;
#134114=ORIENTED_EDGE ( 'NONE', *, *, #191615, .F. ) ;
#134143=CARTESIAN_POINT ( 'NONE',  ( 21.05000000000005400, 64.35000000001119247, -51.02310748452479316 ) ) ;
#134183=DIRECTION ( 'NONE',  ( 0.000000000000000000, 0.8741572761215442577, -0.4856429311786202851 ) ) ;
#134190=LINE ( 'NONE', #233328, #170946 ) ;
#134228=ORIENTED_EDGE ( 'NONE', *, *, #87371, .F. ) ;
#134254=DIRECTION ( 'NONE',  ( 1.000000000000000000, -0.000000000000000000, -0.000000000000000000 ) ) ;
#134334=CARTESIAN_POINT ( 'NONE',  ( -13.39999999999994529, 67.65000000001118963, -25.06452884076210452 ) ) ;
#134347=EDGE_CURVE ( 'NONE', #108159, #10047, #88842, .T. ) ;
#134421=CARTESIAN_POINT ( 'NONE',  ( 21.05000000000005400, 84.00000000001119815, -37.18565239344504647 ) ) ;
#134439=CARTESIAN_POINT ( 'NONE',  ( -21.04999999999994387, 69.83923505573476120, -35.48358590217651454 ) ) ;
#134451=DIRECTION ( 'NONE',  ( 0.000000000000000000, -0.1332476588733589040, 0.9910827722268049644 ) ) ;
#134479=DIRECTION ( 'NONE',  ( 0.000000000000000000, 0.000000000000000000, -1.000000000000000000 ) ) ;
#134496=ORIENTED_EDGE ( 'NONE', *, *, #73536, .T. ) ;
#134539=AXIS2_PLACEMENT_3D ( 'NONE', #175537, #33479, #152123 ) ;
#134551=LINE ( 'NONE', #15945, #20937 ) ;
#134560=FACE_OUTER_BOUND ( 'NONE', #111054, .T. ) ;
#134563=DIRECTION ( 'NONE',  ( 1.000000000000000000, 0.000000000000000000, 0.000000000000000000 ) ) ;
#134649=EDGE_CURVE ( 'NONE', #111962, #106794, #175869, .T. ) ;
#134658=VERTEX_POINT ( 'NONE', #183553 ) ;
#134659=FACE_OUTER_BOUND ( 'NONE', #235066, .T. ) ;
#134661=ORIENTED_EDGE ( 'NONE', *, *, #99862, .F. ) ;
#134698=VERTEX_POINT ( 'NONE', #122294 ) ;
#134741=EDGE_CURVE ( 'NONE', #109797, #187747, #180992, .T. ) ;
#134753=EDGE_CURVE ( 'NONE', #201487, #167224, #46943, .T. ) ;
#134771=VERTEX_POINT ( 'NONE', #53009 ) ;
#134792=CARTESIAN_POINT ( 'NONE',  ( 23.40000000000005187, 82.84256550613280012, -26.34830530078816935 ) ) ;
#134882=EDGE_LOOP ( 'NONE', ( #6947, #41280, #219458, #172019 ) ) ;
#134885=VECTOR ( 'NONE', #1647, 1000.000000000000000 ) ;
#134890=DIRECTION ( 'NONE',  ( -0.000000000000000000, -1.000000000000000000, -0.000000000000000000 ) ) ;
#134994=LINE ( 'NONE', #232858, #85732 ) ;
#135019=CARTESIAN_POINT ( 'NONE',  ( -40.23850191057533010, 65.25000000001119815, -51.02310748452479316 ) ) ;
#135072=CARTESIAN_POINT ( 'NONE',  ( -20.94999999999994600, 87.75000000001122658, -30.12310748452481235 ) ) ;
#135083=EDGE_LOOP ( 'NONE', ( #80220, #235430, #257250, #66817 ) ) ;
#135137=CARTESIAN_POINT ( 'NONE',  ( 0.9000000000000547562, 64.35000000001120668, -10.02310748452479139 ) ) ;
#135160=DIRECTION ( 'NONE',  ( 0.000000000000000000, 0.000000000000000000, 1.000000000000000000 ) ) ;
#135183=CARTESIAN_POINT ( 'NONE',  ( 0.9000000000000549782, 66.35000000001119247, -12.62310748452479281 ) ) ;
#135198=PLANE ( 'NONE',  #148293 ) ;
#135201=CIRCLE ( 'NONE', #151811, 0.09999999999999939493 ) ;
#135208=ORIENTED_EDGE ( 'NONE', *, *, #107769, .F. ) ;
#135247=CIRCLE ( 'NONE', #185150, 0.1000000000000021844 ) ;
#135314=CIRCLE ( 'NONE', #22926, 2.700000000000001066 ) ;
#135335=ORIENTED_EDGE ( 'NONE', *, *, #33437, .T. ) ;
#135372=VERTEX_POINT ( 'NONE', #43427 ) ;
#135395=CARTESIAN_POINT ( 'NONE',  ( 23.50000000000005684, 77.16254490893143725, -43.82310748452479743 ) ) ;
#135425=EDGE_LOOP ( 'NONE', ( #160503, #18655, #209873, #53018 ) ) ;
#135431=EDGE_CURVE ( 'NONE', #60123, #33086, #69425, .T. ) ;
#135462=VECTOR ( 'NONE', #205871, 1000.000000000000000 ) ;
#135476=CARTESIAN_POINT ( 'NONE',  ( -23.49999999999994316, 87.75000000001119815, -43.82310748452479743 ) ) ;
#135480=DIRECTION ( 'NONE',  ( 0.000000000000000000, -0.9910827722268041873, 0.1332476588733659539 ) ) ;
#135489=ORIENTED_EDGE ( 'NONE', *, *, #112028, .T. ) ;
#135511=DIRECTION ( 'NONE',  ( 0.000000000000000000, -0.9910827722268055195, 0.1332476588733540468 ) ) ;
#135514=DIRECTION ( 'NONE',  ( 1.000000000000000000, -0.000000000000000000, -0.000000000000000000 ) ) ;
#135538=AXIS2_PLACEMENT_3D ( 'NONE', #142223, #182658, #223043 ) ;
#135540=VERTEX_POINT ( 'NONE', #111099 ) ;
#135582=CARTESIAN_POINT ( 'NONE',  ( -23.49999999999994316, 64.25000000001119815, -36.02310748452479316 ) ) ;
#135623=DIRECTION ( 'NONE',  ( 1.000000000000000000, 0.000000000000000000, 0.000000000000000000 ) ) ;
#135637=LINE ( 'NONE', #40439, #195820 ) ;
#135725=FACE_OUTER_BOUND ( 'NONE', #158253, .T. ) ;
#135753=ORIENTED_EDGE ( 'NONE', *, *, #64746, .T. ) ;
#135761=VERTEX_POINT ( 'NONE', #85727 ) ;
#135766=ORIENTED_EDGE ( 'NONE', *, *, #214676, .F. ) ;
#135880=DIRECTION ( 'NONE',  ( 1.000000000000000000, 0.000000000000000000, 0.000000000000000000 ) ) ;
#135971=VERTEX_POINT ( 'NONE', #222243 ) ;
#135973=LINE ( 'NONE', #36933, #144715 ) ;
#136148=CIRCLE ( 'NONE', #152787, 0.09999999999999939493 ) ;
#136165=EDGE_LOOP ( 'NONE', ( #235976, #255188, #134496, #65523 ) ) ;
#136256=CIRCLE ( 'NONE', #65553, 0.09999999999999939493 ) ;
#136283=CARTESIAN_POINT ( 'NONE',  ( 21.05000000000005400, 85.52235250936195143, -34.45408804175119144 ) ) ;
#136285=DIRECTION ( 'NONE',  ( 0.000000000000000000, 1.000000000000000000, -0.000000000000000000 ) ) ;
#136307=CARTESIAN_POINT ( 'NONE',  ( 23.50000000000005684, 74.83745509109094485, -43.82310748452479743 ) ) ;
#136308=ORIENTED_EDGE ( 'NONE', *, *, #40544, .F. ) ;
#136318=AXIS2_PLACEMENT_3D ( 'NONE', #33715, #111941, #14126 ) ;
#136405=CARTESIAN_POINT ( 'NONE',  ( 21.15000000000005542, 86.36484105039212977, -51.23044614117323903 ) ) ;
#136421=STYLED_ITEM ( 'NONE', ( #127725 ), #190377 ) ;
#136425=EDGE_LOOP ( 'NONE', ( #185162, #90778, #183690, #159149 ) ) ;
#136469=VERTEX_POINT ( 'NONE', #188915 ) ;
#136588=DIRECTION ( 'NONE',  ( 0.000000000000000000, 0.000000000000000000, 1.000000000000000000 ) ) ;
#136683=DIRECTION ( 'NONE',  ( 0.000000000000000000, 0.000000000000000000, 1.000000000000000000 ) ) ;
#136716=AXIS2_PLACEMENT_3D ( 'NONE', #81095, #283, #160684 ) ;
#136729=DIRECTION ( 'NONE',  ( 0.000000000000000000, -0.000000000000000000, -1.000000000000000000 ) ) ;
#136747=CARTESIAN_POINT ( 'NONE',  ( -11.59999999999994458, 64.35000000001120668, -23.72310748452479245 ) ) ;
#136752=DIRECTION ( 'NONE',  ( 3.469446951953515108E-14, 1.000000000000000000, 0.000000000000000000 ) ) ;
#136776=DIRECTION ( 'NONE',  ( -3.469446951953515108E-14, 1.000000000000000000, 0.000000000000000000 ) ) ;
#136789=VECTOR ( 'NONE', #204008, 1000.000000000000114 ) ;
#136794=ORIENTED_EDGE ( 'NONE', *, *, #257500, .F. ) ;
#136799=PLANE ( 'NONE',  #159820 ) ;
#136826=DIRECTION ( 'NONE',  ( 0.000000000000000000, -0.7071067811865473507, -0.7071067811865477948 ) ) ;
#136884=ORIENTED_EDGE ( 'NONE', *, *, #36383, .F. ) ;
#136955=ORIENTED_EDGE ( 'NONE', *, *, #192409, .F. ) ;
#137023=DIRECTION ( 'NONE',  ( -1.000000000000000000, 0.000000000000000000, 0.000000000000000000 ) ) ;
#137070=DIRECTION ( 'NONE',  ( 0.000000000000000000, 0.000000000000000000, -1.000000000000000000 ) ) ;
#137074=ADVANCED_FACE ( 'NONE', ( #187990 ), #210128, .T. ) ;
#137079=EDGE_CURVE ( 'NONE', #225270, #144437, #148016, .T. ) ;
#137125=CARTESIAN_POINT ( 'NONE',  ( -20.94999999999994600, 64.35000000001119247, -6.023107484524794941 ) ) ;
#137140=DIRECTION ( 'NONE',  ( 0.000000000000000000, 0.000000000000000000, -1.000000000000000000 ) ) ;
#137146=CARTESIAN_POINT ( 'NONE',  ( -21.04999999999994387, 83.98667523412385094, -37.28476067066772970 ) ) ;
#137187=CYLINDRICAL_SURFACE ( 'NONE', #216200, 0.09999999999999982514 ) ;
#137199=CARTESIAN_POINT ( 'NONE',  ( -11.59999999999994458, 67.75000000001118394, -16.98168612828748181 ) ) ;
#137239=CARTESIAN_POINT ( 'NONE',  ( 23.50000000000005684, 64.25000000001119815, -43.82310748452479743 ) ) ;
#137272=DIRECTION ( 'NONE',  ( -0.000000000000000000, -0.000000000000000000, 1.000000000000000000 ) ) ;
#137320=VERTEX_POINT ( 'NONE', #199563 ) ;
#137325=VECTOR ( 'NONE', #152681, 1000.000000000000114 ) ;
#137369=CARTESIAN_POINT ( 'NONE',  ( -21.14999999999994174, 74.83745509109094485, -44.02310748452479316 ) ) ;
#137418=EDGE_CURVE ( 'NONE', #50827, #21187, #24780, .T. ) ;
#137503=DIRECTION ( 'NONE',  ( 1.000000000000000000, 0.000000000000000000, 0.000000000000000000 ) ) ;
#137581=ADVANCED_FACE ( 'NONE', ( #255287 ), #172006, .F. ) ;
#137645=EDGE_LOOP ( 'NONE', ( #253477, #199433, #122203, #89113 ) ) ;
#137677=CYLINDRICAL_SURFACE ( 'NONE', #117299, 0.09999999999999939493 ) ;
#137706=DIRECTION ( 'NONE',  ( 0.000000000000000000, -0.9910827722268055195, -0.1332476588733540468 ) ) ;
#137720=ORIENTED_EDGE ( 'NONE', *, *, #34162, .T. ) ;
#137730=EDGE_LOOP ( 'NONE', ( #131916, #74649, #147233, #3418 ) ) ;
#137805=CARTESIAN_POINT ( 'NONE',  ( -21.14999999999994174, 82.74366731733570646, -26.36310895752070138 ) ) ;
#137831=CARTESIAN_POINT ( 'NONE',  ( -20.94999999999994600, 64.35000000001120668, -30.12310748452479103 ) ) ;
#137869=FACE_OUTER_BOUND ( 'NONE', #86663, .T. ) ;
#137936=ORIENTED_EDGE ( 'NONE', *, *, #171891, .F. ) ;
#137951=CARTESIAN_POINT ( 'NONE',  ( 5.900000000000059863, 64.65000000001120384, -25.92310748452479174 ) ) ;
#137954=EDGE_CURVE ( 'NONE', #90057, #160549, #146969, .T. ) ;
#137955=CYLINDRICAL_SURFACE ( 'NONE', #508, 0.09999999999999939493 ) ;
#138062=FACE_OUTER_BOUND ( 'NONE', #158105, .T. ) ;
#138076=CARTESIAN_POINT ( 'NONE',  ( -20.94999999999994600, 66.15000000001120384, -5.923107484524795296 ) ) ;
#138081=DIRECTION ( 'NONE',  ( -0.000000000000000000, 0.1332476588733665090, 0.9910827722268039652 ) ) ;
#138162=ADVANCED_FACE ( 'NONE', ( #22870 ), #123228, .T. ) ;
#138172=EDGE_CURVE ( 'NONE', #231379, #187553, #185767, .T. ) ;
#138196=ORIENTED_EDGE ( 'NONE', *, *, #117310, .T. ) ;
#138199=EDGE_CURVE ( 'NONE', #32708, #74886, #47517, .T. ) ;
#138227=ORIENTED_EDGE ( 'NONE', *, *, #174167, .T. ) ;
#138323=ORIENTED_EDGE ( 'NONE', *, *, #80351, .F. ) ;
#138343=ORIENTED_EDGE ( 'NONE', *, *, #252772, .F. ) ;
#138441=DIRECTION ( 'NONE',  ( 0.000000000000000000, 1.000000000000000000, 0.000000000000000000 ) ) ;
#138475=DIRECTION ( 'NONE',  ( -1.000000000000000000, 0.000000000000000000, 0.000000000000000000 ) ) ;
#138506=EDGE_CURVE ( 'NONE', #44045, #243775, #102045, .T. ) ;
#138522=EDGE_CURVE ( 'NONE', #252227, #45216, #182910, .T. ) ;
#138527=LINE ( 'NONE', #201097, #148184 ) ;
#138533=EDGE_CURVE ( 'NONE', #46490, #90293, #147170, .T. ) ;
#138536=ORIENTED_EDGE ( 'NONE', *, *, #108446, .T. ) ;
#138567=CARTESIAN_POINT ( 'NONE',  ( -0.8999999999999437339, 64.35000000001120668, -12.62310748452478926 ) ) ;
#138595=AXIS2_PLACEMENT_3D ( 'NONE', #13239, #212719, #133173 ) ;
#138646=ORIENTED_EDGE ( 'NONE', *, *, #108525, .T. ) ;
#138665=EDGE_CURVE ( 'NONE', #109797, #90507, #51647, .T. ) ;
#138675=CIRCLE ( 'NONE', #255183, 0.1999999999999996503 ) ;
#138689=DIRECTION ( 'NONE',  ( -1.000000000000000000, -0.000000000000000000, -0.000000000000000000 ) ) ;
#138717=EDGE_CURVE ( 'NONE', #235335, #99842, #132887, .T. ) ;
#138725=TOROIDAL_SURFACE ( 'NONE', #213591, 11.65000000000000036, 0.1000000000000000056 ) ;
#138738=EDGE_LOOP ( 'NONE', ( #114372, #9533, #135335 ) ) ;
#138772=SPHERICAL_SURFACE ( 'NONE', #167131, 0.1000000000000000056 ) ;
#138784=CARTESIAN_POINT ( 'NONE',  ( 21.15000000000005542, 77.83551161375993388, -47.52760213295649550 ) ) ;
#138797=DIRECTION ( 'NONE',  ( -0.000000000000000000, 0.000000000000000000, 1.000000000000000000 ) ) ;
#138811=ADVANCED_FACE ( 'NONE', ( #178447 ), #139262, .T. ) ;
#138839=CARTESIAN_POINT ( 'NONE',  ( 23.40000000000005187, 83.90000000001120384, -34.77310748452479316 ) ) ;
#138903=CARTESIAN_POINT ( 'NONE',  ( 13.40000000000005898, 66.35000000001119247, -18.42310748452479530 ) ) ;
#138905=VECTOR ( 'NONE', #1480, 1000.000000000000000 ) ;
#138930=TOROIDAL_SURFACE ( 'NONE', #184756, 4.150000000000000355, 0.1000000000000000056 ) ;
#138943=DIRECTION ( 'NONE',  ( 1.000000000000000000, 0.000000000000000000, 0.000000000000000000 ) ) ;
#138950=ORIENTED_EDGE ( 'NONE', *, *, #127295, .T. ) ;
#138954=DIRECTION ( 'NONE',  ( 0.000000000000000000, 0.000000000000000000, -1.000000000000000000 ) ) ;
#138977=CARTESIAN_POINT ( 'NONE',  ( 0.9000000000000546452, 67.75000000001118394, -5.981686128287480919 ) ) ;
#139003=ORIENTED_EDGE ( 'NONE', *, *, #162331, .F. ) ;
#139018=ORIENTED_EDGE ( 'NONE', *, *, #218031, .F. ) ;
#139031=ORIENTED_EDGE ( 'NONE', *, *, #96953, .F. ) ;
#139050=PLANE ( 'NONE',  #56482 ) ;
#139070=EDGE_LOOP ( 'NONE', ( #43675, #204027, #79717, #113016 ) ) ;
#139084=ADVANCED_FACE ( 'NONE', ( #212113 ), #172541, .T. ) ;
#139130=VERTEX_POINT ( 'NONE', #249944 ) ;
#139154=CIRCLE ( 'NONE', #6077, 0.1000000000000002554 ) ;
#139157=CARTESIAN_POINT ( 'NONE',  ( 11.60000000000006004, 64.35000000001120668, -18.32310748452479388 ) ) ;
#139200=VECTOR ( 'NONE', #93686, 1000.000000000000000 ) ;
#139227=DIRECTION ( 'NONE',  ( 1.000000000000000000, -0.000000000000000000, -0.000000000000000000 ) ) ;
#139242=AXIS2_PLACEMENT_3D ( 'NONE', #47100, #67970, #109651 ) ;
#139248=AXIS2_PLACEMENT_3D ( 'NONE', #248124, #168648, #246833 ) ;
#139253=DIRECTION ( 'NONE',  ( -0.000000000000000000, 1.000000000000000000, -0.000000000000000000 ) ) ;
#139256=DIRECTION ( 'NONE',  ( 0.000000000000000000, 0.000000000000000000, -1.000000000000000000 ) ) ;
#139257=ORIENTED_EDGE ( 'NONE', *, *, #239062, .T. ) ;
#139262=CYLINDRICAL_SURFACE ( 'NONE', #230761, 0.1000000000000028644 ) ;
#139324=VERTEX_POINT ( 'NONE', #43731 ) ;
#139354=EDGE_LOOP ( 'NONE', ( #39628, #147320, #73914, #188258 ) ) ;
#139357=ADVANCED_FACE ( 'NONE', ( #127117 ), #46282, .T. ) ;
#139395=ADVANCED_FACE ( 'NONE', ( #25467 ), #255241, .F. ) ;
#139400=DIRECTION ( 'NONE',  ( 1.000000000000000000, 0.000000000000000000, 0.000000000000000000 ) ) ;
#139493=ORIENTED_EDGE ( 'NONE', *, *, #133750, .F. ) ;
#139505=ADVANCED_FACE ( 'NONE', ( #149276 ), #213070, .F. ) ;
#139529=DIRECTION ( 'NONE',  ( 0.000000000000000000, -0.9910827722268049644, 0.1332476588733589318 ) ) ;
#139562=VERTEX_POINT ( 'NONE', #110121 ) ;
#139564=FACE_OUTER_BOUND ( 'NONE', #76098, .T. ) ;
#139565=CYLINDRICAL_SURFACE ( 'NONE', #113689, 0.09999999999999530098 ) ;
#139606=VECTOR ( 'NONE', #77918, 1000.000000000000000 ) ;
#139618=VECTOR ( 'NONE', #90557, 1000.000000000000000 ) ;
#139638=CARTESIAN_POINT ( 'NONE',  ( 23.40000000000005187, 82.78482233730476025, -26.42994920107286916 ) ) ;
#139645=CARTESIAN_POINT ( 'NONE',  ( 23.40000000000005187, 76.00000000001119815, -36.02310748452479316 ) ) ;
#139661=DIRECTION ( 'NONE',  ( 0.000000000000000000, 0.000000000000000000, 1.000000000000000000 ) ) ;
#139730=DIRECTION ( 'NONE',  ( -0.000000000000000000, 1.000000000000000000, -0.000000000000000000 ) ) ;
#139787=ORIENTED_EDGE ( 'NONE', *, *, #178344, .F. ) ;
#139827=AXIS2_PLACEMENT_3D ( 'NONE', #15224, #192567, #210845 ) ;
#139837=EDGE_CURVE ( 'NONE', #19078, #182432, #151460, .T. ) ;
#139849=CARTESIAN_POINT ( 'NONE',  ( -23.49999999999994316, 83.98667523412385094, -34.76145429838185663 ) ) ;
#140014=ORIENTED_EDGE ( 'NONE', *, *, #65408, .T. ) ;
#140068=CARTESIAN_POINT ( 'NONE',  ( -21.14999999999994174, 76.00000000001119815, -36.02310748452479316 ) ) ;
#140081=ADVANCED_FACE ( 'NONE', ( #17074 ), #35134, .F. ) ;
#140082=LINE ( 'NONE', #99660, #90689 ) ;
#140087=ORIENTED_EDGE ( 'NONE', *, *, #193020, .F. ) ;
#140104=CIRCLE ( 'NONE', #256776, 0.1000000000000021844 ) ;
#140105=CARTESIAN_POINT ( 'NONE',  ( 23.40000000000005187, 64.25000000001119815, -51.02310748452479316 ) ) ;
#140110=DIRECTION ( 'NONE',  ( 0.000000000000000000, 1.000000000000000000, -0.000000000000000000 ) ) ;
#140113=CARTESIAN_POINT ( 'NONE',  ( 21.15000000000005542, 83.97335046823651794, -34.66234602115918051 ) ) ;
#140142=ORIENTED_EDGE ( 'NONE', *, *, #256615, .F. ) ;
#140157=ORIENTED_EDGE ( 'NONE', *, *, #124509, .F. ) ;
#140248=ORIENTED_EDGE ( 'NONE', *, *, #141265, .F. ) ;
#140262=FACE_BOUND ( 'NONE', #5797, .T. ) ;
#140289=CARTESIAN_POINT ( 'NONE',  ( 0.9000000000000546452, 67.65000000001118963, -14.06452884076210630 ) ) ;
#140323=EDGE_CURVE ( 'NONE', #60723, #82975, #163005, .T. ) ;
#140358=DIRECTION ( 'NONE',  ( 1.000000000000000000, 0.000000000000000000, 0.000000000000000000 ) ) ;
#140413=CIRCLE ( 'NONE', #103000, 0.09999999999999939493 ) ;
#140524=DIRECTION ( 'NONE',  ( 0.000000000000000000, 1.181088324069315448E-15, 1.000000000000000000 ) ) ;
#140529=ORIENTED_EDGE ( 'NONE', *, *, #257733, .T. ) ;
#140534=CIRCLE ( 'NONE', #40643, 0.09999999999999939493 ) ;
#140543=CIRCLE ( 'NONE', #190477, 11.74999999999999645 ) ;
#140585=EDGE_CURVE ( 'NONE', #89464, #114288, #185765, .T. ) ;
#140601=EDGE_CURVE ( 'NONE', #128152, #62001, #239284, .T. ) ;
#140612=VECTOR ( 'NONE', #608, 1000.000000000000000 ) ;
#140614=FACE_OUTER_BOUND ( 'NONE', #134882, .T. ) ;
#140730=DIRECTION ( 'NONE',  ( 0.000000000000000000, -0.000000000000000000, -1.000000000000000000 ) ) ;
#140737=DIRECTION ( 'NONE',  ( 0.000000000000000000, -0.000000000000000000, 1.000000000000000000 ) ) ;
#140820=DIRECTION ( 'NONE',  ( 1.000000000000000000, 0.000000000000000000, -0.000000000000000000 ) ) ;
#140866=FACE_OUTER_BOUND ( 'NONE', #139354, .T. ) ;
#140869=ORIENTED_EDGE ( 'NONE', *, *, #252133, .T. ) ;
#140897=ADVANCED_FACE ( 'NONE', ( #19985 ), #100739, .T. ) ;
#140898=VECTOR ( 'NONE', #81102, 1000.000000000000000 ) ;
#140942=LINE ( 'NONE', #215326, #28545 ) ;
#140983=ORIENTED_EDGE ( 'NONE', *, *, #40228, .F. ) ;
#141002=ORIENTED_EDGE ( 'NONE', *, *, #193789, .F. ) ;
#141012=DIRECTION ( 'NONE',  ( 0.000000000000000000, 0.000000000000000000, -1.000000000000000000 ) ) ;
#141032=CIRCLE ( 'NONE', #111988, 0.1000000000000028644 ) ;
#141059=FACE_OUTER_BOUND ( 'NONE', #157591, .T. ) ;
#141074=VECTOR ( 'NONE', #192609, 1000.000000000000000 ) ;
#141126=CARTESIAN_POINT ( 'NONE',  ( -0.8999999999999425127, 67.72071067812984779, -13.99381816264344813 ) ) ;
#141134=VECTOR ( 'NONE', #222850, 1000.000000000000000 ) ;
#141176=ADVANCED_FACE ( 'NONE', ( #112359 ), #250560, .T. ) ;
#141179=DIRECTION ( 'NONE',  ( 0.000000000000000000, 0.000000000000000000, 1.000000000000000000 ) ) ;
#141182=CARTESIAN_POINT ( 'NONE',  ( -5.899999999999938183, 64.75000000001119815, -22.02310748452479316 ) ) ;
#141197=CARTESIAN_POINT ( 'NONE',  ( 21.15000000000005187, 74.14873292176677921, -47.62635315998165453 ) ) ;
#141217=CIRCLE ( 'NONE', #28843, 0.1000000000000028644 ) ;
#141241=EDGE_CURVE ( 'NONE', #88024, #128131, #202060, .T. ) ;
#141265=EDGE_CURVE ( 'NONE', #30110, #187156, #160573, .T. ) ;
#141277=DIRECTION ( 'NONE',  ( -1.000000000000000000, 0.000000000000000000, 0.000000000000000000 ) ) ;
#141300=ORIENTED_EDGE ( 'NONE', *, *, #167427, .T. ) ;
#141321=LINE ( 'NONE', #106018, #35334 ) ;
#141344=DIRECTION ( 'NONE',  ( 0.000000000000000000, 0.000000000000000000, 1.000000000000000000 ) ) ;
#141358=DIRECTION ( 'NONE',  ( 0.000000000000000000, -0.9910827722268049644, 0.1332476588733589040 ) ) ;
#141419=DIRECTION ( 'NONE',  ( 1.000000000000000000, 0.000000000000000000, 0.000000000000000000 ) ) ;
#141476=LINE ( 'NONE', #7097, #11109 ) ;
#141525=ORIENTED_EDGE ( 'NONE', *, *, #237074, .F. ) ;
#141576=DIRECTION ( 'NONE',  ( -8.673617379883787770E-15, -1.000000000000000000, 0.000000000000000000 ) ) ;
#141651=AXIS2_PLACEMENT_3D ( 'NONE', #150322, #130741, #207731 ) ;
#141656=EDGE_LOOP ( 'NONE', ( #160531, #170150, #220909, #204906 ) ) ;
#141693=ORIENTED_EDGE ( 'NONE', *, *, #149757, .T. ) ;
#141723=EDGE_LOOP ( 'NONE', ( #98493, #115158, #170002, #228202 ) ) ;
#141779=DIRECTION ( 'NONE',  ( 1.000000000000000000, 0.000000000000000000, 0.000000000000000000 ) ) ;
#141785=DIRECTION ( 'NONE',  ( -1.000000000000000000, -0.000000000000000000, -0.000000000000000000 ) ) ;
#141797=ORIENTED_EDGE ( 'NONE', *, *, #182060, .F. ) ;
#141802=DIRECTION ( 'NONE',  ( 0.000000000000000000, -1.000000000000000000, 0.000000000000000000 ) ) ;
#141843=ORIENTED_EDGE ( 'NONE', *, *, #164203, .T. ) ;
#141859=VERTEX_POINT ( 'NONE', #42769 ) ;
#141909=ORIENTED_EDGE ( 'NONE', *, *, #75557, .F. ) ;
#141928=AXIS2_PLACEMENT_3D ( 'NONE', #9575, #12178, #193380 ) ;
#141956=CIRCLE ( 'NONE', #305, 4.900000000000001243 ) ;
#142028=DIRECTION ( 'NONE',  ( 1.000000000000000000, 0.000000000000000000, 0.000000000000000000 ) ) ;
#142056=VECTOR ( 'NONE', #180786, 1000.000000000000114 ) ;
#142061=ORIENTED_EDGE ( 'NONE', *, *, #108751, .T. ) ;
#142070=EDGE_CURVE ( 'NONE', #23626, #145505, #81755, .T. ) ;
#142085=CARTESIAN_POINT ( 'NONE',  ( 21.15000000000005542, 77.16254490893143725, -43.92310748452479885 ) ) ;
#142091=DIRECTION ( 'NONE',  ( 0.000000000000000000, 1.000000000000000000, 0.000000000000000000 ) ) ;
#142165=AXIS2_PLACEMENT_3D ( 'NONE', #149747, #12805, #148452 ) ;
#142168=ORIENTED_EDGE ( 'NONE', *, *, #30027, .T. ) ;
#142203=ORIENTED_EDGE ( 'NONE', *, *, #166224, .F. ) ;
#142223=CARTESIAN_POINT ( 'NONE',  ( 23.40000000000005542, 78.05591623545335267, -49.16694968567509250 ) ) ;
#142238=EDGE_LOOP ( 'NONE', ( #163473, #165616, #208814, #19740 ) ) ;
#142322=DIRECTION ( 'NONE',  ( 1.000000000000000000, -0.000000000000000000, 0.000000000000000000 ) ) ;
#142377=ORIENTED_EDGE ( 'NONE', *, *, #80584, .T. ) ;
#142400=CARTESIAN_POINT ( 'NONE',  ( 21.15000000000005542, 83.90000000001120384, -37.18565239344504647 ) ) ;
#142419=DIRECTION ( 'NONE',  ( 0.000000000000000000, -1.000000000000000000, 0.000000000000000000 ) ) ;
#142471=CARTESIAN_POINT ( 'NONE',  ( 23.40000000000005187, 83.90000000001120384, -34.77310748452479316 ) ) ;
#142485=ORIENTED_EDGE ( 'NONE', *, *, #17871, .F. ) ;
#142536=EDGE_CURVE ( 'NONE', #88642, #241392, #164360, .T. ) ;
#142541=DIRECTION ( 'NONE',  ( 0.000000000000000000, -1.000000000000000000, 0.000000000000000000 ) ) ;
#142624=DIRECTION ( 'NONE',  ( 0.000000000000000000, -0.1332476588733448597, -0.9910827722268067408 ) ) ;
#142648=FACE_OUTER_BOUND ( 'NONE', #142759, .T. ) ;
#142662=EDGE_CURVE ( 'NONE', #114575, #168296, #157017, .T. ) ;
#142686=DIRECTION ( 'NONE',  ( 0.000000000000000000, 0.000000000000000000, 1.000000000000000000 ) ) ;
#142759=EDGE_LOOP ( 'NONE', ( #130788, #82881, #206627, #42705 ) ) ;
#142766=EDGE_CURVE ( 'NONE', #60596, #202492, #198019, .T. ) ;
#142789=CONICAL_SURFACE ( 'NONE', #30416, 4.000000000000000000, 0.7853981633974489451 ) ;
#142791=VECTOR ( 'NONE', #201822, 1000.000000000000114 ) ;
#142800=CARTESIAN_POINT ( 'NONE',  ( 23.40000000000005542, 77.83551161375991967, -47.52760213295649550 ) ) ;
#142869=EDGE_CURVE ( 'NONE', #153832, #45216, #140413, .T. ) ;
#142966=CYLINDRICAL_SURFACE ( 'NONE', #165610, 0.09999999999999939493 ) ;
#142985=FACE_OUTER_BOUND ( 'NONE', #179797, .T. ) ;
#143059=AXIS2_PLACEMENT_3D ( 'NONE', #145345, #68393, #201466 ) ;
#143089=ORIENTED_EDGE ( 'NONE', *, *, #141241, .F. ) ;
#143103=ORIENTED_EDGE ( 'NONE', *, *, #197515, .T. ) ;
#143107=LINE ( 'NONE', #201808, #185089 ) ;
#143120=FACE_OUTER_BOUND ( 'NONE', #112621, .T. ) ;
#143202=CARTESIAN_POINT ( 'NONE',  ( -11.59999999999994458, 67.65000000001118963, -25.06452884076210452 ) ) ;
#143259=CARTESIAN_POINT ( 'NONE',  ( -21.14999999999994174, 77.83551161375991967, -47.52760213295649550 ) ) ;
#143353=DIRECTION ( 'NONE',  ( 0.000000000000000000, 0.000000000000000000, 1.000000000000000000 ) ) ;
#143369=EDGE_CURVE ( 'NONE', #101028, #135761, #28221, .T. ) ;
#143382=ORIENTED_EDGE ( 'NONE', *, *, #129131, .T. ) ;
#143436=ORIENTED_EDGE ( 'NONE', *, *, #199609, .F. ) ;
#143490=VERTEX_POINT ( 'NONE', #230118 ) ;
#143497=CIRCLE ( 'NONE', #31119, 0.1000000000000028644 ) ;
#143594=EDGE_CURVE ( 'NONE', #68170, #111962, #95003, .T. ) ;
#143602=ORIENTED_EDGE ( 'NONE', *, *, #242816, .T. ) ;
#143683=ORIENTED_EDGE ( 'NONE', *, *, #44961, .T. ) ;
#143799=EDGE_LOOP ( 'NONE', ( #29860, #50498, #145794, #147253 ) ) ;
#143829=DIRECTION ( 'NONE',  ( 0.000000000000000000, 0.000000000000000000, 1.000000000000000000 ) ) ;
#143837=ORIENTED_EDGE ( 'NONE', *, *, #32906, .F. ) ;
#143862=EDGE_LOOP ( 'NONE', ( #243281, #71643, #25901 ) ) ;
#143932=VERTEX_POINT ( 'NONE', #127459 ) ;
#143934=DIRECTION ( 'NONE',  ( 0.000000000000000000, 0.9910827722268055195, -0.1332476588733540468 ) ) ;
#143938=DIRECTION ( 'NONE',  ( 0.000000000000000000, -0.1332476588733448597, -0.9910827722268067408 ) ) ;
#143949=LINE ( 'NONE', #223480, #6800 ) ;
#143983=ORIENTED_EDGE ( 'NONE', *, *, #142869, .F. ) ;
#144006=EDGE_CURVE ( 'NONE', #46490, #230635, #28608, .T. ) ;
#144016=VERTEX_POINT ( 'NONE', #169186 ) ;
#144039=CYLINDRICAL_SURFACE ( 'NONE', #2988, 0.1000000000000002554 ) ;
#144068=ORIENTED_EDGE ( 'NONE', *, *, #214901, .F. ) ;
#144092=AXIS2_PLACEMENT_3D ( 'NONE', #217397, #236988, #34973 ) ;
#144115=CIRCLE ( 'NONE', #102407, 0.09999999999999635569 ) ;
#144132=CARTESIAN_POINT ( 'NONE',  ( -23.39999999999994529, 83.90000000001120384, -34.77310748452479316 ) ) ;
#144140=DIRECTION ( 'NONE',  ( 0.000000000000000000, 0.000000000000000000, -1.000000000000000000 ) ) ;
#144149=DIRECTION ( 'NONE',  ( -1.000000000000000000, 0.000000000000000000, 0.000000000000000000 ) ) ;
#144177=VERTEX_POINT ( 'NONE', #153496 ) ;
#144198=FACE_OUTER_BOUND ( 'NONE', #143799, .T. ) ;
#144331=FACE_OUTER_BOUND ( 'NONE', #96099, .T. ) ;
#144427=DIRECTION ( 'NONE',  ( 0.000000000000000000, 0.000000000000000000, -1.000000000000000000 ) ) ;
#144437=VERTEX_POINT ( 'NONE', #249676 ) ;
#144490=CARTESIAN_POINT ( 'NONE',  ( 21.15000000000005187, 64.25000000001119815, -30.12310748452479103 ) ) ;
#144521=AXIS2_PLACEMENT_3D ( 'NONE', #195528, #54700, #172129 ) ;
#144554=AXIS2_PLACEMENT_3D ( 'NONE', #194613, #255794, #14693 ) ;
#144655=CIRCLE ( 'NONE', #190667, 0.09999999999999530098 ) ;
#144705=EDGE_CURVE ( 'NONE', #96904, #216036, #186403, .T. ) ;
#144715=VECTOR ( 'NONE', #17341, 1000.000000000000114 ) ;
#144788=CIRCLE ( 'NONE', #40795, 4.049999999999998046 ) ;
#144818=VERTEX_POINT ( 'NONE', #52429 ) ;
#144840=DIRECTION ( 'NONE',  ( 0.000000000000000000, 0.000000000000000000, 1.000000000000000000 ) ) ;
#144850=ORIENTED_EDGE ( 'NONE', *, *, #169316, .F. ) ;
#144879=DIRECTION ( 'NONE',  ( 1.000000000000000000, 0.000000000000000000, 0.000000000000000000 ) ) ;
#144899=LINE ( 'NONE', #207479, #192242 ) ;
#144943=EDGE_CURVE ( 'NONE', #170938, #81245, #240083, .T. ) ;
#144952=CIRCLE ( 'NONE', #24177, 0.1999999999999987899 ) ;
#144955=FACE_OUTER_BOUND ( 'NONE', #167443, .T. ) ;
#144989=DIRECTION ( 'NONE',  ( 0.000000000000000000, -1.387778780781454006E-13, 1.000000000000000000 ) ) ;
#145042=ORIENTED_EDGE ( 'NONE', *, *, #18076, .F. ) ;
#145053=ORIENTED_EDGE ( 'NONE', *, *, #74787, .F. ) ;
#145066=CARTESIAN_POINT ( 'NONE',  ( 23.50000000000005684, 64.25000000001119815, -3.123107484524795474 ) ) ;
#145119=ORIENTED_EDGE ( 'NONE', *, *, #190146, .T. ) ;
#145345=CARTESIAN_POINT ( 'NONE',  ( -21.14999999999994174, 78.11805852053666399, -49.62915779269638961 ) ) ;
#145443=CARTESIAN_POINT ( 'NONE',  ( 21.05000000000005400, 77.16254490893143725, -44.02310748452479316 ) ) ;
#145498=DIRECTION ( 'NONE',  ( -0.000000000000000000, 1.000000000000000000, -0.000000000000000000 ) ) ;
#145505=VERTEX_POINT ( 'NONE', #55323 ) ;
#145573=DIRECTION ( 'NONE',  ( -1.000000000000000000, 4.624352451196580357E-15, 3.439547145395922042E-14 ) ) ;
#145598=AXIS2_PLACEMENT_3D ( 'NONE', #136747, #177206, #241005 ) ;
#145623=CIRCLE ( 'NONE', #33244, 0.1000000000000028644 ) ;
#145634=DIRECTION ( 'NONE',  ( 0.000000000000000000, 0.000000000000000000, -1.000000000000000000 ) ) ;
#145651=DIRECTION ( 'NONE',  ( 0.000000000000000000, 0.000000000000000000, 1.000000000000000000 ) ) ;
#145670=DIRECTION ( 'NONE',  ( -1.000000000000000000, 0.000000000000000000, 0.000000000000000000 ) ) ;
#145724=DIRECTION ( 'NONE',  ( -0.000000000000000000, 1.000000000000000000, 0.000000000000000000 ) ) ;
#145794=ORIENTED_EDGE ( 'NONE', *, *, #12239, .F. ) ;
#145828=CARTESIAN_POINT ( 'NONE',  ( 23.40000000000005187, 77.83551161375991967, -47.52760213295649550 ) ) ;
#145830=DIRECTION ( 'NONE',  ( 0.000000000000000000, 0.000000000000000000, 1.000000000000000000 ) ) ;
#145853=ADVANCED_FACE ( 'NONE', ( #85155 ), #44789, .F. ) ;
#145856=CARTESIAN_POINT ( 'NONE',  ( 21.05000000000005400, 87.75000000001119815, -51.02310748452479316 ) ) ;
#145952=CARTESIAN_POINT ( 'NONE',  ( 23.40000000000005542, 83.97335046823651794, -34.66234602115918051 ) ) ;
#146031=CIRCLE ( 'NONE', #75151, 0.09999999999999939493 ) ;
#146087=EDGE_CURVE ( 'NONE', #169204, #40901, #56325, .T. ) ;
#146157=CARTESIAN_POINT ( 'NONE',  ( -11.59999999999994458, 67.75000000001118394, -23.62310748452479103 ) ) ;
#146220=VERTEX_POINT ( 'NONE', #47032 ) ;
#146240=DIRECTION ( 'NONE',  ( 1.000000000000000000, -0.000000000000000000, 0.000000000000000000 ) ) ;
#146299=CARTESIAN_POINT ( 'NONE',  ( 6.000000000000060396, 64.75000000001119815, -26.02310748452479316 ) ) ;
#146308=ORIENTED_EDGE ( 'NONE', *, *, #192515, .T. ) ;
#146317=DIRECTION ( 'NONE',  ( -1.000000000000000000, -0.000000000000000000, -0.000000000000000000 ) ) ;
#146318=EDGE_CURVE ( 'NONE', #141859, #82762, #50878, .T. ) ;
#146329=CARTESIAN_POINT ( 'NONE',  ( 6.100000000000060929, 64.25000000001119815, -25.92310748452479174 ) ) ;
#146341=AXIS2_PLACEMENT_3D ( 'NONE', #155760, #189720, #249695 ) ;
#146380=LINE ( 'NONE', #229790, #60081 ) ;
#146397=CARTESIAN_POINT ( 'NONE',  ( -21.04999999999994387, 67.75000000001118394, -4.623107484524796362 ) ) ;
#146448=AXIS2_PLACEMENT_3D ( 'NONE', #83357, #185051, #247597 ) ;
#146463=CARTESIAN_POINT ( 'NONE',  ( 21.15000000000005187, 76.00000000001119815, -36.02310748452479316 ) ) ;
#146474=DIRECTION ( 'NONE',  ( 0.000000000000000000, 0.000000000000000000, 1.000000000000000000 ) ) ;
#146490=DIRECTION ( 'NONE',  ( 0.000000000000000000, 0.1332476588733636502, 0.9910827722268044093 ) ) ;
#146502=FACE_OUTER_BOUND ( 'NONE', #169350, .T. ) ;
#146517=DIRECTION ( 'NONE',  ( 0.000000000000000000, 0.000000000000000000, -1.000000000000000000 ) ) ;
#146600=DIRECTION ( 'NONE',  ( 0.000000000000000000, 0.000000000000000000, -1.000000000000000000 ) ) ;
#146608=VECTOR ( 'NONE', #119231, 1000.000000000000000 ) ;
#146672=CARTESIAN_POINT ( 'NONE',  ( 23.40000000000005542, 85.84984265665381997, -47.78991727088349251 ) ) ;
#146674=LINE ( 'NONE', #185827, #192583 ) ;
#146691=VECTOR ( 'NONE', #49277, 1000.000000000000000 ) ;
#146774=EDGE_CURVE ( 'NONE', #158981, #186471, #168024, .T. ) ;
#146789=DIRECTION ( 'NONE',  ( -1.000000000000000000, -0.000000000000000000, 0.000000000000000000 ) ) ;
#146804=EDGE_LOOP ( 'NONE', ( #212155, #99163, #14054, #211243 ) ) ;
#146828=AXIS2_PLACEMENT_3D ( 'NONE', #202924, #244614, #108951 ) ;
#146845=FACE_OUTER_BOUND ( 'NONE', #78640, .T. ) ;
#146860=AXIS2_PLACEMENT_3D ( 'NONE', #214230, #298, #175150 ) ;
#146907=CYLINDRICAL_SURFACE ( 'NONE', #248520, 0.09999999999999982514 ) ;
#146955=DIRECTION ( 'NONE',  ( -1.000000000000000000, 0.000000000000000000, 0.000000000000000000 ) ) ;
#146969=CIRCLE ( 'NONE', #34585, 5.000000000000000888 ) ;
#147018=DIRECTION ( 'NONE',  ( -0.000000000000000000, -0.1332476588733650935, 0.9910827722268042983 ) ) ;
#147039=DIRECTION ( 'NONE',  ( 0.000000000000000000, -1.000000000000000000, -0.000000000000000000 ) ) ;
#147051=DIRECTION ( 'NONE',  ( 1.000000000000000000, 0.000000000000000000, 0.000000000000000000 ) ) ;
#147080=CARTESIAN_POINT ( 'NONE',  ( -13.39999999999994529, 67.75000000001118394, -21.02310748452479316 ) ) ;
#147086=CARTESIAN_POINT ( 'NONE',  ( -13.39999999999994529, 63.75000000001119815, -21.02310748452479316 ) ) ;
#147112=ADVANCED_FACE ( 'NONE', ( #153139 ), #91837, .F. ) ;
#147135=LINE ( 'NONE', #165438, #235373 ) ;
#147170=CIRCLE ( 'NONE', #13905, 0.1000000000000028644 ) ;
#147213=AXIS2_PLACEMENT_3D ( 'NONE', #93443, #129994, #173042 ) ;
#147233=ORIENTED_EDGE ( 'NONE', *, *, #80351, .T. ) ;
#147237=CARTESIAN_POINT ( 'NONE',  ( 23.40000000000005542, 77.26165318615413469, -44.00978271863746016 ) ) ;
#147247=VERTEX_POINT ( 'NONE', #423 ) ;
#147253=ORIENTED_EDGE ( 'NONE', *, *, #199839, .F. ) ;
#147287=CARTESIAN_POINT ( 'NONE',  ( 0.9000000000000547562, 67.72071067812984779, -6.052396806406134644 ) ) ;
#147299=VECTOR ( 'NONE', #128490, 1000.000000000000000 ) ;
#147320=ORIENTED_EDGE ( 'NONE', *, *, #167446, .T. ) ;
#147388=CARTESIAN_POINT ( 'NONE',  ( 21.15000000000005542, 74.83745509109094485, -43.92310748452479885 ) ) ;
#147418=EDGE_CURVE ( 'NONE', #252143, #250175, #23129, .T. ) ;
#147461=EDGE_CURVE ( 'NONE', #168923, #123853, #181537, .T. ) ;
#147477=AXIS2_PLACEMENT_3D ( 'NONE', #91434, #167150, #211382 ) ;
#147488=CIRCLE ( 'NONE', #251533, 11.75000000000000000 ) ;
#147507=DIRECTION ( 'NONE',  ( 0.000000000000000000, 0.000000000000000000, 1.000000000000000000 ) ) ;
#147527=AXIS2_PLACEMENT_3D ( 'NONE', #100415, #35375, #60011 ) ;
#147595=DIRECTION ( 'NONE',  ( 0.000000000000000000, 0.9889818879709272315, 0.1480365673253073999 ) ) ;
#147611=ORIENTED_EDGE ( 'NONE', *, *, #251225, .T. ) ;
#147697=CARTESIAN_POINT ( 'NONE',  ( 21.15000000000005542, 87.75000000001119815, -43.82310748452479743 ) ) ;
#147730=DIRECTION ( 'NONE',  ( -1.000000000000000000, 0.000000000000000000, 0.000000000000000000 ) ) ;
#147737=FACE_OUTER_BOUND ( 'NONE', #186023, .T. ) ;
#147746=EDGE_CURVE ( 'NONE', #109039, #130445, #123076, .T. ) ;
#147758=ADVANCED_FACE ( 'NONE', ( #42713 ), #64981, .T. ) ;
#147759=ORIENTED_EDGE ( 'NONE', *, *, #199748, .F. ) ;
#147773=CARTESIAN_POINT ( 'NONE',  ( 20.95000000000005258, 65.19115966511134275, -29.92310748452479174 ) ) ;
#147879=ADVANCED_FACE ( 'NONE', ( #92108 ), #88228, .T. ) ;
#147907=LINE ( 'NONE', #27983, #136789 ) ;
#147910=CARTESIAN_POINT ( 'NONE',  ( -21.14999999999994174, 87.50449464844290048, -37.85861909827351468 ) ) ;
#147922=DIRECTION ( 'NONE',  ( 0.000000000000000000, 0.000000000000000000, -1.000000000000000000 ) ) ;
#147924=DIRECTION ( 'NONE',  ( 0.000000000000000000, 0.000000000000000000, -1.000000000000000000 ) ) ;
#147934=ADVANCED_FACE ( 'NONE', ( #50389 ), #171684, .T. ) ;
#147939=CARTESIAN_POINT ( 'NONE',  ( -11.59999999999994458, 64.25000000001119815, -18.32310748452479388 ) ) ;
#147975=EDGE_LOOP ( 'NONE', ( #92795, #61678, #133203, #25928 ) ) ;
#148011=VECTOR ( 'NONE', #98734, 1000.000000000000114 ) ;
#148016=CIRCLE ( 'NONE', #68940, 0.1000000000000028644 ) ;
#148064=AXIS2_PLACEMENT_3D ( 'NONE', #29320, #188352, #213046 ) ;
#148084=CARTESIAN_POINT ( 'NONE',  ( 23.40000000000005187, 64.25000000001119815, -3.123107484524795474 ) ) ;
#148089=CARTESIAN_POINT ( 'NONE',  ( -5.899999999999938183, 64.35000000001120668, -22.02310748452479316 ) ) ;
#148107=ORIENTED_EDGE ( 'NONE', *, *, #24991, .T. ) ;
#148109=CARTESIAN_POINT ( 'NONE',  ( 21.05000000000005400, 67.73741572762334329, -25.54575917482290848 ) ) ;
#148149=SPHERICAL_SURFACE ( 'NONE', #245268, 0.1000000000000000056 ) ;
#148154=EDGE_LOOP ( 'NONE', ( #37270, #24407, #5436, #160999 ) ) ;
#148184=VECTOR ( 'NONE', #198526, 1000.000000000000000 ) ;
#148239=AXIS2_PLACEMENT_3D ( 'NONE', #20731, #100217, #3706 ) ;
#148293=AXIS2_PLACEMENT_3D ( 'NONE', #217300, #16574, #58229 ) ;
#148304=EDGE_LOOP ( 'NONE', ( #125689, #125499, #154506, #99715 ) ) ;
#148422=DIRECTION ( 'NONE',  ( 0.000000000000000000, 1.000000000000000000, 0.000000000000000000 ) ) ;
#148435=ORIENTED_EDGE ( 'NONE', *, *, #17466, .T. ) ;
#148452=DIRECTION ( 'NONE',  ( 1.000000000000000000, 0.000000000000000000, 0.000000000000000000 ) ) ;
#148497=EDGE_CURVE ( 'NONE', #17064, #32708, #131988, .T. ) ;
#148502=DIRECTION ( 'NONE',  ( -1.000000000000000000, 0.000000000000000000, 0.000000000000000000 ) ) ;
#148506=CIRCLE ( 'NONE', #231713, 0.09999999999999635569 ) ;
#148520=DIRECTION ( 'NONE',  ( 0.000000000000000000, 0.000000000000000000, 1.000000000000000000 ) ) ;
#148639=ORIENTED_EDGE ( 'NONE', *, *, #91788, .F. ) ;
#148649=LINE ( 'NONE', #165646, #83556 ) ;
#148664=CARTESIAN_POINT ( 'NONE',  ( 5.900000000000060751, 64.25000000001119815, -22.02310748452479316 ) ) ;
#148669=VERTEX_POINT ( 'NONE', #64879 ) ;
#148671=CARTESIAN_POINT ( 'NONE',  ( 20.95000000000005258, 66.15000000001114699, -51.02310748452476474 ) ) ;
#148719=AXIS2_PLACEMENT_3D ( 'NONE', #220820, #196131, #100832 ) ;
#148720=ADVANCED_FACE ( 'NONE', ( #143120 ), #222658, .T. ) ;
#148744=VERTEX_POINT ( 'NONE', #227803 ) ;
#148776=FACE_OUTER_BOUND ( 'NONE', #18526, .T. ) ;
#148787=CIRCLE ( 'NONE', #11995, 0.09999999999999982514 ) ;
#148792=CARTESIAN_POINT ( 'NONE',  ( -23.39999999999994529, 74.25000000001119815, -47.64205752314703801 ) ) ;
#148847=DIRECTION ( 'NONE',  ( 0.000000000000000000, 0.000000000000000000, -1.000000000000000000 ) ) ;
#148873=DIRECTION ( 'NONE',  ( 1.000000000000000000, 0.000000000000000000, 0.000000000000000000 ) ) ;
#148924=EDGE_CURVE ( 'NONE', #167941, #251797, #165509, .T. ) ;
#148931=ORIENTED_EDGE ( 'NONE', *, *, #147418, .T. ) ;
#148981=VECTOR ( 'NONE', #13048, 1000.000000000000000 ) ;
#148987=EDGE_CURVE ( 'NONE', #122992, #113629, #190465, .T. ) ;
#148993=EDGE_LOOP ( 'NONE', ( #88583, #24207, #40474, #128467 ) ) ;
#148994=CARTESIAN_POINT ( 'NONE',  ( 21.05000000000005400, 76.00000000001119815, -40.17310748452479174 ) ) ;
#149012=VERTEX_POINT ( 'NONE', #99818 ) ;
#149040=DIRECTION ( 'NONE',  ( 0.000000000000000000, 0.000000000000000000, -1.000000000000000000 ) ) ;
#149049=AXIS2_PLACEMENT_3D ( 'NONE', #243028, #6987, #106064 ) ;
#149050=DIRECTION ( 'NONE',  ( 0.000000000000000000, 0.000000000000000000, -1.000000000000000000 ) ) ;
#149065=ORIENTED_EDGE ( 'NONE', *, *, #207913, .F. ) ;
#149067=EDGE_LOOP ( 'NONE', ( #23976, #16419, #257441, #89622 ) ) ;
#149132=DIRECTION ( 'NONE',  ( 0.000000000000000000, 0.000000000000000000, 1.000000000000000000 ) ) ;
#149141=EDGE_CURVE ( 'NONE', #84197, #50827, #140534, .T. ) ;
#149215=EDGE_CURVE ( 'NONE', #80255, #40557, #111420, .T. ) ;
#149244=ORIENTED_EDGE ( 'NONE', *, *, #147418, .F. ) ;
#149273=AXIS2_PLACEMENT_3D ( 'NONE', #132927, #151204, #134183 ) ;
#149276=FACE_OUTER_BOUND ( 'NONE', #219855, .T. ) ;
#149317=TOROIDAL_SURFACE ( 'NONE', #91040, 11.65000000000000036, 0.1000000000000000056 ) ;
#149485=DIRECTION ( 'NONE',  ( -1.000000000000000000, 0.000000000000000000, 0.000000000000000000 ) ) ;
#149490=FACE_OUTER_BOUND ( 'NONE', #214886, .T. ) ;
#149501=CARTESIAN_POINT ( 'NONE',  ( -11.59999999999994458, 64.35000000001120668, -18.42310748452479174 ) ) ;
#149507=CARTESIAN_POINT ( 'NONE',  ( -23.49999999999994316, 74.16448838626247664, -47.52760213295649550 ) ) ;
#149523=CARTESIAN_POINT ( 'NONE',  ( 23.40000000000005542, 64.35000000001120668, -3.023107484524792277 ) ) ;
#149568=CARTESIAN_POINT ( 'NONE',  ( 11.60000000000006182, 67.72071067812984779, -24.99381816264344636 ) ) ;
#149592=ADVANCED_FACE ( 'NONE', ( #130662 ), #15865, .T. ) ;
#149598=VECTOR ( 'NONE', #245850, 1000.000000000000000 ) ;
#149644=CIRCLE ( 'NONE', #166226, 0.09999999999999939493 ) ;
#149659=CARTESIAN_POINT ( 'NONE',  ( -21.14999999999994174, 82.84256550613280012, -26.34830530078816935 ) ) ;
#149747=CARTESIAN_POINT ( 'NONE',  ( -21.14999999999994174, 77.83551161375991967, -47.52760213295649550 ) ) ;
#149757=EDGE_CURVE ( 'NONE', #117140, #1657, #17164, .T. ) ;
#149787=AXIS2_PLACEMENT_3D ( 'NONE', #184388, #44892, #222212 ) ;
#149851=PLANE ( 'NONE',  #235129 ) ;
#149881=CARTESIAN_POINT ( 'NONE',  ( -23.49999999999994316, 64.25000000001119815, -26.12310748452479103 ) ) ;
#149943=CARTESIAN_POINT ( 'NONE',  ( -20.94999999999994600, 65.36599112033563586, -30.02023607076051803 ) ) ;
#150068=DIRECTION ( 'NONE',  ( 1.000000000000000000, 0.000000000000000000, 0.000000000000000000 ) ) ;
#150092=EDGE_CURVE ( 'NONE', #85754, #30250, #230765, .T. ) ;
#150104=DIRECTION ( 'NONE',  ( 0.000000000000000000, 0.000000000000000000, 1.000000000000000000 ) ) ;
#150118=AXIS2_PLACEMENT_3D ( 'NONE', #124913, #225258, #123626 ) ;
#150150=VERTEX_POINT ( 'NONE', #251592 ) ;
#150158=ADVANCED_FACE ( 'NONE', ( #53393 ), #14293, .T. ) ;
#150217=CIRCLE ( 'NONE', #191926, 0.1000000000000032391 ) ;
#150226=ORIENTED_EDGE ( 'NONE', *, *, #39101, .T. ) ;
#150228=CIRCLE ( 'NONE', #75218, 0.1000000000000002554 ) ;
#150322=CARTESIAN_POINT ( 'NONE',  ( 11.60000000000006004, 64.35000000001120668, -21.02310748452479316 ) ) ;
#150408=DIRECTION ( 'NONE',  ( 1.000000000000000000, 0.000000000000000000, -0.000000000000000000 ) ) ;
#150426=DIRECTION ( 'NONE',  ( -1.000000000000000000, 0.000000000000000000, 0.000000000000000000 ) ) ;
#150448=DIRECTION ( 'NONE',  ( -1.000000000000000000, 0.000000000000000000, -0.000000000000000000 ) ) ;
#150450=VECTOR ( 'NONE', #220119, 1000.000000000000000 ) ;
#150478=DIRECTION ( 'NONE',  ( 1.000000000000000000, 0.000000000000000000, 0.000000000000000000 ) ) ;
#150481=FACE_OUTER_BOUND ( 'NONE', #128053, .T. ) ;
#150534=ORIENTED_EDGE ( 'NONE', *, *, #30027, .F. ) ;
#150535=CARTESIAN_POINT ( 'NONE',  ( 20.95000000000005258, 87.75000000001119815, -5.923107484524795296 ) ) ;
#150587=ADVANCED_FACE ( 'NONE', ( #94446 ), #21361, .T. ) ;
#150606=LINE ( 'NONE', #187179, #149598 ) ;
#150613=CYLINDRICAL_SURFACE ( 'NONE', #152580, 0.1000000000000002554 ) ;
#150745=VERTEX_POINT ( 'NONE', #6904 ) ;
#150757=CIRCLE ( 'NONE', #242336, 11.65000000000000036 ) ;
#150776=CARTESIAN_POINT ( 'NONE',  ( 20.95000000000005258, 87.75000000001122658, -30.12310748452481235 ) ) ;
#150781=LINE ( 'NONE', #71266, #17899 ) ;
#150788=CARTESIAN_POINT ( 'NONE',  ( -20.94999999999994600, 65.19115966511134275, -30.02310748452479316 ) ) ;
#150790=ORIENTED_EDGE ( 'NONE', *, *, #29502, .F. ) ;
#150792=EDGE_CURVE ( 'NONE', #197543, #36158, #66883, .T. ) ;
#150809=LINE ( 'NONE', #208237, #36010 ) ;
#150828=VERTEX_POINT ( 'NONE', #48595 ) ;
#150835=ORIENTED_EDGE ( 'NONE', *, *, #134741, .F. ) ;
#150918=CIRCLE ( 'NONE', #234113, 0.09999999999999939493 ) ;
#150965=CYLINDRICAL_SURFACE ( 'NONE', #4675, 5.000000000000000888 ) ;
#150991=CARTESIAN_POINT ( 'NONE',  ( 23.40000000000005187, 64.35000000001120668, -3.123107484524795474 ) ) ;
#151034=DIRECTION ( 'NONE',  ( 1.000000000000000000, -0.000000000000000000, -0.000000000000000000 ) ) ;
#151074=ORIENTED_EDGE ( 'NONE', *, *, #189550, .F. ) ;
#151127=CARTESIAN_POINT ( 'NONE',  ( -23.39999999999994529, 87.50449464844290048, -37.85861909827351468 ) ) ;
#151172=EDGE_CURVE ( 'NONE', #34933, #135540, #211652, .T. ) ;
#151204=DIRECTION ( 'NONE',  ( -0.000000000000000000, -0.4856429311786292224, -0.8741572761215394838 ) ) ;
#151252=LINE ( 'NONE', #170859, #161306 ) ;
#151253=ORIENTED_EDGE ( 'NONE', *, *, #197695, .F. ) ;
#151366=DIRECTION ( 'NONE',  ( 0.000000000000000000, 0.000000000000000000, -1.000000000000000000 ) ) ;
#151460=CIRCLE ( 'NONE', #68232, 0.09999999999999939493 ) ;
#151508=CARTESIAN_POINT ( 'NONE',  ( -0.8999999999999430678, 63.75000000001118394, -10.02310748452479139 ) ) ;
#151527=CARTESIAN_POINT ( 'NONE',  ( -23.49999999999994316, 82.84256550613280012, -26.34830530078816935 ) ) ;
#151576=DIRECTION ( 'NONE',  ( 0.000000000000000000, -1.000000000000000000, 0.000000000000000000 ) ) ;
#151679=VERTEX_POINT ( 'NONE', #219660 ) ;
#151696=ORIENTED_EDGE ( 'NONE', *, *, #90867, .T. ) ;
#151717=CARTESIAN_POINT ( 'NONE',  ( -21.14999999999994174, 87.50449464844290048, -34.18759587077607165 ) ) ;
#151768=ORIENTED_EDGE ( 'NONE', *, *, #61404, .T. ) ;
#151811=AXIS2_PLACEMENT_3D ( 'NONE', #122553, #27331, #24752 ) ;
#151826=ORIENTED_EDGE ( 'NONE', *, *, #107280, .F. ) ;
#151838=DIRECTION ( 'NONE',  ( 0.000000000000000000, -1.000000000000000000, 0.000000000000000000 ) ) ;
#151864=EDGE_CURVE ( 'NONE', #19078, #29322, #175160, .T. ) ;
#151885=EDGE_CURVE ( 'NONE', #221278, #77791, #12117, .T. ) ;
#151917=EDGE_CURVE ( 'NONE', #14829, #105984, #78698, .T. ) ;
#151999=EDGE_CURVE ( 'NONE', #88201, #60723, #313, .T. ) ;
#152047=DIRECTION ( 'NONE',  ( -1.000000000000000000, -0.000000000000000000, -0.000000000000000000 ) ) ;
#152055=ORIENTED_EDGE ( 'NONE', *, *, #13960, .F. ) ;
#152079=ORIENTED_EDGE ( 'NONE', *, *, #168388, .T. ) ;
#152080=PRODUCT_DEFINITION ( 'UNKNOWN', '', #132161, #240885 ) ;
#152123=DIRECTION ( 'NONE',  ( 0.000000000000000000, 0.9910827722268055195, 0.1332476588733540468 ) ) ;
#152151=EDGE_CURVE ( 'NONE', #88024, #195816, #45594, .T. ) ;
#152190=EDGE_CURVE ( 'NONE', #128152, #60123, #45866, .T. ) ;
#152201=ORIENTED_EDGE ( 'NONE', *, *, #83837, .T. ) ;
#152205=EDGE_CURVE ( 'NONE', #189995, #3592, #33153, .T. ) ;
#152215=DIRECTION ( 'NONE',  ( -0.000000000000000000, 1.156482317317873105E-15, 1.000000000000000000 ) ) ;
#152224=ORIENTED_EDGE ( 'NONE', *, *, #40076, .F. ) ;
#152277=CARTESIAN_POINT ( 'NONE',  ( 23.50000000000005684, 76.00000000001119815, -36.02310748452479316 ) ) ;
#152279=ORIENTED_EDGE ( 'NONE', *, *, #77036, .F. ) ;
#152296=AXIS2_PLACEMENT_3D ( 'NONE', #71026, #127118, #224917 ) ;
#152374=AXIS2_PLACEMENT_3D ( 'NONE', #123655, #238457, #164062 ) ;
#152376=DIRECTION ( 'NONE',  ( 0.000000000000000000, 0.000000000000000000, 1.000000000000000000 ) ) ;
#152377=AXIS2_PLACEMENT_3D ( 'NONE', #135072, #252454, #115521 ) ;
#152403=ORIENTED_EDGE ( 'NONE', *, *, #17368, .T. ) ;
#152404=DIRECTION ( 'NONE',  ( -0.000000000000000000, -0.000000000000000000, -1.000000000000000000 ) ) ;
#152438=DIRECTION ( 'NONE',  ( 0.000000000000000000, 0.000000000000000000, 1.000000000000000000 ) ) ;
#152440=VECTOR ( 'NONE', #215108, 1000.000000000000000 ) ;
#152532=DIRECTION ( 'NONE',  ( -1.000000000000000000, 0.000000000000000000, 0.000000000000000000 ) ) ;
#152537=AXIS2_PLACEMENT_3D ( 'NONE', #133848, #36051, #191290 ) ;
#152561=EDGE_LOOP ( 'NONE', ( #56373, #25838, #106897, #142485 ) ) ;
#152580=AXIS2_PLACEMENT_3D ( 'NONE', #33263, #112766, #55318 ) ;
#152602=LINE ( 'NONE', #212558, #152440 ) ;
#152603=CARTESIAN_POINT ( 'NONE',  ( 23.40000000000005542, 74.16448838626247664, -47.52760213295649550 ) ) ;
#152631=DIRECTION ( 'NONE',  ( 1.000000000000000000, -0.000000000000000000, -0.000000000000000000 ) ) ;
#152681=DIRECTION ( 'NONE',  ( -0.000000000000000000, -0.1332476588733589318, -0.9910827722268049644 ) ) ;
#152687=ORIENTED_EDGE ( 'NONE', *, *, #82999, .F. ) ;
#152756=VECTOR ( 'NONE', #158932, 1000.000000000000114 ) ;
#152787=AXIS2_PLACEMENT_3D ( 'NONE', #65349, #203582, #245288 ) ;
#152793=ORIENTED_EDGE ( 'NONE', *, *, #29307, .F. ) ;
#152869=CARTESIAN_POINT ( 'NONE',  ( -11.59999999999994458, 63.75000000001119815, -21.02310748452479316 ) ) ;
#152883=DIRECTION ( 'NONE',  ( -0.000000000000000000, 0.9910827722268049644, 0.1332476588733589318 ) ) ;
#152926=ADVANCED_FACE ( 'NONE', ( #160085 ), #200476, .F. ) ;
#152962=AXIS2_PLACEMENT_3D ( 'NONE', #159716, #61896, #241808 ) ;
#153003=ORIENTED_EDGE ( 'NONE', *, *, #238942, .T. ) ;
#153011=DIRECTION ( 'NONE',  ( -0.000000000000000000, 0.9910827722268049644, 0.1332476588733589040 ) ) ;
#153017=DIRECTION ( 'NONE',  ( -0.000000000000000000, 1.000000000000000000, 0.000000000000000000 ) ) ;
#153040=VERTEX_POINT ( 'NONE', #30848 ) ;
#153043=EDGE_LOOP ( 'NONE', ( #176841, #55388, #163343, #99269 ) ) ;
#153062=EDGE_CURVE ( 'NONE', #92271, #122419, #250152, .T. ) ;
#153113=CIRCLE ( 'NONE', #173968, 0.09999999999999939493 ) ;
#153139=FACE_OUTER_BOUND ( 'NONE', #128637, .T. ) ;
#153174=DIRECTION ( 'NONE',  ( 1.000000000000000000, 0.000000000000000000, 0.000000000000000000 ) ) ;
#153179=CARTESIAN_POINT ( 'NONE',  ( -40.23850191057533010, 65.27857539272349641, -29.97167177764265489 ) ) ;
#153185=AXIS2_PLACEMENT_3D ( 'NONE', #235877, #157684, #1099 ) ;
#153238=DIRECTION ( 'NONE',  ( 0.000000000000000000, 0.1332476588733448597, 0.9910827722268067408 ) ) ;
#153269=EDGE_CURVE ( 'NONE', #249539, #215142, #21231, .T. ) ;
#153402=ORIENTED_EDGE ( 'NONE', *, *, #61233, .F. ) ;
#153418=ORIENTED_EDGE ( 'NONE', *, *, #42097, .T. ) ;
#153436=EDGE_LOOP ( 'NONE', ( #63922, #432, #152224, #150835 ) ) ;
#153496=CARTESIAN_POINT ( 'NONE',  ( -0.8999999999999438449, 67.72071067812984779, -6.052396806406134644 ) ) ;
#153500=DIRECTION ( 'NONE',  ( -1.000000000000000000, 0.000000000000000000, -0.000000000000000000 ) ) ;
#153513=CARTESIAN_POINT ( 'NONE',  ( 0.000000000000000000, 0.000000000000000000, 0.000000000000000000 ) ) ;
#153524=ORIENTED_EDGE ( 'NONE', *, *, #175669, .T. ) ;
#153552=DIRECTION ( 'NONE',  ( -1.000000000000000000, 0.000000000000000000, 0.000000000000000000 ) ) ;
#153585=AXIS2_PLACEMENT_3D ( 'NONE', #151527, #253157, #137070 ) ;
#153764=CARTESIAN_POINT ( 'NONE',  ( 23.40000000000005187, 76.00000000001119815, -36.02310748452479316 ) ) ;
#153785=VECTOR ( 'NONE', #203894, 1000.000000000000000 ) ;
#153802=ORIENTED_EDGE ( 'NONE', *, *, #201979, .T. ) ;
#153809=DIRECTION ( 'NONE',  ( 0.000000000000000000, 0.000000000000000000, -1.000000000000000000 ) ) ;
#153828=EDGE_LOOP ( 'NONE', ( #167248, #10959, #82358, #202888 ) ) ;
#153832=VERTEX_POINT ( 'NONE', #231965 ) ;
#153843=ORIENTED_EDGE ( 'NONE', *, *, #229330, .F. ) ;
#153954=ADVANCED_FACE ( 'NONE', ( #256582 ), #237079, .T. ) ;
#153959=EDGE_LOOP ( 'NONE', ( #138227, #105514, #232068, #12665 ) ) ;
#153976=ADVANCED_FACE ( 'NONE', ( #58406 ), #137955, .T. ) ;
#153982=CARTESIAN_POINT ( 'NONE',  ( -21.14999999999994174, 74.25000000001119815, -47.64205752314703801 ) ) ;
#153983=EDGE_CURVE ( 'NONE', #253379, #14829, #112959, .T. ) ;
#153989=ORIENTED_EDGE ( 'NONE', *, *, #144943, .F. ) ;
#154033=VERTEX_POINT ( 'NONE', #220082 ) ;
#154063=DIRECTION ( 'NONE',  ( 0.000000000000000000, -1.000000000000000000, 0.000000000000000000 ) ) ;
#154069=CARTESIAN_POINT ( 'NONE',  ( -21.14999999999994174, 85.92654454508293327, -48.30233646433089234 ) ) ;
#154089=ORIENTED_EDGE ( 'NONE', *, *, #84168, .T. ) ;
#154110=AXIS2_PLACEMENT_3D ( 'NONE', #43847, #4691, #50238 ) ;
#154157=DIRECTION ( 'NONE',  ( 0.000000000000000000, 0.000000000000000000, 1.000000000000000000 ) ) ;
#154169=EDGE_CURVE ( 'NONE', #238440, #113568, #25851, .T. ) ;
#154201=CARTESIAN_POINT ( 'NONE',  ( 0.9000000000000535350, 67.75000000001118394, -14.06452884076210630 ) ) ;
#154213=VECTOR ( 'NONE', #209872, 1000.000000000000000 ) ;
#154219=EDGE_LOOP ( 'NONE', ( #235564, #256617, #86557, #72582 ) ) ;
#154286=CARTESIAN_POINT ( 'NONE',  ( -23.39999999999994529, 83.90000000001120384, -34.86056257560453986 ) ) ;
#154376=ORIENTED_EDGE ( 'NONE', *, *, #117319, .T. ) ;
#154415=ORIENTED_EDGE ( 'NONE', *, *, #164724, .T. ) ;
#154443=CIRCLE ( 'NONE', #183634, 0.09999999999999939493 ) ;
#154468=ADVANCED_FACE ( 'NONE', ( #129524 ), #30437, .T. ) ;
#154506=ORIENTED_EDGE ( 'NONE', *, *, #78938, .F. ) ;
#154514=CIRCLE ( 'NONE', #83702, 0.1000000000000021844 ) ;
#154595=ADVANCED_FACE ( 'NONE', ( #45128 ), #124674, .F. ) ;
#154746=CARTESIAN_POINT ( 'NONE',  ( 23.40000000000005542, 87.50449464844290048, -34.18759587077607165 ) ) ;
#154759=CARTESIAN_POINT ( 'NONE',  ( -20.94999999999994600, 65.35000000001120668, -4.623107484524796362 ) ) ;
#154867=ORIENTED_EDGE ( 'NONE', *, *, #191514, .T. ) ;
#154934=DIRECTION ( 'NONE',  ( 1.000000000000000000, 0.000000000000000000, 0.000000000000000000 ) ) ;
#154999=DIRECTION ( 'NONE',  ( 0.000000000000000000, -0.9910827722268055195, 0.1332476588733540468 ) ) ;
#155024=ORIENTED_EDGE ( 'NONE', *, *, #55192, .F. ) ;
#155026=AXIS2_PLACEMENT_3D ( 'NONE', #4289, #205049, #26452 ) ;
#155031=VECTOR ( 'NONE', #207147, 1000.000000000000000 ) ;
#155078=CARTESIAN_POINT ( 'NONE',  ( 23.40000000000005542, 87.50449464844290048, -37.85861909827351468 ) ) ;
#155082=CARTESIAN_POINT ( 'NONE',  ( 23.40000000000005542, 64.35000000001120668, -3.123107484524795474 ) ) ;
#155092=EDGE_LOOP ( 'NONE', ( #139493, #110481, #70972, #216291 ) ) ;
#155111=CARTESIAN_POINT ( 'NONE',  ( 0.9000000000000554223, 63.75000000001118394, -10.02310748452479139 ) ) ;
#155158=CARTESIAN_POINT ( 'NONE',  ( -11.59999999999994458, 64.35000000001120668, -23.62310748452479103 ) ) ;
#155164=CARTESIAN_POINT ( 'NONE',  ( -21.04999999999994387, 83.80000000001119531, -37.18565239344504647 ) ) ;
#155215=DIRECTION ( 'NONE',  ( -1.000000000000000000, -0.000000000000000000, -0.000000000000000000 ) ) ;
#155246=PLANE ( 'NONE',  #133877 ) ;
#155278=CIRCLE ( 'NONE', #205099, 0.1000000000000028644 ) ;
#155325=DIRECTION ( 'NONE',  ( -0.000000000000000000, -0.000000000000000000, 1.000000000000000000 ) ) ;
#155331=CARTESIAN_POINT ( 'NONE',  ( -20.94999999999994600, 65.27857539272349641, -29.97167177764265844 ) ) ;
#155408=EDGE_CURVE ( 'NONE', #134698, #28383, #104698, .T. ) ;
#155413=ORIENTED_EDGE ( 'NONE', *, *, #147461, .T. ) ;
#155421=DIRECTION ( 'NONE',  ( 0.000000000000000000, 0.000000000000000000, -1.000000000000000000 ) ) ;
#155496=PLANE ( 'NONE',  #144554 ) ;
#155497=EDGE_LOOP ( 'NONE', ( #191474, #6179, #16063, #98865 ) ) ;
#155518=ORIENTED_EDGE ( 'NONE', *, *, #204047, .T. ) ;
#155523=DIRECTION ( 'NONE',  ( 0.000000000000000000, 0.000000000000000000, -1.000000000000000000 ) ) ;
#155605=DIRECTION ( 'NONE',  ( 0.000000000000000000, 0.000000000000000000, -1.000000000000000000 ) ) ;
#155625=AXIS2_PLACEMENT_3D ( 'NONE', #83104, #122281, #201804 ) ;
#155657=DIRECTION ( 'NONE',  ( 0.000000000000000000, 0.000000000000000000, 1.000000000000000000 ) ) ;
#155662=AXIS2_PLACEMENT_3D ( 'NONE', #221587, #2552, #143353 ) ;
#155664=ORIENTED_EDGE ( 'NONE', *, *, #93583, .T. ) ;
#155704=ORIENTED_EDGE ( 'NONE', *, *, #138522, .T. ) ;
#155742=EDGE_CURVE ( 'NONE', #131459, #297, #8939, .T. ) ;
#155750=EDGE_CURVE ( 'NONE', #18100, #97476, #96702, .T. ) ;
#155760=CARTESIAN_POINT ( 'NONE',  ( 21.15000000000005542, 82.64476912853859858, -26.37791261425322986 ) ) ;
#155886=DIRECTION ( 'NONE',  ( 0.000000000000000000, 0.000000000000000000, 1.000000000000000000 ) ) ;
#155888=LINE ( 'NONE', #17614, #140612 ) ;
#155931=DIRECTION ( 'NONE',  ( 0.000000000000000000, 0.000000000000000000, 1.000000000000000000 ) ) ;
#155949=CARTESIAN_POINT ( 'NONE',  ( 21.15000000000005187, 83.90000000001120384, -34.77310748452479316 ) ) ;
#155968=CYLINDRICAL_SURFACE ( 'NONE', #83841, 11.74999999999999645 ) ;
#155970=FACE_OUTER_BOUND ( 'NONE', #120510, .T. ) ;
#155977=CARTESIAN_POINT ( 'NONE',  ( 23.40000000000005542, 66.40137734081807253, -35.02137779515522453 ) ) ;
#155982=CARTESIAN_POINT ( 'NONE',  ( -21.14999999999994174, 83.98667523412385094, -34.76145429838185663 ) ) ;
#155990=DIRECTION ( 'NONE',  ( -1.000000000000000000, 0.000000000000000000, 0.000000000000000000 ) ) ;
#156070=ORIENTED_EDGE ( 'NONE', *, *, #234699, .T. ) ;
#156078=CIRCLE ( 'NONE', #130916, 0.09999999999999939493 ) ;
#156112=LINE ( 'NONE', #174413, #237567 ) ;
#156169=ORIENTED_EDGE ( 'NONE', *, *, #85563, .T. ) ;
#156212=FACE_OUTER_BOUND ( 'NONE', #136165, .T. ) ;
#156225=AXIS2_PLACEMENT_3D ( 'NONE', #71688, #11710, #168246 ) ;
#156262=DIRECTION ( 'NONE',  ( 0.000000000000000000, 0.000000000000000000, 1.000000000000000000 ) ) ;
#156318=CARTESIAN_POINT ( 'NONE',  ( -23.39999999999994529, 64.35000000001120668, -3.123107484524795474 ) ) ;
#156436=CARTESIAN_POINT ( 'NONE',  ( 5.900000000000059863, 64.25000000001119815, -25.92310748452479174 ) ) ;
#156504=DIRECTION ( 'NONE',  ( 0.000000000000000000, 0.000000000000000000, 1.000000000000000000 ) ) ;
#156519=EDGE_CURVE ( 'NONE', #213499, #158981, #72653, .T. ) ;
#156534=DIRECTION ( 'NONE',  ( 0.000000000000000000, 0.000000000000000000, -1.000000000000000000 ) ) ;
#156543=AXIS2_PLACEMENT_3D ( 'NONE', #9494, #186877, #32967 ) ;
#156576=EDGE_LOOP ( 'NONE', ( #177057, #171128, #22602, #4017 ) ) ;
#156589=ADVANCED_FACE ( 'NONE', ( #117373 ), #234749, .F. ) ;
#156629=CARTESIAN_POINT ( 'NONE',  ( 20.95000000000005258, 67.65000000001118963, -25.49719488170504533 ) ) ;
#156640=CARTESIAN_POINT ( 'NONE',  ( 21.15000000000005187, 79.88763423575340994, -7.282924647898262549 ) ) ;
#156649=ORIENTED_EDGE ( 'NONE', *, *, #42974, .T. ) ;
#156658=VECTOR ( 'NONE', #180987, 1000.000000000000000 ) ;
#156755=CARTESIAN_POINT ( 'NONE',  ( -21.04999999999994387, 77.83551161375991967, -47.52760213295649550 ) ) ;
#156766=AXIS2_PLACEMENT_3D ( 'NONE', #123306, #202829, #24218 ) ;
#156804=AXIS2_PLACEMENT_3D ( 'NONE', #19055, #214682, #36069 ) ;
#156846=AXIS2_PLACEMENT_3D ( 'NONE', #35528, #36809, #94163 ) ;
#156867=DIRECTION ( 'NONE',  ( 0.000000000000000000, 0.8741572761215442577, -0.4856429311786202851 ) ) ;
#156868=ORIENTED_EDGE ( 'NONE', *, *, #94855, .F. ) ;
#156880=CARTESIAN_POINT ( 'NONE',  ( -23.39999999999994529, 83.80000000001119531, -37.18565239344504647 ) ) ;
#156913=DIRECTION ( 'NONE',  ( -1.000000000000000000, 0.000000000000000000, 0.000000000000000000 ) ) ;
#156936=CARTESIAN_POINT ( 'NONE',  ( -40.23850191057533010, 64.35000000001119247, -6.123107484524794586 ) ) ;
#156959=AXIS2_PLACEMENT_3D ( 'NONE', #179079, #216876, #117786 ) ;
#157017=CIRCLE ( 'NONE', #44581, 0.1000000000000045852 ) ;
#157087=EDGE_CURVE ( 'NONE', #23181, #34352, #19237, .T. ) ;
#157095=ORIENTED_EDGE ( 'NONE', *, *, #1673, .T. ) ;
#157116=FACE_OUTER_BOUND ( 'NONE', #56979, .T. ) ;
#157124=EDGE_CURVE ( 'NONE', #123360, #1569, #256501, .T. ) ;
#157198=ORIENTED_EDGE ( 'NONE', *, *, #55192, .T. ) ;
#157260=DIRECTION ( 'NONE',  ( 0.000000000000000000, 0.000000000000000000, -1.000000000000000000 ) ) ;
#157265=ORIENTED_EDGE ( 'NONE', *, *, #137954, .T. ) ;
#157293=EDGE_CURVE ( 'NONE', #126736, #33512, #7370, .T. ) ;
#157325=AXIS2_PLACEMENT_3D ( 'NONE', #128110, #188081, #107252 ) ;
#157351=ORIENTED_EDGE ( 'NONE', *, *, #215977, .T. ) ;
#157382=EDGE_CURVE ( 'NONE', #149012, #134658, #164591, .T. ) ;
#157392=CIRCLE ( 'NONE', #111573, 2.599999999999998312 ) ;
#157393=ORIENTED_EDGE ( 'NONE', *, *, #78514, .T. ) ;
#157402=EDGE_LOOP ( 'NONE', ( #223326, #21451, #233596, #191419 ) ) ;
#157477=EDGE_CURVE ( 'NONE', #192885, #34352, #93644, .T. ) ;
#157512=CARTESIAN_POINT ( 'NONE',  ( -20.94999999999994600, 65.15000000001120384, -3.023107484524792277 ) ) ;
#157580=AXIS2_PLACEMENT_3D ( 'NONE', #87714, #246797, #29091 ) ;
#157591=EDGE_LOOP ( 'NONE', ( #93303, #60807, #14536, #36484 ) ) ;
#157617=CARTESIAN_POINT ( 'NONE',  ( -6.099999999999939249, 64.25000000001119815, -51.02310748452479316 ) ) ;
#157623=AXIS2_PLACEMENT_3D ( 'NONE', #9552, #188203, #52526 ) ;
#157626=TOROIDAL_SURFACE ( 'NONE', #53534, 11.65000000000000036, 0.1000000000000000056 ) ;
#157638=ORIENTED_EDGE ( 'NONE', *, *, #215345, .F. ) ;
#157667=CARTESIAN_POINT ( 'NONE',  ( 23.40000000000005542, 83.80000000001119531, -37.18565239344504647 ) ) ;
#157673=EDGE_LOOP ( 'NONE', ( #113870, #15297, #39118, #38981 ) ) ;
#157684=DIRECTION ( 'NONE',  ( 0.000000000000000000, -1.000000000000000000, 0.000000000000000000 ) ) ;
#157839=EDGE_CURVE ( 'NONE', #205114, #135372, #56017, .T. ) ;
#157885=ORIENTED_EDGE ( 'NONE', *, *, #24211, .T. ) ;
#157988=LINE ( 'NONE', #75839, #31542 ) ;
#158079=EDGE_CURVE ( 'NONE', #243985, #34352, #206260, .T. ) ;
#158090=CARTESIAN_POINT ( 'NONE',  ( 23.40000000000005542, 76.00000000001119815, -3.123107484524795474 ) ) ;
#158105=EDGE_LOOP ( 'NONE', ( #64444, #124249, #43739, #75700 ) ) ;
#158142=ORIENTED_EDGE ( 'NONE', *, *, #106482, .F. ) ;
#158149=CYLINDRICAL_SURFACE ( 'NONE', #146860, 0.1000000000000021844 ) ;
#158253=EDGE_LOOP ( 'NONE', ( #44697, #164054, #30200, #65444 ) ) ;
#158262=CIRCLE ( 'NONE', #4096, 0.09999999999999939493 ) ;
#158362=AXIS2_PLACEMENT_3D ( 'NONE', #204560, #140737, #5048 ) ;
#158408=DIRECTION ( 'NONE',  ( 0.000000000000000000, 0.000000000000000000, -1.000000000000000000 ) ) ;
#158424=CYLINDRICAL_SURFACE ( 'NONE', #9211, 11.74999999999999645 ) ;
#158438=AXIS2_PLACEMENT_3D ( 'NONE', #49908, #229835, #167320 ) ;
#158441=DIRECTION ( 'NONE',  ( 1.000000000000000000, 0.000000000000000000, 0.000000000000000000 ) ) ;
#158548=EDGE_CURVE ( 'NONE', #201062, #223504, #164917, .T. ) ;
#158597=CARTESIAN_POINT ( 'NONE',  ( -5.899999999999938183, 64.65000000001120384, -25.92310748452479174 ) ) ;
#158631=EDGE_LOOP ( 'NONE', ( #74714, #110203, #200250, #133723 ) ) ;
#158675=ORIENTED_EDGE ( 'NONE', *, *, #89228, .F. ) ;
#158724=ORIENTED_EDGE ( 'NONE', *, *, #44290, .F. ) ;
#158779=AXIS2_PLACEMENT_3D ( 'NONE', #56044, #191769, #170941 ) ;
#158807=DIRECTION ( 'NONE',  ( 0.000000000000000000, 0.000000000000000000, 1.000000000000000000 ) ) ;
#158856=AXIS2_PLACEMENT_3D ( 'NONE', #253833, #255073, #17787 ) ;
#158921=EDGE_LOOP ( 'NONE', ( #40167, #47221, #238541, #143382 ) ) ;
#158929=EDGE_LOOP ( 'NONE', ( #202267, #205002, #44254, #256813 ) ) ;
#158932=DIRECTION ( 'NONE',  ( 0.000000000000000000, -0.1480365673253065117, 0.9889818879709273425 ) ) ;
#158946=CARTESIAN_POINT ( 'NONE',  ( 21.15000000000005187, 64.25000000001119815, -3.123107484524795474 ) ) ;
#158952=ADVANCED_FACE ( 'NONE', ( #257608 ), #195164, .T. ) ;
#158973=CARTESIAN_POINT ( 'NONE',  ( -13.39999999999994351, 63.75000000001119815, -21.02310748452479316 ) ) ;
#158977=DIRECTION ( 'NONE',  ( 0.000000000000000000, 0.000000000000000000, 1.000000000000000000 ) ) ;
#158981=VERTEX_POINT ( 'NONE', #55580 ) ;
#158985=AXIS2_PLACEMENT_3D ( 'NONE', #222844, #84574, #142028 ) ;
#158993=DIRECTION ( 'NONE',  ( 1.000000000000000000, -0.000000000000000000, -0.000000000000000000 ) ) ;
#159048=ORIENTED_EDGE ( 'NONE', *, *, #248568, .T. ) ;
#159095=ADVANCED_FACE ( 'NONE', ( #745 ), #80281, .T. ) ;
#159113=CYLINDRICAL_SURFACE ( 'NONE', #89441, 0.09999999999999982514 ) ;
#159135=PLANE ( 'NONE',  #230641 ) ;
#159149=ORIENTED_EDGE ( 'NONE', *, *, #242490, .F. ) ;
#159157=CARTESIAN_POINT ( 'NONE',  ( 20.95000000000005258, 66.25000000001119815, -4.623107484524796362 ) ) ;
#159162=ORIENTED_EDGE ( 'NONE', *, *, #19825, .T. ) ;
#159167=CARTESIAN_POINT ( 'NONE',  ( -40.23850191057533010, 66.25000000001114131, -51.02310748452476474 ) ) ;
#159184=EDGE_CURVE ( 'NONE', #6953, #252227, #206801, .T. ) ;
#159200=TOROIDAL_SURFACE ( 'NONE', #46740, 2.699999999999999734, 0.1000000000000000056 ) ;
#159255=DIRECTION ( 'NONE',  ( 0.000000000000000000, 0.000000000000000000, -1.000000000000000000 ) ) ;
#159303=DIRECTION ( 'NONE',  ( 0.000000000000000000, -0.9910827722268055195, 0.1332476588733540468 ) ) ;
#159322=ADVANCED_FACE ( 'NONE', ( #3026 ), #211082, .F. ) ;
#159414=DIRECTION ( 'NONE',  ( 1.000000000000000000, -0.000000000000000000, -0.000000000000000000 ) ) ;
#159415=EDGE_CURVE ( 'NONE', #43374, #231379, #103403, .T. ) ;
#159419=EDGE_LOOP ( 'NONE', ( #155664, #60247 ) ) ;
#159473=ADVANCED_FACE ( 'NONE', ( #29073 ), #14315, .T. ) ;
#159528=CARTESIAN_POINT ( 'NONE',  ( 21.15000000000005542, 77.73640333653723644, -47.54092689884382850 ) ) ;
#159552=VECTOR ( 'NONE', #189224, 1000.000000000000000 ) ;
#159555=EDGE_CURVE ( 'NONE', #109039, #224041, #90253, .T. ) ;
#159645=CIRCLE ( 'NONE', #47189, 11.65000000000000036 ) ;
#159716=CARTESIAN_POINT ( 'NONE',  ( -23.39999999999994529, 77.16254490893143725, -44.02310748452479316 ) ) ;
#159750=ADVANCED_FACE ( 'NONE', ( #7555 ), #36516, .T. ) ;
#159784=TOROIDAL_SURFACE ( 'NONE', #43081, 2.699999999999999734, 0.1000000000000000056 ) ;
#159815=ORIENTED_EDGE ( 'NONE', *, *, #140323, .F. ) ;
#159820=AXIS2_PLACEMENT_3D ( 'NONE', #158973, #19438, #16881 ) ;
#159853=LINE ( 'NONE', #20346, #223392 ) ;
#159916=ADVANCED_FACE ( 'NONE', ( #212191 ), #47953, .T. ) ;
#159972=AXIS2_PLACEMENT_3D ( 'NONE', #211889, #54074, #250977 ) ;
#160007=ORIENTED_EDGE ( 'NONE', *, *, #14679, .F. ) ;
#160010=CARTESIAN_POINT ( 'NONE',  ( -23.49999999999994316, 77.83551161375991967, -47.52760213295649550 ) ) ;
#160016=CARTESIAN_POINT ( 'NONE',  ( 21.05000000000005400, 67.65000000001118963, -25.49719488170504533 ) ) ;
#160063=DIRECTION ( 'NONE',  ( 0.000000000000000000, -0.000000000000000000, 1.000000000000000000 ) ) ;
#160085=FACE_OUTER_BOUND ( 'NONE', #153436, .T. ) ;
#160109=DIRECTION ( 'NONE',  ( -1.000000000000000000, 0.000000000000000000, -0.000000000000000000 ) ) ;
#160188=FACE_OUTER_BOUND ( 'NONE', #32543, .T. ) ;
#160256=ORIENTED_EDGE ( 'NONE', *, *, #144705, .T. ) ;
#160304=FACE_OUTER_BOUND ( 'NONE', #207347, .T. ) ;
#160328=AXIS2_PLACEMENT_3D ( 'NONE', #7804, #28690, #224261 ) ;
#160355=EDGE_LOOP ( 'NONE', ( #48494, #54146, #174742, #97428 ) ) ;
#160383=ORIENTED_EDGE ( 'NONE', *, *, #242263, .T. ) ;
#160443=DIRECTION ( 'NONE',  ( 0.000000000000000000, -1.000000000000000000, 0.000000000000000000 ) ) ;
#160474=TOROIDAL_SURFACE ( 'NONE', #185390, 4.041421356237307805, 0.1000000000000000056 ) ;
#160503=ORIENTED_EDGE ( 'NONE', *, *, #246345, .T. ) ;
#160513=DIRECTION ( 'NONE',  ( 0.000000000000000000, -1.000000000000000000, 0.000000000000000000 ) ) ;
#160531=ORIENTED_EDGE ( 'NONE', *, *, #104142, .T. ) ;
#160537=ORIENTED_EDGE ( 'NONE', *, *, #67883, .T. ) ;
#160549=VERTEX_POINT ( 'NONE', #228570 ) ;
#160556=ORIENTED_EDGE ( 'NONE', *, *, #151999, .F. ) ;
#160566=CARTESIAN_POINT ( 'NONE',  ( -23.39999999999994529, 74.83745509109094485, -44.02310748452479316 ) ) ;
#160573=CIRCLE ( 'NONE', #189759, 0.1999999999999987899 ) ;
#160684=DIRECTION ( 'NONE',  ( 0.000000000000000000, 0.000000000000000000, -1.000000000000000000 ) ) ;
#160718=CARTESIAN_POINT ( 'NONE',  ( -13.39999999999994351, 66.35000000001119247, -18.42310748452479174 ) ) ;
#160760=ORIENTED_EDGE ( 'NONE', *, *, #68350, .F. ) ;
#160949=EDGE_CURVE ( 'NONE', #215142, #207750, #224455, .T. ) ;
#160991=CARTESIAN_POINT ( 'NONE',  ( -13.39999999999994529, 67.65000000001118963, -21.02310748452479316 ) ) ;
#160999=ORIENTED_EDGE ( 'NONE', *, *, #153062, .T. ) ;
#161036=EDGE_LOOP ( 'NONE', ( #115050, #128674, #52515, #31622 ) ) ;
#161087=ORIENTED_EDGE ( 'NONE', *, *, #75636, .T. ) ;
#161110=FACE_OUTER_BOUND ( 'NONE', #234116, .T. ) ;
#161116=VERTEX_POINT ( 'NONE', #205481 ) ;
#161153=CARTESIAN_POINT ( 'NONE',  ( 5.900000000000060751, 64.65000000001120384, -22.12310748452479103 ) ) ;
#161172=ORIENTED_EDGE ( 'NONE', *, *, #52973, .T. ) ;
#161187=ORIENTED_EDGE ( 'NONE', *, *, #203593, .F. ) ;
#161245=CARTESIAN_POINT ( 'NONE',  ( 11.60000000000006004, 64.25000000001119815, -21.02310748452479316 ) ) ;
#161298=EDGE_LOOP ( 'NONE', ( #173997, #219032, #103014, #246117 ) ) ;
#161306=VECTOR ( 'NONE', #7893, 1000.000000000000000 ) ;
#161318=DIRECTION ( 'NONE',  ( 1.000000000000000000, -0.000000000000000000, -0.000000000000000000 ) ) ;
#161411=CIRCLE ( 'NONE', #28143, 0.09999999999999939493 ) ;
#161428=CARTESIAN_POINT ( 'NONE',  ( -21.14999999999994174, 64.25000000001119815, -36.02310748452479316 ) ) ;
#161436=CIRCLE ( 'NONE', #132197, 4.041421356237314022 ) ;
#161445=CARTESIAN_POINT ( 'NONE',  ( 21.05000000000005400, 67.85000000001119247, -25.49719488170504533 ) ) ;
#161470=CARTESIAN_POINT ( 'NONE',  ( 21.05000000000005400, 74.63923853664559260, -43.99645795275012006 ) ) ;
#161503=EDGE_CURVE ( 'NONE', #172317, #210574, #197471, .T. ) ;
#161533=EDGE_CURVE ( 'NONE', #148669, #146220, #3110, .T. ) ;
#161561=ORIENTED_EDGE ( 'NONE', *, *, #226448, .F. ) ;
#161607=FACE_OUTER_BOUND ( 'NONE', #203495, .T. ) ;
#161655=DIRECTION ( 'NONE',  ( -1.000000000000000000, -0.000000000000000000, -0.000000000000000000 ) ) ;
#161700=EDGE_CURVE ( 'NONE', #132923, #145505, #5067, .T. ) ;
#161732=VERTEX_POINT ( 'NONE', #104184 ) ;
#161819=DIRECTION ( 'NONE',  ( 1.000000000000000000, 0.000000000000000000, 0.000000000000000000 ) ) ;
#161846=CARTESIAN_POINT ( 'NONE',  ( -23.49999999999994316, 76.00000000001119815, -36.02310748452479316 ) ) ;
#161937=ORIENTED_EDGE ( 'NONE', *, *, #251511, .T. ) ;
#161988=DIRECTION ( 'NONE',  ( 0.000000000000000000, 0.000000000000000000, 1.000000000000000000 ) ) ;
#162047=DIRECTION ( 'NONE',  ( -1.000000000000000000, 0.000000000000000000, -0.000000000000000000 ) ) ;
#162066=ADVANCED_FACE ( 'NONE', ( #184702 ), #245978, .T. ) ;
#162331=EDGE_CURVE ( 'NONE', #135761, #59396, #1588, .T. ) ;
#162333=EDGE_CURVE ( 'NONE', #9389, #30313, #95865, .T. ) ;
#162522=DIRECTION ( 'NONE',  ( -1.000000000000000000, 0.000000000000000000, 0.000000000000000000 ) ) ;
#162562=DIRECTION ( 'NONE',  ( 1.000000000000000000, 0.000000000000000000, 0.000000000000000000 ) ) ;
#162573=TOROIDAL_SURFACE ( 'NONE', #50107, 4.150000000000000355, 0.1000000000000000056 ) ;
#162586=FACE_OUTER_BOUND ( 'NONE', #4303, .T. ) ;
#162686=CARTESIAN_POINT ( 'NONE',  ( -21.04999999999994387, 76.00000000001119815, -36.02310748452479316 ) ) ;
#162694=AXIS2_PLACEMENT_3D ( 'NONE', #225363, #84535, #183699 ) ;
#162772=PLANE ( 'NONE',  #181165 ) ;
#162810=EDGE_CURVE ( 'NONE', #3259, #73651, #24929, .T. ) ;
#162901=CARTESIAN_POINT ( 'NONE',  ( -23.39999999999994529, 74.16448838626247664, -47.62760213295649692 ) ) ;
#162937=AXIS2_PLACEMENT_3D ( 'NONE', #37130, #134890, #35841 ) ;
#162968=ORIENTED_EDGE ( 'NONE', *, *, #191615, .T. ) ;
#163005=LINE ( 'NONE', #122592, #10157 ) ;
#163016=EDGE_CURVE ( 'NONE', #197879, #167673, #14155, .T. ) ;
#163051=EDGE_CURVE ( 'NONE', #121523, #106796, #250178, .T. ) ;
#163074=AXIS2_PLACEMENT_3D ( 'NONE', #8652, #92033, #171613 ) ;
#163077=CARTESIAN_POINT ( 'NONE',  ( -13.39999999999994529, 64.25000000001119815, -18.32310748452479388 ) ) ;
#163093=EDGE_LOOP ( 'NONE', ( #63614, #120775, #18837, #200003 ) ) ;
#163219=VECTOR ( 'NONE', #204320, 1000.000000000000114 ) ;
#163238=CARTESIAN_POINT ( 'NONE',  ( -23.49999999999994316, 76.00000000001119815, -36.02310748452479316 ) ) ;
#163268=AXIS2_PLACEMENT_3D ( 'NONE', #219235, #141012, #101837 ) ;
#163293=LINE ( 'NONE', #139849, #33719 ) ;
#163314=ORIENTED_EDGE ( 'NONE', *, *, #239328, .F. ) ;
#163316=DIRECTION ( 'NONE',  ( -6.420062716055394467E-16, 0.1480365673253023484, -0.9889818879709282307 ) ) ;
#163342=CARTESIAN_POINT ( 'NONE',  ( 23.40000000000005187, 77.75000000001119815, -47.64205752314703801 ) ) ;
#163343=ORIENTED_EDGE ( 'NONE', *, *, #213756, .F. ) ;
#163358=ORIENTED_EDGE ( 'NONE', *, *, #159415, .T. ) ;
#163372=ADVANCED_FACE ( 'NONE', ( #8683 ), #20832, .F. ) ;
#163416=DIRECTION ( 'NONE',  ( 0.000000000000000000, 0.000000000000000000, -1.000000000000000000 ) ) ;
#163421=VECTOR ( 'NONE', #62195, 1000.000000000000000 ) ;
#163473=ORIENTED_EDGE ( 'NONE', *, *, #86271, .T. ) ;
#163520=DIRECTION ( 'NONE',  ( 1.000000000000000000, -0.000000000000000000, -0.000000000000000000 ) ) ;
#163535=ADVANCED_FACE ( 'NONE', ( #193741 ), #77610, .F. ) ;
#163556=AXIS2_PLACEMENT_3D ( 'NONE', #88644, #165664, #27461 ) ;
#163630=FACE_OUTER_BOUND ( 'NONE', #231549, .T. ) ;
#163639=DIRECTION ( 'NONE',  ( -0.000000000000000000, 1.000000000000000000, -0.000000000000000000 ) ) ;
#163713=DIRECTION ( 'NONE',  ( -1.000000000000000000, 0.000000000000000000, 0.000000000000000000 ) ) ;
#163790=ORIENTED_EDGE ( 'NONE', *, *, #255989, .F. ) ;
#163816=ORIENTED_EDGE ( 'NONE', *, *, #38735, .F. ) ;
#163819=ORIENTED_EDGE ( 'NONE', *, *, #215977, .F. ) ;
#163857=FACE_BOUND ( 'NONE', #29406, .T. ) ;
#163934=CARTESIAN_POINT ( 'NONE',  ( -21.14999999999994174, 76.00000000001119815, -3.123107484524795474 ) ) ;
#163938=EDGE_CURVE ( 'NONE', #90057, #178217, #191897, .T. ) ;
#163971=ORIENTED_EDGE ( 'NONE', *, *, #195472, .F. ) ;
#164028=AXIS2_PLACEMENT_3D ( 'NONE', #179561, #180832, #101231 ) ;
#164054=ORIENTED_EDGE ( 'NONE', *, *, #225314, .T. ) ;
#164062=DIRECTION ( 'NONE',  ( 0.000000000000000000, 0.000000000000000000, -1.000000000000000000 ) ) ;
#164157=DIRECTION ( 'NONE',  ( -1.000000000000000000, 0.000000000000000000, 0.000000000000000000 ) ) ;
#164169=CARTESIAN_POINT ( 'NONE',  ( -40.23850191057533010, 65.35000000001120668, -4.523107484524794053 ) ) ;
#164203=EDGE_CURVE ( 'NONE', #249539, #207750, #37950, .T. ) ;
#164248=CARTESIAN_POINT ( 'NONE',  ( 21.05000000000005400, 77.36076146337680370, -43.99645795275012006 ) ) ;
#164287=( LENGTH_UNIT ( ) NAMED_UNIT ( * ) SI_UNIT ( .MILLI., .METRE. ) );
#164360=LINE ( 'NONE', #246452, #186031 ) ;
#164362=ORIENTED_EDGE ( 'NONE', *, *, #160949, .F. ) ;
#164467=AXIS2_PLACEMENT_3D ( 'NONE', #67891, #249118, #45757 ) ;
#164529=ADVANCED_FACE ( 'NONE', ( #218458 ), #155968, .T. ) ;
#164533=AXIS2_PLACEMENT_3D ( 'NONE', #98590, #101148, #119496 ) ;
#164536=DIRECTION ( 'NONE',  ( 0.000000000000000000, 1.000000000000000000, 0.000000000000000000 ) ) ;
#164576=DIRECTION ( 'NONE',  ( 0.000000000000000000, 0.000000000000000000, -1.000000000000000000 ) ) ;
#164591=CIRCLE ( 'NONE', #97903, 0.09999999999999939493 ) ;
#164596=ORIENTED_EDGE ( 'NONE', *, *, #240703, .F. ) ;
#164619=EDGE_CURVE ( 'NONE', #123853, #191279, #187957, .T. ) ;
#164682=CIRCLE ( 'NONE', #177183, 3.970710678118653636 ) ;
#164693=FACE_OUTER_BOUND ( 'NONE', #84895, .T. ) ;
#164695=DIRECTION ( 'NONE',  ( 0.000000000000000000, 0.000000000000000000, -1.000000000000000000 ) ) ;
#164724=EDGE_CURVE ( 'NONE', #74170, #201487, #190935, .T. ) ;
#164757=EDGE_LOOP ( 'NONE', ( #235245, #24135, #96973 ) ) ;
#164789=EDGE_CURVE ( 'NONE', #223504, #170630, #144899, .T. ) ;
#164891=ORIENTED_EDGE ( 'NONE', *, *, #120961, .T. ) ;
#164917=CIRCLE ( 'NONE', #73381, 0.1000000000000028644 ) ;
#164929=ORIENTED_EDGE ( 'NONE', *, *, #193481, .T. ) ;
#164942=CARTESIAN_POINT ( 'NONE',  ( 0.9000000000000547562, 67.75000000001118394, -10.02310748452479139 ) ) ;
#164981=DIRECTION ( 'NONE',  ( 0.000000000000000000, 0.000000000000000000, 1.000000000000000000 ) ) ;
#164982=CARTESIAN_POINT ( 'NONE',  ( -23.49999999999994316, 78.47315729244128590, -52.27034697567518862 ) ) ;
#164989=EDGE_CURVE ( 'NONE', #200341, #123360, #113494, .T. ) ;
#165013=EDGE_LOOP ( 'NONE', ( #114608, #24543, #113365, #228765 ) ) ;
#165068=DIRECTION ( 'NONE',  ( 0.000000000000000000, 0.9889818879709272315, 0.1480365673253073999 ) ) ;
#165097=DIRECTION ( 'NONE',  ( 0.000000000000000000, 0.9889818879709274535, 0.1480365673253065395 ) ) ;
#165228=DIRECTION ( 'NONE',  ( 0.000000000000000000, 0.000000000000000000, 1.000000000000000000 ) ) ;
#165241=AXIS2_PLACEMENT_3D ( 'NONE', #49769, #172340, #129310 ) ;
#165248=CARTESIAN_POINT ( 'NONE',  ( -13.39999999999994529, 64.35000000001120668, -21.02310748452479316 ) ) ;
#165269=DIRECTION ( 'NONE',  ( 0.000000000000000000, 0.000000000000000000, -1.000000000000000000 ) ) ;
#165290=EDGE_LOOP ( 'NONE', ( #13705, #136884, #201661, #140087 ) ) ;
#165357=ORIENTED_EDGE ( 'NONE', *, *, #146318, .F. ) ;
#165369=CARTESIAN_POINT ( 'NONE',  ( -23.49999999999994316, 64.35000000001120668, -51.02310748452479316 ) ) ;
#165372=AXIS2_PLACEMENT_3D ( 'NONE', #134792, #223323, #81237 ) ;
#165404=EDGE_CURVE ( 'NONE', #211140, #186900, #256961, .T. ) ;
#165416=PLANE ( 'NONE',  #223760 ) ;
#165429=CIRCLE ( 'NONE', #57046, 0.09999999999999939493 ) ;
#165438=CARTESIAN_POINT ( 'NONE',  ( -11.59999999999994458, 63.75000000001119815, -21.02310748452479316 ) ) ;
#165439=DIRECTION ( 'NONE',  ( 1.000000000000000000, -0.000000000000000000, -0.000000000000000000 ) ) ;
#165446=VECTOR ( 'NONE', #111241, 1000.000000000000000 ) ;
#165490=VERTEX_POINT ( 'NONE', #229445 ) ;
#165492=DIRECTION ( 'NONE',  ( 1.000000000000000000, 0.000000000000000000, 0.000000000000000000 ) ) ;
#165503=ORIENTED_EDGE ( 'NONE', *, *, #43457, .F. ) ;
#165509=CIRCLE ( 'NONE', #82254, 0.1999999999999987899 ) ;
#165563=DIRECTION ( 'NONE',  ( 0.000000000000000000, 0.000000000000000000, 1.000000000000000000 ) ) ;
#165597=VECTOR ( 'NONE', #122864, 1000.000000000000000 ) ;
#165610=AXIS2_PLACEMENT_3D ( 'NONE', #223801, #242083, #6034 ) ;
#165615=ORIENTED_EDGE ( 'NONE', *, *, #42097, .F. ) ;
#165616=ORIENTED_EDGE ( 'NONE', *, *, #217147, .T. ) ;
#165646=CARTESIAN_POINT ( 'NONE',  ( -13.39999999999994529, 63.75000000001119815, -21.02310748452479316 ) ) ;
#165652=DIRECTION ( 'NONE',  ( -1.000000000000000000, -0.000000000000000000, -0.000000000000000000 ) ) ;
#165664=DIRECTION ( 'NONE',  ( 1.000000000000000000, -0.000000000000000000, -0.000000000000000000 ) ) ;
#165677=CARTESIAN_POINT ( 'NONE',  ( -23.49999999999994316, 87.50449464844290048, -37.85861909827351468 ) ) ;
#165735=ORIENTED_EDGE ( 'NONE', *, *, #143369, .F. ) ;
#165740=DIRECTION ( 'NONE',  ( 1.000000000000000000, 0.000000000000000000, 0.000000000000000000 ) ) ;
#165749=ORIENTED_EDGE ( 'NONE', *, *, #142869, .T. ) ;
#165756=CIRCLE ( 'NONE', #182311, 4.150000000000001243 ) ;
#165771=DIRECTION ( 'NONE',  ( 1.000000000000000000, 0.000000000000000000, 0.000000000000000000 ) ) ;
#165784=ADVANCED_FACE ( 'NONE', ( #42795 ), #189686, .T. ) ;
#165834=CARTESIAN_POINT ( 'NONE',  ( -23.49999999999994316, 74.83745509109094485, -43.92310748452479885 ) ) ;
#165837=DIRECTION ( 'NONE',  ( 0.000000000000000000, -0.7071067811865472397, -0.7071067811865479058 ) ) ;
#165953=DIRECTION ( 'NONE',  ( 0.000000000000000000, 0.000000000000000000, 1.000000000000000000 ) ) ;
#165986=CIRCLE ( 'NONE', #36988, 0.1000000000000028644 ) ;
#166017=CARTESIAN_POINT ( 'NONE',  ( -23.49999999999994316, 76.00000000001119815, -40.07310748452479032 ) ) ;
#166224=EDGE_CURVE ( 'NONE', #11972, #58156, #6881, .T. ) ;
#166226=AXIS2_PLACEMENT_3D ( 'NONE', #33246, #110166, #31951 ) ;
#166236=CARTESIAN_POINT ( 'NONE',  ( 21.05000000000005400, 87.75000000001119815, -3.123107484524795474 ) ) ;
#166272=DIRECTION ( 'NONE',  ( 1.000000000000000000, 0.000000000000000000, 0.000000000000000000 ) ) ;
#166340=CARTESIAN_POINT ( 'NONE',  ( -11.59999999999994458, 67.72071067812984779, -17.05239680640613642 ) ) ;
#166363=DIRECTION ( 'NONE',  ( 0.000000000000000000, 0.000000000000000000, 1.000000000000000000 ) ) ;
#166421=CIRCLE ( 'NONE', #83135, 4.150000000000001243 ) ;
#166555=VERTEX_POINT ( 'NONE', #240069 ) ;
#166562=CYLINDRICAL_SURFACE ( 'NONE', #243740, 0.09999999999999939493 ) ;
#166577=AXIS2_PLACEMENT_3D ( 'NONE', #72525, #92060, #171645 ) ;
#166634=ORIENTED_EDGE ( 'NONE', *, *, #244498, .F. ) ;
#166653=ORIENTED_EDGE ( 'NONE', *, *, #81158, .F. ) ;
#166697=CARTESIAN_POINT ( 'NONE',  ( 21.05000000000005400, 83.97335046823651794, -37.38386894789040582 ) ) ;
#166785=DIRECTION ( 'NONE',  ( 0.000000000000000000, 0.000000000000000000, 1.000000000000000000 ) ) ;
#166853=CARTESIAN_POINT ( 'NONE',  ( -21.04999999999994387, 83.97335046823651794, -37.38386894789040582 ) ) ;
#166870=CIRCLE ( 'NONE', #229, 0.1000000000000028644 ) ;
#166948=ORIENTED_EDGE ( 'NONE', *, *, #64638, .F. ) ;
#166955=DIRECTION ( 'NONE',  ( -0.000000000000000000, 1.000000000000000000, -0.000000000000000000 ) ) ;
#167075=CARTESIAN_POINT ( 'NONE',  ( -21.14999999999994174, 87.50449464844290048, -37.85861909827351468 ) ) ;
#167079=DIRECTION ( 'NONE',  ( 0.000000000000000000, 0.000000000000000000, 1.000000000000000000 ) ) ;
#167097=FACE_OUTER_BOUND ( 'NONE', #208447, .T. ) ;
#167131=AXIS2_PLACEMENT_3D ( 'NONE', #218327, #200077, #61854 ) ;
#167150=DIRECTION ( 'NONE',  ( 1.000000000000000000, 0.000000000000000000, 0.000000000000000000 ) ) ;
#167159=DIRECTION ( 'NONE',  ( -1.000000000000000000, 0.000000000000000000, 0.000000000000000000 ) ) ;
#167177=DIRECTION ( 'NONE',  ( 0.000000000000000000, 0.000000000000000000, -1.000000000000000000 ) ) ;
#167211=CIRCLE ( 'NONE', #21452, 0.1000000000000002554 ) ;
#167214=EDGE_CURVE ( 'NONE', #24890, #133820, #97515, .T. ) ;
#167224=VERTEX_POINT ( 'NONE', #210897 ) ;
#167243=CARTESIAN_POINT ( 'NONE',  ( 5.900000000000061640, 64.75000000001119815, -22.12310748452479103 ) ) ;
#167248=ORIENTED_EDGE ( 'NONE', *, *, #197824, .T. ) ;
#167289=DIRECTION ( 'NONE',  ( -1.000000000000000000, 0.000000000000000000, 0.000000000000000000 ) ) ;
#167311=AXIS2_PLACEMENT_3D ( 'NONE', #113470, #15695, #76908 ) ;
#167320=DIRECTION ( 'NONE',  ( 0.000000000000000000, 0.000000000000000000, -1.000000000000000000 ) ) ;
#167351=CIRCLE ( 'NONE', #242141, 0.09999999999999939493 ) ;
#167395=DIRECTION ( 'NONE',  ( 1.000000000000000000, 0.000000000000000000, 0.000000000000000000 ) ) ;
#167400=DIRECTION ( 'NONE',  ( 0.000000000000000000, 0.000000000000000000, 1.000000000000000000 ) ) ;
#167427=EDGE_CURVE ( 'NONE', #26051, #5207, #155278, .T. ) ;
#167443=EDGE_LOOP ( 'NONE', ( #23192, #255245, #54774, #5376 ) ) ;
#167446=EDGE_CURVE ( 'NONE', #74847, #169204, #127203, .T. ) ;
#167470=ADVANCED_FACE ( 'NONE', ( #102463 ), #183328, .T. ) ;
#167586=CARTESIAN_POINT ( 'NONE',  ( 23.40000000000004476, 84.00000000001119815, -34.86056257560453986 ) ) ;
#167590=CIRCLE ( 'NONE', #55111, 0.1999999999999987899 ) ;
#167612=CARTESIAN_POINT ( 'NONE',  ( -23.39999999999994529, 79.88763423575340994, -7.282924647898262549 ) ) ;
#167673=VERTEX_POINT ( 'NONE', #39368 ) ;
#167743=DIRECTION ( 'NONE',  ( -0.000000000000000000, 0.8164390028469705740, -0.5774316882803059992 ) ) ;
#167856=ORIENTED_EDGE ( 'NONE', *, *, #78727, .T. ) ;
#167876=ADVANCED_FACE ( 'NONE', ( #229540 ), #31368, .F. ) ;
#167916=ADVANCED_FACE ( 'NONE', ( #234666 ), #79825, .T. ) ;
#167941=VERTEX_POINT ( 'NONE', #155164 ) ;
#168024=LINE ( 'NONE', #231820, #229186 ) ;
#168094=DIRECTION ( 'NONE',  ( -1.000000000000000000, 0.000000000000000000, 0.000000000000000000 ) ) ;
#168099=FACE_OUTER_BOUND ( 'NONE', #216809, .T. ) ;
#168166=EDGE_CURVE ( 'NONE', #230635, #113629, #125802, .T. ) ;
#168187=AXIS2_PLACEMENT_3D ( 'NONE', #36128, #17812, #191365 ) ;
#168242=AXIS2_PLACEMENT_3D ( 'NONE', #25835, #46652, #110490 ) ;
#168246=DIRECTION ( 'NONE',  ( 1.000000000000000000, 0.000000000000000000, 0.000000000000000000 ) ) ;
#168284=ORIENTED_EDGE ( 'NONE', *, *, #169667, .T. ) ;
#168294=EDGE_CURVE ( 'NONE', #210105, #209133, #192453, .T. ) ;
#168296=VERTEX_POINT ( 'NONE', #48006 ) ;
#168304=DIRECTION ( 'NONE',  ( 0.000000000000000000, 0.000000000000000000, -1.000000000000000000 ) ) ;
#168353=ORIENTED_EDGE ( 'NONE', *, *, #42886, .T. ) ;
#168388=EDGE_CURVE ( 'NONE', #216036, #61669, #150757, .T. ) ;
#168389=DIRECTION ( 'NONE',  ( -1.000000000000000000, -0.000000000000000000, -0.000000000000000000 ) ) ;
#168396=CARTESIAN_POINT ( 'NONE',  ( -21.14999999999994174, 76.00000000001119815, -36.02310748452479316 ) ) ;
#168431=DIRECTION ( 'NONE',  ( 0.000000000000000000, -0.1480365673253065117, 0.9889818879709273425 ) ) ;
#168478=EDGE_CURVE ( 'NONE', #68170, #144016, #242527, .T. ) ;
#168503=DIRECTION ( 'NONE',  ( 1.000000000000000000, -0.000000000000000000, -0.000000000000000000 ) ) ;
#168511=AXIS2_PLACEMENT_3D ( 'NONE', #31254, #187736, #7807 ) ;
#168532=VERTEX_POINT ( 'NONE', #41318 ) ;
#168587=FACE_OUTER_BOUND ( 'NONE', #104090, .T. ) ;
#168598=AXIS2_PLACEMENT_3D ( 'NONE', #165248, #85667, #88247 ) ;
#168648=DIRECTION ( 'NONE',  ( -1.000000000000000000, -0.000000000000000000, -0.000000000000000000 ) ) ;
#168650=ORIENTED_EDGE ( 'NONE', *, *, #30080, .F. ) ;
#168710=EDGE_CURVE ( 'NONE', #114106, #148744, #250885, .T. ) ;
#168757=CARTESIAN_POINT ( 'NONE',  ( 23.40000000000005542, 77.83551161375991967, -47.52760213295649550 ) ) ;
#168769=LINE ( 'NONE', #189572, #75764 ) ;
#168849=CARTESIAN_POINT ( 'NONE',  ( -0.8999999999999437339, 67.75000000001118394, -10.02310748452479139 ) ) ;
#168923=VERTEX_POINT ( 'NONE', #230726 ) ;
#169019=FACE_OUTER_BOUND ( 'NONE', #157402, .T. ) ;
#169110=ORIENTED_EDGE ( 'NONE', *, *, #74182, .T. ) ;
#169123=EDGE_CURVE ( 'NONE', #51994, #59493, #30527, .T. ) ;
#169131=DIRECTION ( 'NONE',  ( 1.000000000000000000, -0.000000000000000000, -0.000000000000000000 ) ) ;
#169155=ADVANCED_FACE ( 'NONE', ( #160188 ), #113713, .T. ) ;
#169173=AXIS2_PLACEMENT_3D ( 'NONE', #257093, #38115, #255813 ) ;
#169186=CARTESIAN_POINT ( 'NONE',  ( -23.49999999999994316, 79.78873604695631627, -7.297728304630792806 ) ) ;
#169204=VERTEX_POINT ( 'NONE', #44067 ) ;
#169234=VECTOR ( 'NONE', #49678, 1000.000000000000114 ) ;
#169261=AXIS2_PLACEMENT_3D ( 'NONE', #4156, #164536, #49708 ) ;
#169276=CYLINDRICAL_SURFACE ( 'NONE', #86, 0.09999999999999530098 ) ;
#169312=EDGE_CURVE ( 'NONE', #119288, #82975, #18034, .T. ) ;
#169316=EDGE_CURVE ( 'NONE', #175937, #211183, #230416, .T. ) ;
#169350=EDGE_LOOP ( 'NONE', ( #44256, #75890, #20383, #9410 ) ) ;
#169381=ADVANCED_FACE ( 'NONE', ( #170482 ), #9836, .T. ) ;
#169449=DIRECTION ( 'NONE',  ( 0.000000000000000000, 0.1480365673253036252, -0.9889818879709278976 ) ) ;
#169493=CARTESIAN_POINT ( 'NONE',  ( -20.94999999999994600, 87.75000000001122658, -30.02310748452481448 ) ) ;
#169497=VERTEX_POINT ( 'NONE', #75204 ) ;
#169515=EDGE_CURVE ( 'NONE', #178868, #168923, #113895, .T. ) ;
#169540=FACE_OUTER_BOUND ( 'NONE', #30704, .T. ) ;
#169559=ADVANCED_FACE ( 'NONE', ( #60727, #140262, #256310, #179434, #236807 ), #235522, .T. ) ;
#169586=EDGE_LOOP ( 'NONE', ( #210191, #157393, #39902, #248706 ) ) ;
#169667=EDGE_CURVE ( 'NONE', #211462, #75088, #222356, .T. ) ;
#169701=CARTESIAN_POINT ( 'NONE',  ( 21.05000000000005400, 64.35000000001120668, -3.023107484524792277 ) ) ;
#169724=CARTESIAN_POINT ( 'NONE',  ( -23.49999999999994316, 86.36484105039212977, -51.23044614117323903 ) ) ;
#169835=ORIENTED_EDGE ( 'NONE', *, *, #135431, .T. ) ;
#169841=CIRCLE ( 'NONE', #73962, 0.09999999999999939493 ) ;
#169843=VERTEX_POINT ( 'NONE', #31921 ) ;
#169860=ORIENTED_EDGE ( 'NONE', *, *, #82999, .T. ) ;
#169900=( NAMED_UNIT ( * ) SI_UNIT ( $, .STERADIAN. ) SOLID_ANGLE_UNIT ( ) );
#169962=CARTESIAN_POINT ( 'NONE',  ( -23.49999999999994316, 77.83551161375991967, -47.52760213295649550 ) ) ;
#169986=DIRECTION ( 'NONE',  ( 0.000000000000000000, 0.000000000000000000, -1.000000000000000000 ) ) ;
#170002=ORIENTED_EDGE ( 'NONE', *, *, #182966, .F. ) ;
#170021=LINE ( 'NONE', #243397, #82431 ) ;
#170129=ORIENTED_EDGE ( 'NONE', *, *, #235454, .T. ) ;
#170132=CARTESIAN_POINT ( 'NONE',  ( 0.9000000000000546452, 67.65000000001118963, -5.981686128287480919 ) ) ;
#170150=ORIENTED_EDGE ( 'NONE', *, *, #1338, .T. ) ;
#170169=EDGE_CURVE ( 'NONE', #249282, #210105, #146380, .T. ) ;
#170176=TOROIDAL_SURFACE ( 'NONE', #199168, 0.2000000000000000111, 0.1000000000000000056 ) ;
#170177=CARTESIAN_POINT ( 'NONE',  ( -20.94999999999994600, 66.15000000001120384, -4.623107484524796362 ) ) ;
#170225=TOROIDAL_SURFACE ( 'NONE', #203498, 4.900000000000000355, 0.1000000000000000056 ) ;
#170226=FACE_OUTER_BOUND ( 'NONE', #70093, .T. ) ;
#170231=AXIS2_PLACEMENT_3D ( 'NONE', #255535, #174822, #74427 ) ;
#170338=CARTESIAN_POINT ( 'NONE',  ( 13.40000000000005898, 64.25000000001119815, -18.32310748452479388 ) ) ;
#170435=DIRECTION ( 'NONE',  ( 1.000000000000000000, 0.000000000000000000, 0.000000000000000000 ) ) ;
#170467=AXIS2_PLACEMENT_3D ( 'NONE', #42645, #217415, #19235 ) ;
#170476=EDGE_LOOP ( 'NONE', ( #113087, #120715, #250366, #254045 ) ) ;
#170482=FACE_OUTER_BOUND ( 'NONE', #141723, .T. ) ;
#170499=ORIENTED_EDGE ( 'NONE', *, *, #151999, .T. ) ;
#170556=DIRECTION ( 'NONE',  ( 0.000000000000000000, 0.000000000000000000, 1.000000000000000000 ) ) ;
#170561=CARTESIAN_POINT ( 'NONE',  ( -21.14999999999994174, 87.60324567546805952, -34.17184040628037422 ) ) ;
#170578=CARTESIAN_POINT ( 'NONE',  ( -21.14999999999994174, 73.58898499266442172, -51.80813886865390572 ) ) ;
#170599=ORIENTED_EDGE ( 'NONE', *, *, #181547, .F. ) ;
#170621=AXIS2_PLACEMENT_3D ( 'NONE', #25627, #179582, #201688 ) ;
#170630=VERTEX_POINT ( 'NONE', #147388 ) ;
#170647=ORIENTED_EDGE ( 'NONE', *, *, #58134, .F. ) ;
#170708=ADVANCED_FACE ( 'NONE', ( #60778 ), #181102, .T. ) ;
#170725=ORIENTED_EDGE ( 'NONE', *, *, #234699, .F. ) ;
#170773=ORIENTED_EDGE ( 'NONE', *, *, #117834, .T. ) ;
#170782=EDGE_CURVE ( 'NONE', #88024, #38614, #97841, .T. ) ;
#170859=CARTESIAN_POINT ( 'NONE',  ( -23.49999999999994316, 64.25000000001119815, -3.123107484524795474 ) ) ;
#170877=ORIENTED_EDGE ( 'NONE', *, *, #254228, .T. ) ;
#170914=AXIS2_PLACEMENT_3D ( 'NONE', #44264, #23439, #204597 ) ;
#170933=LINE ( 'NONE', #135582, #182167 ) ;
#170938=VERTEX_POINT ( 'NONE', #62082 ) ;
#170941=DIRECTION ( 'NONE',  ( 1.000000000000000000, 0.000000000000000000, 0.000000000000000000 ) ) ;
#170946=VECTOR ( 'NONE', #110783, 1000.000000000000000 ) ;
#171029=CARTESIAN_POINT ( 'NONE',  ( 21.15000000000004476, 74.83745509109094485, -44.02310748452479316 ) ) ;
#171128=ORIENTED_EDGE ( 'NONE', *, *, #68638, .F. ) ;
#171277=ORIENTED_EDGE ( 'NONE', *, *, #112733, .F. ) ;
#171331=CARTESIAN_POINT ( 'NONE',  ( -23.49999999999994316, 74.26359666348515987, -47.54092689884382850 ) ) ;
#171339=ADVANCED_FACE ( 'NONE', ( #147737 ), #249411, .F. ) ;
#171409=ORIENTED_EDGE ( 'NONE', *, *, #229851, .T. ) ;
#171411=CARTESIAN_POINT ( 'NONE',  ( 23.40000000000005542, 87.51781941433023349, -37.75951082105083145 ) ) ;
#171434=DIRECTION ( 'NONE',  ( -1.284434275755705296E-16, 0.7071067811865471286, 0.7071067811865479058 ) ) ;
#171465=ORIENTED_EDGE ( 'NONE', *, *, #64638, .T. ) ;
#171527=CARTESIAN_POINT ( 'NONE',  ( -21.04999999999994387, 65.15000000001120384, -3.123107484524795474 ) ) ;
#171531=LINE ( 'NONE', #29463, #128991 ) ;
#171534=EDGE_CURVE ( 'NONE', #40979, #101028, #38078, .T. ) ;
#171613=DIRECTION ( 'NONE',  ( 0.000000000000000000, 0.000000000000000000, -1.000000000000000000 ) ) ;
#171645=DIRECTION ( 'NONE',  ( 0.000000000000000000, 0.000000000000000000, 1.000000000000000000 ) ) ;
#171652=EDGE_CURVE ( 'NONE', #133332, #30250, #239909, .T. ) ;
#171684=CYLINDRICAL_SURFACE ( 'NONE', #27615, 0.09999999999999939493 ) ;
#171711=CIRCLE ( 'NONE', #17543, 0.1000000000000028644 ) ;
#171767=DIRECTION ( 'NONE',  ( 1.000000000000000000, 0.000000000000000000, 0.000000000000000000 ) ) ;
#171840=LINE ( 'NONE', #72731, #99157 ) ;
#171842=ORIENTED_EDGE ( 'NONE', *, *, #154169, .F. ) ;
#171868=EDGE_LOOP ( 'NONE', ( #18131, #80379, #30121, #189823 ) ) ;
#171883=CARTESIAN_POINT ( 'NONE',  ( 23.40000000000005542, 77.73640333653723644, -47.54092689884382850 ) ) ;
#171891=EDGE_CURVE ( 'NONE', #109039, #215142, #152602, .T. ) ;
#171896=CARTESIAN_POINT ( 'NONE',  ( -21.14999999999994174, 82.64476912853859858, -26.37791261425322986 ) ) ;
#172006=CYLINDRICAL_SURFACE ( 'NONE', #109379, 0.1000000000000028644 ) ;
#172019=ORIENTED_EDGE ( 'NONE', *, *, #169515, .T. ) ;
#172067=DIRECTION ( 'NONE',  ( 0.000000000000000000, 0.000000000000000000, -1.000000000000000000 ) ) ;
#172115=ORIENTED_EDGE ( 'NONE', *, *, #183615, .F. ) ;
#172129=DIRECTION ( 'NONE',  ( 0.000000000000000000, 0.000000000000000000, 1.000000000000000000 ) ) ;
#172186=VECTOR ( 'NONE', #52956, 1000.000000000000000 ) ;
#172205=EDGE_CURVE ( 'NONE', #73109, #84197, #246229, .T. ) ;
#172213=AXIS2_PLACEMENT_3D ( 'NONE', #42781, #122319, #201849 ) ;
#172259=LINE ( 'NONE', #153982, #137325 ) ;
#172304=VECTOR ( 'NONE', #22441, 1000.000000000000000 ) ;
#172317=VERTEX_POINT ( 'NONE', #12771 ) ;
#172340=DIRECTION ( 'NONE',  ( 1.000000000000000000, -0.000000000000000000, -0.000000000000000000 ) ) ;
#172396=DIRECTION ( 'NONE',  ( 1.000000000000000000, 0.000000000000000000, 0.000000000000000000 ) ) ;
#172435=DIRECTION ( 'NONE',  ( -1.000000000000000000, 0.000000000000000000, 0.000000000000000000 ) ) ;
#172437=DIRECTION ( 'NONE',  ( 1.284434275755705296E-16, -0.7071067811865471286, -0.7071067811865479058 ) ) ;
#172453=DIRECTION ( 'NONE',  ( 0.000000000000000000, 0.000000000000000000, -1.000000000000000000 ) ) ;
#172470=ORIENTED_EDGE ( 'NONE', *, *, #153062, .F. ) ;
#172477=DIRECTION ( 'NONE',  ( 1.000000000000000000, -0.000000000000000000, -0.000000000000000000 ) ) ;
#172495=DIRECTION ( 'NONE',  ( 0.000000000000000000, -0.1332476588733448597, -0.9910827722268067408 ) ) ;
#172506=CARTESIAN_POINT ( 'NONE',  ( -23.49999999999994316, 77.85126707825561709, -47.62635315998165453 ) ) ;
#172530=DIRECTION ( 'NONE',  ( 0.000000000000000000, 0.000000000000000000, -1.000000000000000000 ) ) ;
#172541=TOROIDAL_SURFACE ( 'NONE', #26761, 0.2000000000000000111, 0.1000000000000000056 ) ;
#172546=VECTOR ( 'NONE', #140730, 1000.000000000000000 ) ;
#172560=CIRCLE ( 'NONE', #226662, 0.1000000000000028644 ) ;
#172566=FACE_OUTER_BOUND ( 'NONE', #38724, .T. ) ;
#172576=DIRECTION ( 'NONE',  ( -0.000000000000000000, 0.000000000000000000, -1.000000000000000000 ) ) ;
#172583=DIRECTION ( 'NONE',  ( 8.565286242868724116E-15, -0.1575546449569727447, 0.9875102702516478370 ) ) ;
#172597=EDGE_CURVE ( 'NONE', #50827, #256542, #215310, .T. ) ;
#172638=AXIS2_PLACEMENT_3D ( 'NONE', #108478, #168503, #69370 ) ;
#172670=DIRECTION ( 'NONE',  ( 1.000000000000000000, 0.000000000000000000, -0.000000000000000000 ) ) ;
#172684=VECTOR ( 'NONE', #140820, 1000.000000000000000 ) ;
#172687=ADVANCED_FACE ( 'NONE', ( #98035 ), #176348, .T. ) ;
#172712=DIRECTION ( 'NONE',  ( 0.000000000000000000, 1.000000000000000000, 0.000000000000000000 ) ) ;
#172868=CARTESIAN_POINT ( 'NONE',  ( -23.49999999999994316, 76.00000000001119815, -36.02310748452479316 ) ) ;
#172893=CARTESIAN_POINT ( 'NONE',  ( -21.04999999999994387, 77.16254490893143725, -43.92310748452479885 ) ) ;
#172911=DIRECTION ( 'NONE',  ( 1.284434275755705296E-16, -0.7071067811865471286, 0.7071067811865479058 ) ) ;
#172913=FACE_OUTER_BOUND ( 'NONE', #196178, .T. ) ;
#172996=VECTOR ( 'NONE', #46485, 1000.000000000000000 ) ;
#173008=CIRCLE ( 'NONE', #81349, 0.1999999999999987899 ) ;
#173025=ORIENTED_EDGE ( 'NONE', *, *, #238300, .T. ) ;
#173042=DIRECTION ( 'NONE',  ( 0.000000000000000000, 0.000000000000000000, -1.000000000000000000 ) ) ;
#173155=VERTEX_POINT ( 'NONE', #12741 ) ;
#173183=VERTEX_POINT ( 'NONE', #170561 ) ;
#173212=EDGE_LOOP ( 'NONE', ( #55792, #216259, #66414 ) ) ;
#173238=ORIENTED_EDGE ( 'NONE', *, *, #242076, .F. ) ;
#173245=CIRCLE ( 'NONE', #152374, 2.699999999999999289 ) ;
#173319=DIRECTION ( 'NONE',  ( 3.469446951953515108E-14, -1.000000000000000000, 0.000000000000000000 ) ) ;
#173390=ORIENTED_EDGE ( 'NONE', *, *, #234340, .F. ) ;
#173397=LINE ( 'NONE', #212487, #210121 ) ;
#173414=VECTOR ( 'NONE', #107241, 1000.000000000000000 ) ;
#173470=ORIENTED_EDGE ( 'NONE', *, *, #138522, .F. ) ;
#173698=AXIS2_PLACEMENT_3D ( 'NONE', #174686, #117230, #136776 ) ;
#173704=ORIENTED_EDGE ( 'NONE', *, *, #52095, .F. ) ;
#173783=AXIS2_PLACEMENT_3D ( 'NONE', #161153, #240676, #141576 ) ;
#173795=DIRECTION ( 'NONE',  ( 0.000000000000000000, 1.000000000000000000, -1.224646799147353207E-16 ) ) ;
#173808=SPHERICAL_SURFACE ( 'NONE', #115846, 0.1000000000000000056 ) ;
#173835=DIRECTION ( 'NONE',  ( 0.000000000000000000, 0.000000000000000000, 1.000000000000000000 ) ) ;
#173888=DIRECTION ( 'NONE',  ( -3.469446951953515108E-14, 0.000000000000000000, -1.000000000000000000 ) ) ;
#173931=DIRECTION ( 'NONE',  ( 0.000000000000000000, 0.000000000000000000, 1.000000000000000000 ) ) ;
#173938=CARTESIAN_POINT ( 'NONE',  ( -13.39999999999994529, 64.35000000001120668, -23.72310748452479245 ) ) ;
#173957=ORIENTED_EDGE ( 'NONE', *, *, #243618, .T. ) ;
#173968=AXIS2_PLACEMENT_3D ( 'NONE', #86345, #100143, #256622 ) ;
#173997=ORIENTED_EDGE ( 'NONE', *, *, #52047, .T. ) ;
#174110=AXIS2_PLACEMENT_3D ( 'NONE', #129953, #70029, #88252 ) ;
#174116=DIRECTION ( 'NONE',  ( -1.000000000000000000, -0.000000000000000000, -0.000000000000000000 ) ) ;
#174167=EDGE_CURVE ( 'NONE', #514, #10605, #78097, .T. ) ;
#174226=CARTESIAN_POINT ( 'NONE',  ( -0.8999999999999437339, 64.35000000001120668, -10.02310748452479139 ) ) ;
#174257=DIRECTION ( 'NONE',  ( -1.000000000000000000, -0.000000000000000000, -0.000000000000000000 ) ) ;
#174295=DIRECTION ( 'NONE',  ( 0.000000000000000000, 0.000000000000000000, -1.000000000000000000 ) ) ;
#174339=DIRECTION ( 'NONE',  ( 1.000000000000000000, 0.000000000000000000, 0.000000000000000000 ) ) ;
#174364=CARTESIAN_POINT ( 'NONE',  ( 21.05000000000005400, 83.80000000001119531, -51.02310748452479316 ) ) ;
#174390=ORIENTED_EDGE ( 'NONE', *, *, #188316, .F. ) ;
#174401=EDGE_CURVE ( 'NONE', #250992, #23181, #82352, .T. ) ;
#174413=CARTESIAN_POINT ( 'NONE',  ( 21.15000000000005187, 74.25000000001119815, -47.64205752314703801 ) ) ;
#174440=DIRECTION ( 'NONE',  ( 0.000000000000000000, 0.000000000000000000, -1.000000000000000000 ) ) ;
#174491=CARTESIAN_POINT ( 'NONE',  ( -20.94999999999994600, 66.15000000001120384, -6.023107484524794941 ) ) ;
#174562=LINE ( 'NONE', #75435, #37435 ) ;
#174574=ORIENTED_EDGE ( 'NONE', *, *, #108189, .T. ) ;
#174597=EDGE_CURVE ( 'NONE', #227850, #153040, #45154, .T. ) ;
#174626=DIRECTION ( 'NONE',  ( -0.000000000000000000, -0.000000000000000000, 1.000000000000000000 ) ) ;
#174649=ORIENTED_EDGE ( 'NONE', *, *, #67450, .T. ) ;
#174656=CARTESIAN_POINT ( 'NONE',  ( -21.14999999999994174, 74.94272479589878344, -3.123107484524795474 ) ) ;
#174680=ORIENTED_EDGE ( 'NONE', *, *, #226498, .T. ) ;
#174686=CARTESIAN_POINT ( 'NONE',  ( 23.40000000000005542, 87.50449464844290048, -34.18759587077607165 ) ) ;
#174695=FACE_BOUND ( 'NONE', #122554, .T. ) ;
#174742=ORIENTED_EDGE ( 'NONE', *, *, #40458, .F. ) ;
#174764=TOROIDAL_SURFACE ( 'NONE', #128932, 11.65000000000000036, 0.1000000000000000056 ) ;
#174795=CARTESIAN_POINT ( 'NONE',  ( -5.899999999999938183, 64.35000000001120668, -21.92310748452479174 ) ) ;
#174813=LINE ( 'NONE', #148792, #169234 ) ;
#174822=DIRECTION ( 'NONE',  ( 0.000000000000000000, -1.000000000000000000, 0.000000000000000000 ) ) ;
#174828=LINE ( 'NONE', #117374, #104196 ) ;
#174871=ADVANCED_FACE ( 'NONE', ( #1838 ), #157626, .T. ) ;
#174883=ORIENTED_EDGE ( 'NONE', *, *, #216561, .T. ) ;
#174909=LINE ( 'NONE', #13224, #103124 ) ;
#175058=CARTESIAN_POINT ( 'NONE',  ( -5.899999999999938183, 64.35000000001120668, -22.12310748452479103 ) ) ;
#175071=DIRECTION ( 'NONE',  ( 0.000000000000000000, 0.000000000000000000, 1.000000000000000000 ) ) ;
#175073=DIRECTION ( 'NONE',  ( 1.000000000000000000, 0.000000000000000000, 0.000000000000000000 ) ) ;
#175110=ORIENTED_EDGE ( 'NONE', *, *, #220027, .T. ) ;
#175141=DIRECTION ( 'NONE',  ( 1.000000000000000000, 0.000000000000000000, 0.000000000000000000 ) ) ;
#175150=DIRECTION ( 'NONE',  ( 0.000000000000000000, 0.1332476588733448597, -0.9910827722268067408 ) ) ;
#175160=LINE ( 'NONE', #112580, #116343 ) ;
#175161=AXIS2_PLACEMENT_3D ( 'NONE', #135019, #15110, #56754 ) ;
#175181=CARTESIAN_POINT ( 'NONE',  ( 11.60000000000006182, 64.25000000001119815, -23.72310748452479601 ) ) ;
#175182=ORIENTED_EDGE ( 'NONE', *, *, #215818, .F. ) ;
#175487=DIRECTION ( 'NONE',  ( 0.000000000000000000, 0.000000000000000000, -1.000000000000000000 ) ) ;
#175488=CARTESIAN_POINT ( 'NONE',  ( 21.15000000000004476, 84.00000000001119815, -37.18565239344504647 ) ) ;
#175490=ADVANCED_FACE ( 'NONE', ( #40093 ), #19213, .T. ) ;
#175537=CARTESIAN_POINT ( 'NONE',  ( 23.40000000000005542, 77.83551161375993388, -47.52760213295649550 ) ) ;
#175582=EDGE_CURVE ( 'NONE', #101028, #85681, #3832, .T. ) ;
#175601=ORIENTED_EDGE ( 'NONE', *, *, #215019, .F. ) ;
#175626=ORIENTED_EDGE ( 'NONE', *, *, #50165, .T. ) ;
#175669=EDGE_CURVE ( 'NONE', #12539, #139324, #131144, .T. ) ;
#175686=ORIENTED_EDGE ( 'NONE', *, *, #3574, .T. ) ;
#175702=EDGE_CURVE ( 'NONE', #30427, #40157, #232800, .T. ) ;
#175751=DIRECTION ( 'NONE',  ( -1.000000000000000000, 0.000000000000000000, 0.000000000000000000 ) ) ;
#175782=AXIS2_PLACEMENT_3D ( 'NONE', #218972, #82001, #40389 ) ;
#175822=DIRECTION ( 'NONE',  ( -0.000000000000000000, 1.000000000000000000, -0.000000000000000000 ) ) ;
#175824=CARTESIAN_POINT ( 'NONE',  ( -23.49999999999994316, 74.63923853664559260, -43.99645795275012006 ) ) ;
#175854=EDGE_CURVE ( 'NONE', #116279, #109234, #120746, .T. ) ;
#175869=LINE ( 'NONE', #255326, #254995 ) ;
#175877=AXIS2_PLACEMENT_3D ( 'NONE', #122097, #162522, #2123 ) ;
#175883=DIRECTION ( 'NONE',  ( 1.000000000000000000, -0.000000000000000000, 0.000000000000000000 ) ) ;
#175937=VERTEX_POINT ( 'NONE', #65734 ) ;
#175939=DIRECTION ( 'NONE',  ( 0.000000000000000000, 0.000000000000000000, 1.000000000000000000 ) ) ;
#176077=FACE_OUTER_BOUND ( 'NONE', #139070, .T. ) ;
#176112=CARTESIAN_POINT ( 'NONE',  ( -13.39999999999994529, 64.35000000001120668, -18.42310748452479174 ) ) ;
#176138=CIRCLE ( 'NONE', #46908, 0.1000000000000032391 ) ;
#176162=FACE_OUTER_BOUND ( 'NONE', #98124, .T. ) ;
#176230=VECTOR ( 'NONE', #116907, 1000.000000000000000 ) ;
#176264=ADVANCED_FACE ( 'NONE', ( #116917 ), #49977, .T. ) ;
#176294=DIRECTION ( 'NONE',  ( 1.000000000000000000, -0.000000000000000000, 0.000000000000000000 ) ) ;
#176348=CYLINDRICAL_SURFACE ( 'NONE', #169173, 0.09999999999999939493 ) ;
#176356=EDGE_LOOP ( 'NONE', ( #189373, #238516, #40761, #80651 ) ) ;
#176394=LINE ( 'NONE', #137239, #140898 ) ;
#176437=CARTESIAN_POINT ( 'NONE',  ( -23.49999999999994316, 76.00000000001119815, -36.02310748452479316 ) ) ;
#176468=FACE_OUTER_BOUND ( 'NONE', #212790, .T. ) ;
#176476=DIRECTION ( 'NONE',  ( -1.000000000000000000, 0.000000000000000000, 0.000000000000000000 ) ) ;
#176509=VERTEX_POINT ( 'NONE', #46347 ) ;
#176518=CARTESIAN_POINT ( 'NONE',  ( 23.40000000000005187, 83.90000000001120384, -37.27310748452479316 ) ) ;
#176621=EDGE_CURVE ( 'NONE', #239496, #169204, #217204, .T. ) ;
#176658=EDGE_CURVE ( 'NONE', #6487, #197879, #1472, .T. ) ;
#176744=ADVANCED_FACE ( 'NONE', ( #188 ), #4045, .F. ) ;
#176841=ORIENTED_EDGE ( 'NONE', *, *, #175854, .T. ) ;
#176952=ORIENTED_EDGE ( 'NONE', *, *, #115538, .F. ) ;
#176985=FACE_OUTER_BOUND ( 'NONE', #56519, .T. ) ;
#177045=FACE_OUTER_BOUND ( 'NONE', #93962, .T. ) ;
#177057=ORIENTED_EDGE ( 'NONE', *, *, #69337, .T. ) ;
#177133=ORIENTED_EDGE ( 'NONE', *, *, #73316, .F. ) ;
#177183=AXIS2_PLACEMENT_3D ( 'NONE', #195015, #78874, #95879 ) ;
#177206=DIRECTION ( 'NONE',  ( -1.000000000000000000, 0.000000000000000000, 0.000000000000000000 ) ) ;
#177217=DIRECTION ( 'NONE',  ( -1.000000000000000000, 0.000000000000000000, 0.000000000000000000 ) ) ;
#177230=CARTESIAN_POINT ( 'NONE',  ( 21.15000000000005187, 77.83551161375991967, -47.62760213295649692 ) ) ;
#177242=EDGE_CURVE ( 'NONE', #33031, #195816, #104103, .T. ) ;
#177533=ORIENTED_EDGE ( 'NONE', *, *, #244501, .T. ) ;
#177553=DIRECTION ( 'NONE',  ( 0.000000000000000000, -1.000000000000000000, 0.000000000000000000 ) ) ;
#177577=CARTESIAN_POINT ( 'NONE',  ( 20.95000000000005258, 64.25000000001119815, -6.123107484524794586 ) ) ;
#177600=CYLINDRICAL_SURFACE ( 'NONE', #245476, 0.1000000000000028644 ) ;
#177612=TOROIDAL_SURFACE ( 'NONE', #77587, 0.2000000000000000111, 0.1000000000000000056 ) ;
#177623=VERTEX_POINT ( 'NONE', #171527 ) ;
#177685=DIRECTION ( 'NONE',  ( -0.000000000000000000, 0.1332476588733589318, -0.9910827722268049644 ) ) ;
#177797=EDGE_CURVE ( 'NONE', #169204, #103163, #86521, .T. ) ;
#177798=ORIENTED_EDGE ( 'NONE', *, *, #243225, .F. ) ;
#177854=DIRECTION ( 'NONE',  ( 1.000000000000000000, 0.000000000000000000, -0.000000000000000000 ) ) ;
#177900=EDGE_LOOP ( 'NONE', ( #228693, #72506, #136955 ) ) ;
#177965=DIRECTION ( 'NONE',  ( -0.000000000000000000, 1.000000000000000000, -0.000000000000000000 ) ) ;
#178031=ADVANCED_FACE ( 'NONE', ( #52508 ), #102703, .T. ) ;
#178130=CARTESIAN_POINT ( 'NONE',  ( -21.04999999999994387, 84.00000000001119815, -37.18565239344504647 ) ) ;
#178162=DIRECTION ( 'NONE',  ( 0.000000000000000000, 0.000000000000000000, -1.000000000000000000 ) ) ;
#178175=AXIS2_PLACEMENT_3D ( 'NONE', #109417, #188976, #130267 ) ;
#178217=VERTEX_POINT ( 'NONE', #39413 ) ;
#178225=LINE ( 'NONE', #216024, #223120 ) ;
#178324=TOROIDAL_SURFACE ( 'NONE', #82577, 0.2000000000000000111, 0.1000000000000000056 ) ;
#178333=DIRECTION ( 'NONE',  ( -1.000000000000000000, 0.000000000000000000, 0.000000000000000000 ) ) ;
#178342=DIRECTION ( 'NONE',  ( 0.000000000000000000, 0.000000000000000000, -1.000000000000000000 ) ) ;
#178344=EDGE_CURVE ( 'NONE', #1569, #106796, #48750, .T. ) ;
#178428=CARTESIAN_POINT ( 'NONE',  ( -20.94999999999994245, 67.75000000001118394, -3.123107484524795474 ) ) ;
#178447=FACE_OUTER_BOUND ( 'NONE', #135425, .T. ) ;
#178497=AXIS2_PLACEMENT_3D ( 'NONE', #255685, #172396, #134479 ) ;
#178589=AXIS2_PLACEMENT_3D ( 'NONE', #217515, #139253, #214964 ) ;
#178706=DIRECTION ( 'NONE',  ( 1.000000000000000000, -0.000000000000000000, 0.000000000000000000 ) ) ;
#178739=CARTESIAN_POINT ( 'NONE',  ( 20.95000000000005969, 61.64150943397345372, -36.51839050339276582 ) ) ;
#178743=TOROIDAL_SURFACE ( 'NONE', #87096, 0.2000000000000000111, 0.1000000000000000056 ) ;
#178833=CIRCLE ( 'NONE', #66371, 0.1000000000000028644 ) ;
#178838=ORIENTED_EDGE ( 'NONE', *, *, #56196, .T. ) ;
#178868=VERTEX_POINT ( 'NONE', #78829 ) ;
#178887=EDGE_LOOP ( 'NONE', ( #110027, #139257, #108534, #55923 ) ) ;
#178904=CARTESIAN_POINT ( 'NONE',  ( -23.49999999999994316, 74.16448838626247664, -47.62760213295649692 ) ) ;
#178925=CARTESIAN_POINT ( 'NONE',  ( -0.8999999999999437339, 64.25000000001119815, -7.323107484524790323 ) ) ;
#178938=ORIENTED_EDGE ( 'NONE', *, *, #103283, .T. ) ;
#178971=DIRECTION ( 'NONE',  ( 0.000000000000000000, -1.000000000000000000, 0.000000000000000000 ) ) ;
#178995=LINE ( 'NONE', #255869, #97648 ) ;
#179055=LINE ( 'NONE', #141182, #134885 ) ;
#179057=CARTESIAN_POINT ( 'NONE',  ( 23.50000000000005684, 74.94272479589878344, -8.023107484524793165 ) ) ;
#179079=CARTESIAN_POINT ( 'NONE',  ( 21.15000000000003055, 84.00000000001119815, -37.18565239344504647 ) ) ;
#179096=ADVANCED_FACE ( 'NONE', ( #16042 ), #10888, .T. ) ;
#179137=ADVANCED_FACE ( 'NONE', ( #111268 ), #178324, .T. ) ;
#179141=DIRECTION ( 'NONE',  ( 1.000000000000000000, -0.000000000000000000, 0.000000000000000000 ) ) ;
#179227=EDGE_CURVE ( 'NONE', #201062, #41849, #176394, .T. ) ;
#179261=DIRECTION ( 'NONE',  ( -0.000000000000000000, -1.000000000000000000, 0.000000000000000000 ) ) ;
#179269=DIRECTION ( 'NONE',  ( -3.469446951953501855E-14, 0.1575546449569757979, -0.9875102702516471709 ) ) ;
#179303=VERTEX_POINT ( 'NONE', #219336 ) ;
#179323=FACE_OUTER_BOUND ( 'NONE', #99221, .T. ) ;
#179332=CARTESIAN_POINT ( 'NONE',  ( -23.39999999999994529, 76.00000000001119815, -36.02310748452479316 ) ) ;
#179398=FACE_OUTER_BOUND ( 'NONE', #240181, .T. ) ;
#179434=FACE_BOUND ( 'NONE', #66537, .T. ) ;
#179467=CARTESIAN_POINT ( 'NONE',  ( 23.50000000000005684, 82.64476912853859858, -26.37791261425322986 ) ) ;
#179478=ADVANCED_FACE ( 'NONE', ( #47103 ), #83646, .F. ) ;
#179500=EDGE_LOOP ( 'NONE', ( #229804, #41572, #92570 ) ) ;
#179523=FACE_OUTER_BOUND ( 'NONE', #246613, .T. ) ;
#179524=VERTEX_POINT ( 'NONE', #241484 ) ;
#179561=CARTESIAN_POINT ( 'NONE',  ( -23.49999999999994316, 76.00000000001119815, -36.02310748452479316 ) ) ;
#179579=ADVANCED_FACE ( 'NONE', ( #70576 ), #13148, .T. ) ;
#179582=DIRECTION ( 'NONE',  ( -1.000000000000000000, 0.000000000000000000, 0.000000000000000000 ) ) ;
#179595=AXIS2_PLACEMENT_3D ( 'NONE', #145856, #164157, #45485 ) ;
#179603=CARTESIAN_POINT ( 'NONE',  ( 5.551115123125782702E-14, 64.75000000001119815, -25.92310748452479174 ) ) ;
#179702=DIRECTION ( 'NONE',  ( -0.000000000000000000, 0.000000000000000000, 1.000000000000000000 ) ) ;
#179745=CARTESIAN_POINT ( 'NONE',  ( 21.05000000000005400, 66.25000000001119815, -5.923107484524795296 ) ) ;
#179751=ORIENTED_EDGE ( 'NONE', *, *, #168166, .F. ) ;
#179754=ORIENTED_EDGE ( 'NONE', *, *, #29502, .T. ) ;
#179768=DIRECTION ( 'NONE',  ( -0.000000000000000000, -0.000000000000000000, 1.000000000000000000 ) ) ;
#179797=EDGE_LOOP ( 'NONE', ( #10230, #2707, #170647, #100311 ) ) ;
#179799=AXIS2_PLACEMENT_3D ( 'NONE', #137831, #874, #80401 ) ;
#179805=VERTEX_POINT ( 'NONE', #31001 ) ;
#179815=EDGE_CURVE ( 'NONE', #23611, #12539, #131342, .T. ) ;
#179823=ORIENTED_EDGE ( 'NONE', *, *, #175854, .F. ) ;
#179896=CYLINDRICAL_SURFACE ( 'NONE', #117266, 0.09999999999999939493 ) ;
#179917=EDGE_CURVE ( 'NONE', #45940, #195803, #149644, .T. ) ;
#179918=DIRECTION ( 'NONE',  ( -1.000000000000000000, 0.000000000000000000, 0.000000000000000000 ) ) ;
#179952=CIRCLE ( 'NONE', #155026, 0.09999999999999635569 ) ;
#179955=CARTESIAN_POINT ( 'NONE',  ( 21.15000000000005187, 76.00000000001119815, -31.87310748452479459 ) ) ;
#179988=CARTESIAN_POINT ( 'NONE',  ( -20.94999999999994600, 65.19115966511134275, -30.12310748452479103 ) ) ;
#180033=EDGE_CURVE ( 'NONE', #123853, #139130, #80002, .T. ) ;
#180085=ORIENTED_EDGE ( 'NONE', *, *, #54126, .F. ) ;
#180229=DIRECTION ( 'NONE',  ( 1.000000000000000000, 0.000000000000000000, 0.000000000000000000 ) ) ;
#180242=EDGE_LOOP ( 'NONE', ( #59188, #257680, #150226, #155704 ) ) ;
#180253=CARTESIAN_POINT ( 'NONE',  ( 11.60000000000006182, 63.75000000001119815, -21.02310748452479316 ) ) ;
#180323=DIRECTION ( 'NONE',  ( 0.000000000000000000, 0.000000000000000000, -1.000000000000000000 ) ) ;
#180329=DIRECTION ( 'NONE',  ( 0.000000000000000000, 0.000000000000000000, 1.000000000000000000 ) ) ;
#180406=DIRECTION ( 'NONE',  ( 1.000000000000000000, 0.000000000000000000, 0.000000000000000000 ) ) ;
#180414=AXIS2_PLACEMENT_3D ( 'NONE', #98458, #97173, #56776 ) ;
#180417=DIRECTION ( 'NONE',  ( -1.000000000000000000, 0.000000000000000000, 0.000000000000000000 ) ) ;
#180439=AXIS2_PLACEMENT_3D ( 'NONE', #41022, #180515, #103517 ) ;
#180496=CIRCLE ( 'NONE', #122228, 0.09999999999999982514 ) ;
#180515=DIRECTION ( 'NONE',  ( 1.000000000000000000, 0.000000000000000000, -0.000000000000000000 ) ) ;
#180670=AXIS2_PLACEMENT_3D ( 'NONE', #93630, #131474, #136588 ) ;
#180703=ORIENTED_EDGE ( 'NONE', *, *, #77210, .F. ) ;
#180749=DIRECTION ( 'NONE',  ( 0.000000000000000000, 0.000000000000000000, -1.000000000000000000 ) ) ;
#180786=DIRECTION ( 'NONE',  ( -0.000000000000000000, -0.9910827722268049644, 0.1332476588733589318 ) ) ;
#180801=ORIENTED_EDGE ( 'NONE', *, *, #52973, .F. ) ;
#180802=DIRECTION ( 'NONE',  ( 0.000000000000000000, 0.000000000000000000, 1.000000000000000000 ) ) ;
#180832=DIRECTION ( 'NONE',  ( 1.000000000000000000, -0.000000000000000000, -0.000000000000000000 ) ) ;
#180836=CARTESIAN_POINT ( 'NONE',  ( -21.04999999999994387, 67.75000000001119815, -30.12310748452479459 ) ) ;
#180860=CARTESIAN_POINT ( 'NONE',  ( -0.8999999999999437339, 67.75000000001118394, -7.423107484524793520 ) ) ;
#180889=CARTESIAN_POINT ( 'NONE',  ( -21.14999999999994174, 83.90000000001120384, -34.77310748452479316 ) ) ;
#180928=LINE ( 'NONE', #23158, #163219 ) ;
#180960=CARTESIAN_POINT ( 'NONE',  ( 21.15000000000005542, 65.15000000001120384, -3.023107484524792277 ) ) ;
#180987=DIRECTION ( 'NONE',  ( -1.000000000000000000, 0.000000000000000000, -0.000000000000000000 ) ) ;
#180992=LINE ( 'NONE', #205659, #142791 ) ;
#180994=FACE_OUTER_BOUND ( 'NONE', #190474, .T. ) ;
#181021=DIRECTION ( 'NONE',  ( 1.000000000000000000, 0.000000000000000000, 0.000000000000000000 ) ) ;
#181102=TOROIDAL_SURFACE ( 'NONE', #164533, 4.150000000000000355, 0.1000000000000000056 ) ;
#181113=CARTESIAN_POINT ( 'NONE',  ( 0.9000000000000547562, 67.75000000001118394, -7.423107484524793520 ) ) ;
#181165=AXIS2_PLACEMENT_3D ( 'NONE', #3668, #61080, #182334 ) ;
#181170=ORIENTED_EDGE ( 'NONE', *, *, #26916, .T. ) ;
#181234=ORIENTED_EDGE ( 'NONE', *, *, #158079, .F. ) ;
#181341=ORIENTED_EDGE ( 'NONE', *, *, #100935, .T. ) ;
#181347=CIRCLE ( 'NONE', #247954, 4.041421356237306917 ) ;
#181349=CARTESIAN_POINT ( 'NONE',  ( -21.14999999999994174, 79.88763423575340994, -7.282924647898262549 ) ) ;
#181373=ORIENTED_EDGE ( 'NONE', *, *, #217003, .F. ) ;
#181374=ORIENTED_EDGE ( 'NONE', *, *, #59944, .F. ) ;
#181398=CARTESIAN_POINT ( 'NONE',  ( 23.40000000000004476, 74.83745509109094485, -44.02310748452479316 ) ) ;
#181421=CARTESIAN_POINT ( 'NONE',  ( -23.39999999999994529, 77.73640333653723644, -47.54092689884382850 ) ) ;
#181433=ORIENTED_EDGE ( 'NONE', *, *, #47424, .F. ) ;
#181455=AXIS2_PLACEMENT_3D ( 'NONE', #246485, #226924, #127838 ) ;
#181537=CIRCLE ( 'NONE', #2429, 0.1000000000000028644 ) ;
#181547=EDGE_CURVE ( 'NONE', #60723, #62069, #92087, .T. ) ;
#181550=CARTESIAN_POINT ( 'NONE',  ( 21.15000000000005542, 64.25000000001119815, -3.023107484524792277 ) ) ;
#181553=CARTESIAN_POINT ( 'NONE',  ( -23.49999999999994316, 76.00000000001119815, -36.02310748452479316 ) ) ;
#181577=CARTESIAN_POINT ( 'NONE',  ( 21.15000000000005542, 67.85000000001119247, -3.123107484524795474 ) ) ;
#181691=DIRECTION ( 'NONE',  ( 0.000000000000000000, 0.000000000000000000, -1.000000000000000000 ) ) ;
#181696=FACE_OUTER_BOUND ( 'NONE', #132124, .T. ) ;
#181707=AXIS2_PLACEMENT_3D ( 'NONE', #118397, #141785, #182217 ) ;
#181726=CARTESIAN_POINT ( 'NONE',  ( -20.94999999999994600, 66.15000000001120384, -5.923107484524795296 ) ) ;
#181735=CIRCLE ( 'NONE', #173783, 0.1000000000000028644 ) ;
#181776=ORIENTED_EDGE ( 'NONE', *, *, #182060, .T. ) ;
#181814=VECTOR ( 'NONE', #226645, 1000.000000000000000 ) ;
#181818=DIRECTION ( 'NONE',  ( 0.000000000000000000, -1.000000000000000000, 0.000000000000000000 ) ) ;
#181819=EDGE_LOOP ( 'NONE', ( #188000, #160256, #148107 ) ) ;
#181891=AXIS2_PLACEMENT_3D ( 'NONE', #231414, #31942, #73641 ) ;
#181904=VECTOR ( 'NONE', #73776, 1000.000000000000000 ) ;
#181923=ADVANCED_FACE ( 'NONE', ( #184998, #161607 ), #242390, .T. ) ;
#181924=ORIENTED_EDGE ( 'NONE', *, *, #179227, .T. ) ;
#182008=LINE ( 'NONE', #144132, #47957 ) ;
#182046=ORIENTED_EDGE ( 'NONE', *, *, #30080, .T. ) ;
#182060=EDGE_CURVE ( 'NONE', #116777, #14829, #92269, .T. ) ;
#182074=ADVANCED_FACE ( 'NONE', ( #229271 ), #127595, .T. ) ;
#182098=LINE ( 'NONE', #226321, #52854 ) ;
#182132=EDGE_LOOP ( 'NONE', ( #13355, #211143, #48739, #177798 ) ) ;
#182155=CARTESIAN_POINT ( 'NONE',  ( -21.14999999999994174, 64.35000000001120668, -3.123107484524795474 ) ) ;
#182167=VECTOR ( 'NONE', #152631, 1000.000000000000000 ) ;
#182188=ADVANCED_FACE ( 'NONE', ( #16645 ), #118305, .F. ) ;
#182217=DIRECTION ( 'NONE',  ( 0.000000000000000000, 0.000000000000000000, -1.000000000000000000 ) ) ;
#182245=EDGE_CURVE ( 'NONE', #121144, #21187, #246408, .T. ) ;
#182311=AXIS2_PLACEMENT_3D ( 'NONE', #236576, #99616, #218287 ) ;
#182334=DIRECTION ( 'NONE',  ( 0.000000000000000000, -0.000000000000000000, 1.000000000000000000 ) ) ;
#182361=CARTESIAN_POINT ( 'NONE',  ( -13.39999999999994529, 67.75000000001118394, -21.02310748452479316 ) ) ;
#182412=FACE_OUTER_BOUND ( 'NONE', #147975, .T. ) ;
#182432=VERTEX_POINT ( 'NONE', #23071 ) ;
#182494=CARTESIAN_POINT ( 'NONE',  ( 23.40000000000005187, 76.00000000001119815, -36.02310748452479316 ) ) ;
#182525=CARTESIAN_POINT ( 'NONE',  ( -21.04999999999994387, 67.85000000001119247, -3.123107484524795474 ) ) ;
#182547=TOROIDAL_SURFACE ( 'NONE', #70127, 4.041421356237312246, 0.1000000000000000056 ) ;
#182566=AXIS2_PLACEMENT_3D ( 'NONE', #79534, #100375, #219051 ) ;
#182577=ORIENTED_EDGE ( 'NONE', *, *, #64847, .T. ) ;
#182605=AXIS2_PLACEMENT_3D ( 'NONE', #114266, #174295, #37315 ) ;
#182608=AXIS2_PLACEMENT_3D ( 'NONE', #112626, #190907, #150478 ) ;
#182612=ORIENTED_EDGE ( 'NONE', *, *, #64746, .F. ) ;
#182657=ORIENTED_EDGE ( 'NONE', *, *, #62876, .T. ) ;
#182658=DIRECTION ( 'NONE',  ( 0.000000000000000000, 0.1332476588733589318, -0.9910827722268050755 ) ) ;
#182674=ORIENTED_EDGE ( 'NONE', *, *, #126415, .F. ) ;
#182692=VECTOR ( 'NONE', #57316, 1000.000000000000000 ) ;
#182708=ADVANCED_FACE ( 'NONE', ( #231529 ), #33358, .F. ) ;
#182739=EDGE_LOOP ( 'NONE', ( #225293, #128367, #173704, #120971 ) ) ;
#182815=AXIS2_PLACEMENT_3D ( 'NONE', #248115, #210293, #29123 ) ;
#182822=EDGE_CURVE ( 'NONE', #97363, #214650, #141956, .T. ) ;
#182841=CARTESIAN_POINT ( 'NONE',  ( 21.05000000000005400, 82.84256550613280012, -26.34830530078816935 ) ) ;
#182867=DIRECTION ( 'NONE',  ( 0.000000000000000000, -1.000000000000000000, 0.000000000000000000 ) ) ;
#182907=AXIS2_PLACEMENT_3D ( 'NONE', #123451, #247232, #68617 ) ;
#182910=LINE ( 'NONE', #142471, #93010 ) ;
#182966=EDGE_CURVE ( 'NONE', #149012, #170938, #233743, .T. ) ;
#182983=CARTESIAN_POINT ( 'NONE',  ( -23.49999999999994316, 64.25000000001119815, -3.123107484524795474 ) ) ;
#182997=AXIS2_PLACEMENT_3D ( 'NONE', #149659, #50508, #210891 ) ;
#183057=DIRECTION ( 'NONE',  ( 0.000000000000000000, -0.4856429311786307212, -0.8741572761215384846 ) ) ;
#183067=CARTESIAN_POINT ( 'NONE',  ( -0.8999999999999425127, 64.35000000001120668, -7.423107484524793520 ) ) ;
#183102=ORIENTED_EDGE ( 'NONE', *, *, #99644, .T. ) ;
#183107=ORIENTED_EDGE ( 'NONE', *, *, #187811, .T. ) ;
#183166=AXIS2_PLACEMENT_3D ( 'NONE', #258042, #119893, #199424 ) ;
#183226=VERTEX_POINT ( 'NONE', #104194 ) ;
#183328=CYLINDRICAL_SURFACE ( 'NONE', #246806, 0.1000000000000028644 ) ;
#183366=DIRECTION ( 'NONE',  ( -1.000000000000000000, 0.000000000000000000, -0.000000000000000000 ) ) ;
#183369=VERTEX_POINT ( 'NONE', #26819 ) ;
#183384=CARTESIAN_POINT ( 'NONE',  ( -23.49999999999994316, 79.88763423575340994, -7.282924647898262549 ) ) ;
#183421=CARTESIAN_POINT ( 'NONE',  ( 11.60000000000006182, 66.35000000001119247, -18.42310748452479530 ) ) ;
#183430=AXIS2_PLACEMENT_3D ( 'NONE', #20951, #154063, #19646 ) ;
#183478=CYLINDRICAL_SURFACE ( 'NONE', #86806, 0.09999999999999530098 ) ;
#183479=DIRECTION ( 'NONE',  ( 0.000000000000000000, 0.000000000000000000, -1.000000000000000000 ) ) ;
#183513=DIRECTION ( 'NONE',  ( 0.000000000000000000, 0.000000000000000000, -1.000000000000000000 ) ) ;
#183518=AXIS2_PLACEMENT_3D ( 'NONE', #237032, #242153, #23140 ) ;
#183553=CARTESIAN_POINT ( 'NONE',  ( 5.900000000000059863, 64.25000000001119815, -26.12310748452479103 ) ) ;
#183572=AXIS2_PLACEMENT_3D ( 'NONE', #150535, #151838, #213060 ) ;
#183615=EDGE_CURVE ( 'NONE', #197543, #118259, #96512, .T. ) ;
#183634=AXIS2_PLACEMENT_3D ( 'NONE', #204819, #127877, #70501 ) ;
#183678=CARTESIAN_POINT ( 'NONE',  ( 21.05000000000005400, 86.36484105039212977, -51.23044614117323903 ) ) ;
#183690=ORIENTED_EDGE ( 'NONE', *, *, #16409, .F. ) ;
#183691=DIRECTION ( 'NONE',  ( 0.000000000000000000, -0.000000000000000000, 1.000000000000000000 ) ) ;
#183699=DIRECTION ( 'NONE',  ( 0.000000000000000000, 0.000000000000000000, -1.000000000000000000 ) ) ;
#183728=CARTESIAN_POINT ( 'NONE',  ( -23.39999999999994529, 76.00000000001119815, -36.02310748452479316 ) ) ;
#183796=FACE_OUTER_BOUND ( 'NONE', #47691, .T. ) ;
#183859=ORIENTED_EDGE ( 'NONE', *, *, #193369, .T. ) ;
#183888=ADVANCED_FACE ( 'NONE', ( #114634 ), #192898, .T. ) ;
#183958=ORIENTED_EDGE ( 'NONE', *, *, #235000, .T. ) ;
#183979=CARTESIAN_POINT ( 'NONE',  ( -5.899999999999938183, 64.75000000001119815, -25.92310748452479174 ) ) ;
#184020=CARTESIAN_POINT ( 'NONE',  ( -23.39999999999994529, 74.16448838626247664, -47.52760213295649550 ) ) ;
#184062=VERTEX_POINT ( 'NONE', #61070 ) ;
#184111=DIRECTION ( 'NONE',  ( 0.000000000000000000, 0.000000000000000000, -1.000000000000000000 ) ) ;
#184127=DIRECTION ( 'NONE',  ( -1.000000000000000000, 0.000000000000000000, -0.000000000000000000 ) ) ;
#184155=EDGE_CURVE ( 'NONE', #167941, #248236, #146674, .T. ) ;
#184229=AXIS2_PLACEMENT_3D ( 'NONE', #31741, #250742, #173835 ) ;
#184274=CIRCLE ( 'NONE', #213501, 0.09999999999999939493 ) ;
#184306=ORIENTED_EDGE ( 'NONE', *, *, #17466, .F. ) ;
#184326=AXIS2_PLACEMENT_3D ( 'NONE', #46895, #106876, #129030 ) ;
#184353=CARTESIAN_POINT ( 'NONE',  ( -6.099999999999939249, 64.35000000001120668, -51.02310748452479316 ) ) ;
#184359=ORIENTED_EDGE ( 'NONE', *, *, #97713, .F. ) ;
#184388=CARTESIAN_POINT ( 'NONE',  ( -21.14999999999994174, 64.35000000001120668, -3.123107484524795474 ) ) ;
#184394=SPHERICAL_SURFACE ( 'NONE', #94405, 0.1000000000000000056 ) ;
#184434=AXIS2_PLACEMENT_3D ( 'NONE', #239704, #75514, #256632 ) ;
#184447=DIRECTION ( 'NONE',  ( 0.000000000000000000, 0.000000000000000000, -1.000000000000000000 ) ) ;
#184458=DIRECTION ( 'NONE',  ( 0.000000000000000000, 0.9910827722268049644, -0.1332476588733589040 ) ) ;
#184515=ADVANCED_FACE ( 'NONE', ( #218205 ), #23917, .F. ) ;
#184547=CARTESIAN_POINT ( 'NONE',  ( -23.49999999999994316, 77.16254490893143725, -43.82310748452479743 ) ) ;
#184620=VERTEX_POINT ( 'NONE', #44746 ) ;
#184649=DIRECTION ( 'NONE',  ( 0.000000000000000000, 0.1332476588733589318, 0.9910827722268049644 ) ) ;
#184662=VERTEX_POINT ( 'NONE', #148994 ) ;
#184673=DIRECTION ( 'NONE',  ( -0.000000000000000000, 0.000000000000000000, -1.000000000000000000 ) ) ;
#184676=CIRCLE ( 'NONE', #180414, 0.1000000000000028644 ) ;
#184688=CARTESIAN_POINT ( 'NONE',  ( 21.05000000000005400, 74.94272479589878344, -3.123107484524795474 ) ) ;
#184702=FACE_OUTER_BOUND ( 'NONE', #12360, .T. ) ;
#184727=AXIS2_PLACEMENT_3D ( 'NONE', #5309, #230835, #15649 ) ;
#184747=DIRECTION ( 'NONE',  ( 1.000000000000000000, -0.000000000000000000, 0.000000000000000000 ) ) ;
#184756=AXIS2_PLACEMENT_3D ( 'NONE', #197085, #18464, #52432 ) ;
#184778=ORIENTED_EDGE ( 'NONE', *, *, #168478, .T. ) ;
#184801=DIRECTION ( 'NONE',  ( 1.000000000000000000, 0.000000000000000000, 0.000000000000000000 ) ) ;
#184936=DIRECTION ( 'NONE',  ( 0.000000000000000000, 0.000000000000000000, 1.000000000000000000 ) ) ;
#184960=ORIENTED_EDGE ( 'NONE', *, *, #128540, .T. ) ;
#184970=FACE_OUTER_BOUND ( 'NONE', #163093, .T. ) ;
#184997=FACE_OUTER_BOUND ( 'NONE', #238084, .T. ) ;
#184998=FACE_BOUND ( 'NONE', #226081, .T. ) ;
#185026=DIRECTION ( 'NONE',  ( -1.000000000000000000, -0.000000000000000000, -0.000000000000000000 ) ) ;
#185036=ORIENTED_EDGE ( 'NONE', *, *, #241026, .T. ) ;
#185051=DIRECTION ( 'NONE',  ( -0.000000000000000000, 0.000000000000000000, -1.000000000000000000 ) ) ;
#185065=CARTESIAN_POINT ( 'NONE',  ( -21.14999999999994174, 77.83551161375991967, -47.62760213295649692 ) ) ;
#185089=VECTOR ( 'NONE', #24489, 1000.000000000000114 ) ;
#185122=( NAMED_UNIT ( * ) SI_UNIT ( $, .STERADIAN. ) SOLID_ANGLE_UNIT ( ) );
#185150=AXIS2_PLACEMENT_3D ( 'NONE', #57677, #18578, #194675 ) ;
#185162=ORIENTED_EDGE ( 'NONE', *, *, #201940, .T. ) ;
#185167=DIRECTION ( 'NONE',  ( 1.000000000000000000, -0.000000000000000000, 0.000000000000000000 ) ) ;
#185211=ADVANCED_FACE ( 'NONE', ( #115979 ), #136799, .F. ) ;
#185293=EDGE_CURVE ( 'NONE', #11972, #69129, #60029, .T. ) ;
#185378=PLANE ( 'NONE',  #226635 ) ;
#185384=ORIENTED_EDGE ( 'NONE', *, *, #35563, .T. ) ;
#185390=AXIS2_PLACEMENT_3D ( 'NONE', #85860, #123745, #27242 ) ;
#185393=DIRECTION ( 'NONE',  ( 0.000000000000000000, -0.000000000000000000, 1.000000000000000000 ) ) ;
#185396=ORIENTED_EDGE ( 'NONE', *, *, #55748, .T. ) ;
#185412=EDGE_LOOP ( 'NONE', ( #233658, #142061, #206221 ) ) ;
#185442=TOROIDAL_SURFACE ( 'NONE', #118811, 0.2000000000000000111, 0.1000000000000000056 ) ;
#185449=AXIS2_PLACEMENT_3D ( 'NONE', #59085, #133526, #115248 ) ;
#185541=DIRECTION ( 'NONE',  ( 0.000000000000000000, -1.000000000000000000, 0.000000000000000000 ) ) ;
#185556=( LENGTH_UNIT ( ) NAMED_UNIT ( * ) SI_UNIT ( .MILLI., .METRE. ) );
#185612=CARTESIAN_POINT ( 'NONE',  ( -21.04999999999994387, 57.01194402951015405, -45.05752083424646059 ) ) ;
#185659=EDGE_LOOP ( 'NONE', ( #36787, #66547, #177133, #90784 ) ) ;
#185765=LINE ( 'NONE', #166236, #97785 ) ;
#185767=LINE ( 'NONE', #24145, #130420 ) ;
#185785=ORIENTED_EDGE ( 'NONE', *, *, #2437, .T. ) ;
#185827=CARTESIAN_POINT ( 'NONE',  ( -21.04999999999994387, 83.80000000001119531, -51.02310748452479316 ) ) ;
#185863=ORIENTED_EDGE ( 'NONE', *, *, #168478, .F. ) ;
#185909=CYLINDRICAL_SURFACE ( 'NONE', #175877, 0.1000000000000002554 ) ;
#185967=CARTESIAN_POINT ( 'NONE',  ( -23.49999999999994316, 77.25000000001119815, -43.92310748452479885 ) ) ;
#185980=DIRECTION ( 'NONE',  ( -1.000000000000000000, 0.000000000000000000, 0.000000000000000000 ) ) ;
#186011=ADVANCED_FACE ( 'NONE', ( #50217 ), #52786, .T. ) ;
#186023=EDGE_LOOP ( 'NONE', ( #73453, #113240, #196330, #69476 ) ) ;
#186031=VECTOR ( 'NONE', #165652, 1000.000000000000000 ) ;
#186045=ADVANCED_FACE ( 'NONE', ( #62758 ), #121478, .T. ) ;
#186080=EDGE_CURVE ( 'NONE', #45216, #74886, #214343, .T. ) ;
#186109=VERTEX_POINT ( 'NONE', #219249 ) ;
#186120=ORIENTED_EDGE ( 'NONE', *, *, #96629, .T. ) ;
#186122=AXIS2_PLACEMENT_3D ( 'NONE', #252647, #192700, #210977 ) ;
#186192=EDGE_LOOP ( 'NONE', ( #141909, #197253, #107047, #40617 ) ) ;
#186219=TOROIDAL_SURFACE ( 'NONE', #7122, 0.2000000000000000111, 0.1000000000000000056 ) ;
#186235=ADVANCED_FACE ( 'NONE', ( #125306 ), #204817, .T. ) ;
#186241=ORIENTED_EDGE ( 'NONE', *, *, #204943, .T. ) ;
#186243=CIRCLE ( 'NONE', #144521, 0.1000000000000002554 ) ;
#186266=DIRECTION ( 'NONE',  ( -1.713057248573685501E-14, 0.9875102702516477260, 0.1575546449569727447 ) ) ;
#186268=PLANE ( 'NONE',  #196019 ) ;
#186302=DIRECTION ( 'NONE',  ( 0.000000000000000000, 0.000000000000000000, 1.000000000000000000 ) ) ;
#186359=ORIENTED_EDGE ( 'NONE', *, *, #225314, .F. ) ;
#186363=CARTESIAN_POINT ( 'NONE',  ( -21.14999999999994174, 74.16448838626247664, -47.52760213295649550 ) ) ;
#186403=CIRCLE ( 'NONE', #111553, 0.1000000000000028644 ) ;
#186445=ORIENTED_EDGE ( 'NONE', *, *, #17389, .T. ) ;
#186467=DIRECTION ( 'NONE',  ( 0.000000000000000000, 1.000000000000000000, -0.000000000000000000 ) ) ;
#186471=VERTEX_POINT ( 'NONE', #116023 ) ;
#186584=CARTESIAN_POINT ( 'NONE',  ( -23.49999999999994316, 84.00000000001119815, -34.86056257560453986 ) ) ;
#186612=LINE ( 'NONE', #6663, #21341 ) ;
#186650=EDGE_CURVE ( 'NONE', #234836, #184062, #222890, .T. ) ;
#186658=ORIENTED_EDGE ( 'NONE', *, *, #229851, .F. ) ;
#186680=CARTESIAN_POINT ( 'NONE',  ( -23.49999999999994316, 87.51781941433023349, -34.28670414799875488 ) ) ;
#186686=AXIS2_PLACEMENT_3D ( 'NONE', #39282, #1390, #22275 ) ;
#186697=AXIS2_PLACEMENT_3D ( 'NONE', #249501, #150408, #172576 ) ;
#186716=ADVANCED_FACE ( 'NONE', ( #85828 ), #227826, .T. ) ;
#186730=AXIS2_PLACEMENT_3D ( 'NONE', #113920, #253424, #12282 ) ;
#186825=CARTESIAN_POINT ( 'NONE',  ( -20.94999999999994600, 87.75000000001119815, -6.023107484524794941 ) ) ;
#186827=DIRECTION ( 'NONE',  ( 1.000000000000000000, 0.000000000000000000, 0.000000000000000000 ) ) ;
#186841=CARTESIAN_POINT ( 'NONE',  ( -20.94999999999994245, 67.75000000001118394, -25.49719488170504533 ) ) ;
#186848=DIRECTION ( 'NONE',  ( 1.000000000000000000, -0.000000000000000000, -0.000000000000000000 ) ) ;
#186852=PLANE ( 'NONE',  #157580 ) ;
#186860=CIRCLE ( 'NONE', #236714, 2.600000000000000089 ) ;
#186877=DIRECTION ( 'NONE',  ( 0.000000000000000000, -0.8741572761215385956, 0.4856429311786307768 ) ) ;
#186900=VERTEX_POINT ( 'NONE', #137805 ) ;
#186923=DIRECTION ( 'NONE',  ( 1.000000000000000000, -0.000000000000000000, -0.000000000000000000 ) ) ;
#186977=PLANE ( 'NONE',  #5588 ) ;
#186986=ORIENTED_EDGE ( 'NONE', *, *, #50165, .F. ) ;
#186991=VERTEX_POINT ( 'NONE', #243337 ) ;
#187011=EDGE_CURVE ( 'NONE', #191399, #166555, #182098, .T. ) ;
#187064=CYLINDRICAL_SURFACE ( 'NONE', #69811, 4.049999999999998046 ) ;
#187095=AXIS2_PLACEMENT_3D ( 'NONE', #143202, #41575, #27155 ) ;
#187100=CYLINDRICAL_SURFACE ( 'NONE', #55361, 2.600000000000000089 ) ;
#187146=FACE_OUTER_BOUND ( 'NONE', #169586, .T. ) ;
#187156=VERTEX_POINT ( 'NONE', #119107 ) ;
#187163=ORIENTED_EDGE ( 'NONE', *, *, #234884, .F. ) ;
#187179=CARTESIAN_POINT ( 'NONE',  ( -5.899999999999938183, 64.75000000001119815, -36.02310748452479316 ) ) ;
#187301=DIRECTION ( 'NONE',  ( -0.000000000000000000, 1.000000000000000000, -0.000000000000000000 ) ) ;
#187306=DIRECTION ( 'NONE',  ( -1.000000000000000000, 0.000000000000000000, 0.000000000000000000 ) ) ;
#187352=DIRECTION ( 'NONE',  ( 1.000000000000000000, -0.000000000000000000, -0.000000000000000000 ) ) ;
#187361=DIRECTION ( 'NONE',  ( 0.000000000000000000, -1.000000000000000000, 0.000000000000000000 ) ) ;
#187393=FACE_OUTER_BOUND ( 'NONE', #70090, .T. ) ;
#187396=ORIENTED_EDGE ( 'NONE', *, *, #97292, .F. ) ;
#187434=VERTEX_POINT ( 'NONE', #12172 ) ;
#187459=ORIENTED_EDGE ( 'NONE', *, *, #246975, .T. ) ;
#187528=ORIENTED_EDGE ( 'NONE', *, *, #180033, .T. ) ;
#187553=VERTEX_POINT ( 'NONE', #241471 ) ;
#187582=FACE_OUTER_BOUND ( 'NONE', #102446, .T. ) ;
#187626=AXIS2_PLACEMENT_3D ( 'NONE', #92067, #33428, #109060 ) ;
#187736=DIRECTION ( 'NONE',  ( 0.000000000000000000, -0.000000000000000000, -1.000000000000000000 ) ) ;
#187742=CIRCLE ( 'NONE', #204460, 0.1000000000000045852 ) ;
#187747=VERTEX_POINT ( 'NONE', #83632 ) ;
#187760=EDGE_LOOP ( 'NONE', ( #181776, #92423, #66281 ) ) ;
#187801=DIRECTION ( 'NONE',  ( 0.000000000000000000, 0.000000000000000000, -1.000000000000000000 ) ) ;
#187811=EDGE_CURVE ( 'NONE', #224621, #21018, #256478, .T. ) ;
#187920=LINE ( 'NONE', #202331, #10977 ) ;
#187957=CIRCLE ( 'NONE', #50553, 0.1000000000000021844 ) ;
#187990=FACE_OUTER_BOUND ( 'NONE', #54778, .T. ) ;
#188000=ORIENTED_EDGE ( 'NONE', *, *, #206805, .F. ) ;
#188049=ADVANCED_FACE ( 'NONE', ( #142985 ), #222528, .F. ) ;
#188053=EDGE_LOOP ( 'NONE', ( #175110, #233339, #207779, #253842 ) ) ;
#188058=AXIS2_PLACEMENT_3D ( 'NONE', #199075, #79100, #180802 ) ;
#188081=DIRECTION ( 'NONE',  ( -1.000000000000000000, 0.000000000000000000, 0.000000000000000000 ) ) ;
#188086=CARTESIAN_POINT ( 'NONE',  ( -23.39999999999994529, 87.50449464844290048, -34.18759587077607165 ) ) ;
#188090=CIRCLE ( 'NONE', #59049, 0.09999999999999982514 ) ;
#188125=ORIENTED_EDGE ( 'NONE', *, *, #188694, .F. ) ;
#188127=( NAMED_UNIT ( * ) PLANE_ANGLE_UNIT ( ) SI_UNIT ( $, .RADIAN. ) );
#188182=AXIS2_PLACEMENT_3D ( 'NONE', #183979, #5311, #144840 ) ;
#188203=DIRECTION ( 'NONE',  ( 1.000000000000000000, 0.000000000000000000, 0.000000000000000000 ) ) ;
#188217=PLANE ( 'NONE',  #7661 ) ;
#188233=DIRECTION ( 'NONE',  ( 0.000000000000000000, 0.1332476588733589318, -0.9910827722268049644 ) ) ;
#188258=ORIENTED_EDGE ( 'NONE', *, *, #217050, .T. ) ;
#188316=EDGE_CURVE ( 'NONE', #186991, #196305, #52892, .T. ) ;
#188323=ORIENTED_EDGE ( 'NONE', *, *, #62942, .F. ) ;
#188352=DIRECTION ( 'NONE',  ( 0.000000000000000000, 0.000000000000000000, 1.000000000000000000 ) ) ;
#188361=DIRECTION ( 'NONE',  ( 0.000000000000000000, 0.000000000000000000, 1.000000000000000000 ) ) ;
#188399=ADVANCED_FACE ( 'NONE', ( #104825 ), #184394, .T. ) ;
#188496=VECTOR ( 'NONE', #208639, 1000.000000000000000 ) ;
#188521=DIRECTION ( 'NONE',  ( 0.000000000000000000, 0.1575546449569757979, 0.9875102702516471709 ) ) ;
#188564=CARTESIAN_POINT ( 'NONE',  ( 13.40000000000005898, 67.75000000001118394, -16.98168612828748891 ) ) ;
#188579=CYLINDRICAL_SURFACE ( 'NONE', #40053, 0.1000000000000002554 ) ;
#188583=CYLINDRICAL_SURFACE ( 'NONE', #55817, 0.1000000000000002554 ) ;
#188694=EDGE_CURVE ( 'NONE', #21878, #64265, #138527, .T. ) ;
#188754=ORIENTED_EDGE ( 'NONE', *, *, #157382, .F. ) ;
#188769=DIRECTION ( 'NONE',  ( -1.000000000000000000, 0.000000000000000000, 0.000000000000000000 ) ) ;
#188817=DIRECTION ( 'NONE',  ( -1.040834085586050557E-13, 0.1575546449569757979, -0.9875102702516471709 ) ) ;
#188888=LINE ( 'NONE', #10259, #135462 ) ;
#188915=CARTESIAN_POINT ( 'NONE',  ( 21.05000000000005400, 76.00000000001119815, -31.87310748452479459 ) ) ;
#188925=CYLINDRICAL_SURFACE ( 'NONE', #105110, 2.599999999999998312 ) ;
#188937=CARTESIAN_POINT ( 'NONE',  ( -23.49999999999994316, 83.80000000001119531, -51.02310748452479316 ) ) ;
#188976=DIRECTION ( 'NONE',  ( 0.000000000000000000, -1.000000000000000000, 0.000000000000000000 ) ) ;
#189073=CARTESIAN_POINT ( 'NONE',  ( 0.9000000000000547562, 64.25000000001119815, -12.72310748452479245 ) ) ;
#189131=CARTESIAN_POINT ( 'NONE',  ( -0.8999999999999438449, 67.72071067812984779, -13.99381816264344813 ) ) ;
#189156=DIRECTION ( 'NONE',  ( 0.000000000000000000, 1.000000000000000000, 0.000000000000000000 ) ) ;
#189178=CARTESIAN_POINT ( 'NONE',  ( -23.39999999999994529, 77.83551161375991967, -47.52760213295649550 ) ) ;
#189224=DIRECTION ( 'NONE',  ( -0.000000000000000000, -0.000000000000000000, 1.000000000000000000 ) ) ;
#189233=AXIS2_PLACEMENT_3D ( 'NONE', #107420, #190852, #150426 ) ;
#189242=ADVANCED_FACE ( 'NONE', ( #241218 ), #39177, .T. ) ;
#189270=ORIENTED_EDGE ( 'NONE', *, *, #10581, .T. ) ;
#189276=DIRECTION ( 'NONE',  ( 1.000000000000000000, 0.000000000000000000, 0.000000000000000000 ) ) ;
#189282=ADVANCED_FACE ( 'NONE', ( #183796 ), #206636, .T. ) ;
#189299=CARTESIAN_POINT ( 'NONE',  ( 21.05000000000005400, 77.16254490893143725, -43.82310748452479743 ) ) ;
#189318=ORIENTED_EDGE ( 'NONE', *, *, #72723, .T. ) ;
#189336=VERTEX_POINT ( 'NONE', #164248 ) ;
#189373=ORIENTED_EDGE ( 'NONE', *, *, #67100, .T. ) ;
#189381=ORIENTED_EDGE ( 'NONE', *, *, #230793, .T. ) ;
#189446=DIRECTION ( 'NONE',  ( -0.000000000000000000, 1.000000000000000000, 0.000000000000000000 ) ) ;
#189486=CARTESIAN_POINT ( 'NONE',  ( 21.15000000000003055, 84.00000000001119815, -34.86056257560453986 ) ) ;
#189516=LINE ( 'NONE', #52546, #122805 ) ;
#189518=CYLINDRICAL_SURFACE ( 'NONE', #141928, 11.74999999999999645 ) ;
#189533=ORIENTED_EDGE ( 'NONE', *, *, #142766, .T. ) ;
#189550=EDGE_CURVE ( 'NONE', #114575, #151679, #117100, .T. ) ;
#189572=CARTESIAN_POINT ( 'NONE',  ( 21.05000000000003979, 83.98667523412385094, -34.76145429838185663 ) ) ;
#189612=EDGE_LOOP ( 'NONE', ( #222944, #210856, #241884, #2533 ) ) ;
#189617=AXIS2_PLACEMENT_3D ( 'NONE', #168849, #108816, #253462 ) ;
#189678=EDGE_CURVE ( 'NONE', #77791, #221278, #69475, .T. ) ;
#189684=CARTESIAN_POINT ( 'NONE',  ( 21.15000000000005542, 87.51781941433023349, -37.75951082105083145 ) ) ;
#189686=CYLINDRICAL_SURFACE ( 'NONE', #209335, 0.09999999999999635569 ) ;
#189720=DIRECTION ( 'NONE',  ( 0.000000000000000000, 0.1480365673253023762, -0.9889818879709281196 ) ) ;
#189759=AXIS2_PLACEMENT_3D ( 'NONE', #96599, #19676, #220444 ) ;
#189823=ORIENTED_EDGE ( 'NONE', *, *, #38183, .T. ) ;
#189859=DIRECTION ( 'NONE',  ( 1.000000000000000000, 0.000000000000000000, 0.000000000000000000 ) ) ;
#189956=ORIENTED_EDGE ( 'NONE', *, *, #175582, .T. ) ;
#189961=DIRECTION ( 'NONE',  ( 0.000000000000000000, 0.000000000000000000, -1.000000000000000000 ) ) ;
#189995=VERTEX_POINT ( 'NONE', #90153 ) ;
#190064=DIRECTION ( 'NONE',  ( 0.000000000000000000, 0.000000000000000000, -1.000000000000000000 ) ) ;
#190065=CARTESIAN_POINT ( 'NONE',  ( -23.39999999999994529, 84.00000000001119815, -34.86056257560453986 ) ) ;
#190121=DIRECTION ( 'NONE',  ( 1.000000000000000000, 0.000000000000000000, 0.000000000000000000 ) ) ;
#190134=EDGE_CURVE ( 'NONE', #132923, #62069, #174909, .T. ) ;
#190139=AXIS2_PLACEMENT_3D ( 'NONE', #58120, #155990, #195120 ) ;
#190146=EDGE_CURVE ( 'NONE', #108159, #109234, #254360, .T. ) ;
#190157=CIRCLE ( 'NONE', #77682, 0.09999999999999939493 ) ;
#190167=ORIENTED_EDGE ( 'NONE', *, *, #58134, .T. ) ;
#190216=FACE_OUTER_BOUND ( 'NONE', #14593, .T. ) ;
#190251=CARTESIAN_POINT ( 'NONE',  ( -20.94999999999994600, 66.15000000001114699, -51.02310748452476474 ) ) ;
#190255=ADVANCED_FACE ( 'NONE', ( #140866 ), #239971, .F. ) ;
#190307=EDGE_CURVE ( 'NONE', #165490, #182432, #217802, .T. ) ;
#190338=DIRECTION ( 'NONE',  ( -0.000000000000000000, 0.000000000000000000, -1.000000000000000000 ) ) ;
#190377=MANIFOLD_SOLID_BREP ( 'Stock-MAS-200-1', #224133 ) ;
#190442=VECTOR ( 'NONE', #146240, 1000.000000000000000 ) ;
#190443=FACE_OUTER_BOUND ( 'NONE', #67917, .T. ) ;
#190458=ADVANCED_FACE ( 'NONE', ( #129008 ), #53254, .T. ) ;
#190465=CIRCLE ( 'NONE', #65524, 11.74999999999999645 ) ;
#190474=EDGE_LOOP ( 'NONE', ( #38752, #153989, #55566, #104899 ) ) ;
#190477=AXIS2_PLACEMENT_3D ( 'NONE', #153764, #233275, #54597 ) ;
#190501=CARTESIAN_POINT ( 'NONE',  ( 21.15000000000005542, 77.26165318615413469, -44.00978271863746016 ) ) ;
#190528=EDGE_CURVE ( 'NONE', #126736, #52328, #49150, .T. ) ;
#190543=DIRECTION ( 'NONE',  ( 1.000000000000000000, 0.000000000000000000, 0.000000000000000000 ) ) ;
#190553=DIRECTION ( 'NONE',  ( 1.000000000000000000, 0.000000000000000000, -0.000000000000000000 ) ) ;
#190648=( GEOMETRIC_REPRESENTATION_CONTEXT ( 3 ) GLOBAL_UNCERTAINTY_ASSIGNED_CONTEXT ( ( #126045 ) ) GLOBAL_UNIT_ASSIGNED_CONTEXT ( ( #164287, #106851, #185122 ) ) REPRESENTATION_CONTEXT ( 'NONE', 'WORKASPACE' ) );
#190667=AXIS2_PLACEMENT_3D ( 'NONE', #252904, #138081, #135511 ) ;
#190704=LINE ( 'NONE', #152869, #61082 ) ;
#190781=DIRECTION ( 'NONE',  ( -1.000000000000000000, 0.000000000000000000, 0.000000000000000000 ) ) ;
#190839=ORIENTED_EDGE ( 'NONE', *, *, #77273, .F. ) ;
#190852=DIRECTION ( 'NONE',  ( -0.000000000000000000, -0.000000000000000000, 1.000000000000000000 ) ) ;
#190871=ORIENTED_EDGE ( 'NONE', *, *, #238300, .F. ) ;
#190890=AXIS2_PLACEMENT_3D ( 'NONE', #206234, #4170, #202382 ) ;
#190901=ORIENTED_EDGE ( 'NONE', *, *, #29198, .T. ) ;
#190907=DIRECTION ( 'NONE',  ( 0.000000000000000000, -0.000000000000000000, 1.000000000000000000 ) ) ;
#190935=LINE ( 'NONE', #30573, #217333 ) ;
#190938=VERTEX_POINT ( 'NONE', #110395 ) ;
#190949=FACE_OUTER_BOUND ( 'NONE', #103767, .T. ) ;
#190961=DIRECTION ( 'NONE',  ( 0.000000000000000000, 0.000000000000000000, 1.000000000000000000 ) ) ;
#190997=ORIENTED_EDGE ( 'NONE', *, *, #20775, .F. ) ;
#191002=DIRECTION ( 'NONE',  ( 1.000000000000000000, 0.000000000000000000, 0.000000000000000000 ) ) ;
#191038=ORIENTED_EDGE ( 'NONE', *, *, #224199, .T. ) ;
#191048=ADVANCED_FACE ( 'NONE', ( #246892 ), #188217, .T. ) ;
#191055=ADVANCED_FACE ( 'NONE', ( #207810 ), #149317, .T. ) ;
#191102=ADVANCED_FACE ( 'NONE', ( #17175 ), #97944, .T. ) ;
#191133=AXIS2_PLACEMENT_3D ( 'NONE', #108291, #88688, #168304 ) ;
#191210=CARTESIAN_POINT ( 'NONE',  ( -23.49999999999994316, 82.78482233730476025, -26.42994920107286916 ) ) ;
#191279=VERTEX_POINT ( 'NONE', #165677 ) ;
#191290=DIRECTION ( 'NONE',  ( 1.000000000000000000, 0.000000000000000000, 0.000000000000000000 ) ) ;
#191319=DIRECTION ( 'NONE',  ( 0.000000000000000000, 0.1332476588733448597, -0.9910827722268067408 ) ) ;
#191342=LINE ( 'NONE', #73965, #246929 ) ;
#191346=CARTESIAN_POINT ( 'NONE',  ( -23.49999999999994316, 83.97335046823651794, -34.66234602115918051 ) ) ;
#191365=DIRECTION ( 'NONE',  ( 0.000000000000000000, -0.000000000000000000, 1.000000000000000000 ) ) ;
#191399=VERTEX_POINT ( 'NONE', #189073 ) ;
#191400=DIRECTION ( 'NONE',  ( 0.000000000000000000, -0.9910827722268055195, 0.1332476588733540468 ) ) ;
#191419=ORIENTED_EDGE ( 'NONE', *, *, #168294, .F. ) ;
#191432=CARTESIAN_POINT ( 'NONE',  ( -21.04999999999994387, 78.11805852053666399, -49.62915779269638961 ) ) ;
#191474=ORIENTED_EDGE ( 'NONE', *, *, #112734, .T. ) ;
#191509=FACE_OUTER_BOUND ( 'NONE', #120492, .T. ) ;
#191514=EDGE_CURVE ( 'NONE', #168923, #191279, #124727, .T. ) ;
#191551=CIRCLE ( 'NONE', #54137, 0.09999999999999939493 ) ;
#191554=DIRECTION ( 'NONE',  ( 0.000000000000000000, 0.000000000000000000, 1.000000000000000000 ) ) ;
#191588=ORIENTED_EDGE ( 'NONE', *, *, #77961, .T. ) ;
#191589=ADVANCED_FACE ( 'NONE', ( #119822, #174695, #254159, #138062 ), #198042, .T. ) ;
#191615=EDGE_CURVE ( 'NONE', #244869, #21878, #99739, .T. ) ;
#191630=DIRECTION ( 'NONE',  ( -0.000000000000000000, 1.000000000000000000, -0.000000000000000000 ) ) ;
#191637=ORIENTED_EDGE ( 'NONE', *, *, #138717, .T. ) ;
#191662=ORIENTED_EDGE ( 'NONE', *, *, #149757, .F. ) ;
#191769=DIRECTION ( 'NONE',  ( 0.000000000000000000, 1.000000000000000000, 0.000000000000000000 ) ) ;
#191865=CARTESIAN_POINT ( 'NONE',  ( 21.05000000000005400, 65.15000000001120384, -4.523107484524794053 ) ) ;
#191897=CIRCLE ( 'NONE', #54483, 0.09999999999999982514 ) ;
#191922=EDGE_LOOP ( 'NONE', ( #232903, #82386, #89695, #83095 ) ) ;
#191926=AXIS2_PLACEMENT_3D ( 'NONE', #34689, #16410, #95909 ) ;
#191960=ORIENTED_EDGE ( 'NONE', *, *, #257733, .F. ) ;
#192011=CARTESIAN_POINT ( 'NONE',  ( 23.40000000000005542, 82.74366731733570646, -26.36310895752070138 ) ) ;
#192018=CARTESIAN_POINT ( 'NONE',  ( 20.95000000000005258, 65.35000000001120668, -4.523107484524794053 ) ) ;
#192061=DIRECTION ( 'NONE',  ( 0.000000000000000000, -1.000000000000000000, 0.000000000000000000 ) ) ;
#192070=ORIENTED_EDGE ( 'NONE', *, *, #205065, .T. ) ;
#192107=ORIENTED_EDGE ( 'NONE', *, *, #94129, .F. ) ;
#192109=ORIENTED_EDGE ( 'NONE', *, *, #83734, .F. ) ;
#192150=LINE ( 'NONE', #175181, #30166 ) ;
#192242=VECTOR ( 'NONE', #168389, 1000.000000000000000 ) ;
#192267=ADVANCED_FACE ( 'NONE', ( #220836 ), #239128, .F. ) ;
#192409=EDGE_CURVE ( 'NONE', #33086, #49193, #254072, .T. ) ;
#192430=CARTESIAN_POINT ( 'NONE',  ( 21.15000000000005542, 87.51781941433023349, -34.28670414799875488 ) ) ;
#192453=CIRCLE ( 'NONE', #200844, 2.600000000000000089 ) ;
#192462=CARTESIAN_POINT ( 'NONE',  ( 23.50000000000005684, 76.00000000001119815, -36.02310748452479316 ) ) ;
#192515=EDGE_CURVE ( 'NONE', #12539, #241392, #229334, .T. ) ;
#192552=DIRECTION ( 'NONE',  ( -1.284434275755705789E-16, 0.7071067811865472397, 0.7071067811865479058 ) ) ;
#192567=DIRECTION ( 'NONE',  ( -0.000000000000000000, -0.000000000000000000, -1.000000000000000000 ) ) ;
#192569=DIRECTION ( 'NONE',  ( 0.000000000000000000, 0.1480365673253065395, -0.9889818879709274535 ) ) ;
#192583=VECTOR ( 'NONE', #164981, 1000.000000000000000 ) ;
#192584=DIRECTION ( 'NONE',  ( 0.000000000000000000, 0.9910827722268055195, 0.1332476588733540468 ) ) ;
#192609=DIRECTION ( 'NONE',  ( 0.000000000000000000, 1.000000000000000000, 0.000000000000000000 ) ) ;
#192643=TOROIDAL_SURFACE ( 'NONE', #201190, 4.041421356237312246, 0.1000000000000000056 ) ;
#192652=DIRECTION ( 'NONE',  ( 1.000000000000000000, -0.000000000000000000, -0.000000000000000000 ) ) ;
#192700=DIRECTION ( 'NONE',  ( -0.000000000000000000, 0.000000000000000000, 1.000000000000000000 ) ) ;
#192712=CARTESIAN_POINT ( 'NONE',  ( 23.40000000000005187, 74.16448838626247664, -47.52760213295649550 ) ) ;
#192781=CARTESIAN_POINT ( 'NONE',  ( 20.95000000000005613, 67.75000000001118394, -25.49719488170504533 ) ) ;
#192793=DIRECTION ( 'NONE',  ( -0.000000000000000000, 1.000000000000000000, -0.000000000000000000 ) ) ;
#192834=CARTESIAN_POINT ( 'NONE',  ( 21.15000000000005542, 77.16254490893143725, -43.82310748452479743 ) ) ;
#192845=CARTESIAN_POINT ( 'NONE',  ( -21.14999999999994174, 87.50449464844290048, -37.85861909827351468 ) ) ;
#192849=ORIENTED_EDGE ( 'NONE', *, *, #21985, .F. ) ;
#192853=AXIS2_PLACEMENT_3D ( 'NONE', #232114, #96414, #92569 ) ;
#192885=VERTEX_POINT ( 'NONE', #256410 ) ;
#192898=PLANE ( 'NONE',  #217317 ) ;
#192929=CIRCLE ( 'NONE', #80443, 0.1999999999999987899 ) ;
#193020=EDGE_CURVE ( 'NONE', #18100, #186991, #203991, .T. ) ;
#193071=DIRECTION ( 'NONE',  ( 1.000000000000000000, -0.000000000000000000, -0.000000000000000000 ) ) ;
#193118=EDGE_CURVE ( 'NONE', #145505, #119288, #171531, .T. ) ;
#193141=CARTESIAN_POINT ( 'NONE',  ( -20.94999999999994600, 64.35000000001119247, -5.923107484524795296 ) ) ;
#193165=PRODUCT_DEFINITION_SHAPE ( 'NONE', 'NONE',  #152080 ) ;
#193214=ORIENTED_EDGE ( 'NONE', *, *, #197695, .T. ) ;
#193225=DIRECTION ( 'NONE',  ( 1.000000000000000000, -0.000000000000000000, 0.000000000000000000 ) ) ;
#193369=EDGE_CURVE ( 'NONE', #161116, #24547, #43553, .T. ) ;
#193380=DIRECTION ( 'NONE',  ( 0.000000000000000000, 0.000000000000000000, -1.000000000000000000 ) ) ;
#193404=CARTESIAN_POINT ( 'NONE',  ( -21.14999999999994174, 65.87745128126655914, -37.09527722473000466 ) ) ;
#193481=EDGE_CURVE ( 'NONE', #80879, #200341, #191551, .T. ) ;
#193543=CIRCLE ( 'NONE', #247697, 0.09999999999999530098 ) ;
#193545=AXIS2_PLACEMENT_3D ( 'NONE', #107748, #212006, #189859 ) ;
#193627=ORIENTED_EDGE ( 'NONE', *, *, #65408, .F. ) ;
#193705=ORIENTED_EDGE ( 'NONE', *, *, #15540, .T. ) ;
#193741=FACE_OUTER_BOUND ( 'NONE', #121439, .T. ) ;
#193789=EDGE_CURVE ( 'NONE', #5207, #148744, #245872, .T. ) ;
#193846=ADVANCED_FACE ( 'NONE', ( #141059 ), #2806, .T. ) ;
#193910=FACE_OUTER_BOUND ( 'NONE', #158631, .T. ) ;
#193938=AXIS2_PLACEMENT_3D ( 'NONE', #9937, #128606, #245988 ) ;
#193999=DIRECTION ( 'NONE',  ( 0.000000000000000000, 0.000000000000000000, 1.000000000000000000 ) ) ;
#194053=ADVANCED_FACE ( 'NONE', ( #113474 ), #255504, .F. ) ;
#194079=DIRECTION ( 'NONE',  ( 1.000000000000000000, -0.000000000000000000, -0.000000000000000000 ) ) ;
#194088=ORIENTED_EDGE ( 'NONE', *, *, #170782, .T. ) ;
#194124=DIRECTION ( 'NONE',  ( 0.000000000000000000, 1.000000000000000000, 0.000000000000000000 ) ) ;
#194185=CARTESIAN_POINT ( 'NONE',  ( 21.05000000000005400, 83.80000000001119531, -37.18565239344504647 ) ) ;
#194209=AXIS2_PLACEMENT_3D ( 'NONE', #170177, #11052, #153174 ) ;
#194232=LINE ( 'NONE', #155111, #39338 ) ;
#194272=PLANE ( 'NONE',  #253788 ) ;
#194320=DIRECTION ( 'NONE',  ( 0.000000000000000000, 0.000000000000000000, 1.000000000000000000 ) ) ;
#194373=ORIENTED_EDGE ( 'NONE', *, *, #42974, .F. ) ;
#194383=VECTOR ( 'NONE', #96233, 1000.000000000000114 ) ;
#194403=AXIS2_PLACEMENT_3D ( 'NONE', #128194, #207746, #29139 ) ;
#194449=ORIENTED_EDGE ( 'NONE', *, *, #250558, .F. ) ;
#194456=DIRECTION ( 'NONE',  ( 0.000000000000000000, -0.9889818879709272315, -0.1480365673253073999 ) ) ;
#194474=CIRCLE ( 'NONE', #206917, 0.09999999999999939493 ) ;
#194487=VERTEX_POINT ( 'NONE', #59245 ) ;
#194613=CARTESIAN_POINT ( 'NONE',  ( 5.551115123125782702E-14, 76.00000000001119815, -3.023107484524792277 ) ) ;
#194675=DIRECTION ( 'NONE',  ( 0.000000000000000000, -0.1332476588733448597, 0.9910827722268067408 ) ) ;
#194756=DIRECTION ( 'NONE',  ( 0.000000000000000000, -1.387778780781442141E-13, 1.000000000000000000 ) ) ;
#194843=EDGE_CURVE ( 'NONE', #173155, #121523, #34081, .T. ) ;
#194854=AXIS2_PLACEMENT_3D ( 'NONE', #72903, #194124, #152438 ) ;
#195015=CARTESIAN_POINT ( 'NONE',  ( 11.60000000000006004, 67.72071067812984779, -21.02310748452479316 ) ) ;
#195051=FACE_OUTER_BOUND ( 'NONE', #93374, .T. ) ;
#195066=VECTOR ( 'NONE', #46777, 1000.000000000000000 ) ;
#195090=ORIENTED_EDGE ( 'NONE', *, *, #175702, .T. ) ;
#195120=DIRECTION ( 'NONE',  ( 0.000000000000000000, 0.000000000000000000, 1.000000000000000000 ) ) ;
#195125=CIRCLE ( 'NONE', #103500, 0.1000000000000032391 ) ;
#195144=DIRECTION ( 'NONE',  ( 0.000000000000000000, -1.000000000000000000, 0.000000000000000000 ) ) ;
#195155=CARTESIAN_POINT ( 'NONE',  ( -23.39999999999994529, 76.00000000001119815, -36.02310748452479316 ) ) ;
#195164=CYLINDRICAL_SURFACE ( 'NONE', #202518, 0.09999999999999635569 ) ;
#195225=CARTESIAN_POINT ( 'NONE',  ( 6.100000000000062705, 64.25000000001119815, -22.12310748452479103 ) ) ;
#195266=CYLINDRICAL_SURFACE ( 'NONE', #132198, 0.09999999999999939493 ) ;
#195399=DIRECTION ( 'NONE',  ( 0.000000000000000000, 1.000000000000000000, 0.000000000000000000 ) ) ;
#195418=ORIENTED_EDGE ( 'NONE', *, *, #155742, .T. ) ;
#195472=EDGE_CURVE ( 'NONE', #129355, #80209, #109400, .T. ) ;
#195484=DIRECTION ( 'NONE',  ( -0.000000000000000000, 0.1575546449569769913, 0.9875102702516470599 ) ) ;
#195528=CARTESIAN_POINT ( 'NONE',  ( 20.95000000000005258, 65.35000000001120668, -4.623107484524796362 ) ) ;
#195542=VECTOR ( 'NONE', #205403, 1000.000000000000000 ) ;
#195544=ORIENTED_EDGE ( 'NONE', *, *, #206805, .T. ) ;
#195593=ORIENTED_EDGE ( 'NONE', *, *, #148497, .T. ) ;
#195634=DIRECTION ( 'NONE',  ( 0.000000000000000000, 0.000000000000000000, 1.000000000000000000 ) ) ;
#195713=CARTESIAN_POINT ( 'NONE',  ( -11.59999999999994458, 64.25000000001119815, -23.72310748452479245 ) ) ;
#195736=ORIENTED_EDGE ( 'NONE', *, *, #92045, .F. ) ;
#195755=EDGE_CURVE ( 'NONE', #22457, #56611, #35611, .T. ) ;
#195764=CIRCLE ( 'NONE', #45898, 0.1000000000000028644 ) ;
#195803=VERTEX_POINT ( 'NONE', #199806 ) ;
#195816=VERTEX_POINT ( 'NONE', #62838 ) ;
#195819=DIRECTION ( 'NONE',  ( 1.000000000000000000, 0.000000000000000000, 0.000000000000000000 ) ) ;
#195820=VECTOR ( 'NONE', #61249, 1000.000000000000000 ) ;
#195863=EDGE_LOOP ( 'NONE', ( #155413, #67678, #151253, #75426 ) ) ;
#195896=VECTOR ( 'NONE', #83585, 1000.000000000000000 ) ;
#195938=CARTESIAN_POINT ( 'NONE',  ( -21.14999999999994174, 74.16448838626247664, -47.52760213295649550 ) ) ;
#195940=ORIENTED_EDGE ( 'NONE', *, *, #127605, .T. ) ;
#195948=DIRECTION ( 'NONE',  ( 0.000000000000000000, 0.000000000000000000, 1.000000000000000000 ) ) ;
#196019=AXIS2_PLACEMENT_3D ( 'NONE', #83271, #145830, #27217 ) ;
#196051=EDGE_CURVE ( 'NONE', #175937, #207750, #79178, .T. ) ;
#196095=EDGE_LOOP ( 'NONE', ( #223716, #4129, #171277, #218194 ) ) ;
#196131=DIRECTION ( 'NONE',  ( -0.000000000000000000, 0.000000000000000000, 1.000000000000000000 ) ) ;
#196137=ORIENTED_EDGE ( 'NONE', *, *, #203888, .F. ) ;
#196178=EDGE_LOOP ( 'NONE', ( #163819, #164929, #153402 ) ) ;
#196180=CARTESIAN_POINT ( 'NONE',  ( 21.15000000000005542, 87.50449464844290048, -37.85861909827351468 ) ) ;
#196208=ORIENTED_EDGE ( 'NONE', *, *, #118898, .F. ) ;
#196234=TOROIDAL_SURFACE ( 'NONE', #158856, 0.2000000000000000111, 0.1000000000000000056 ) ;
#196251=DIRECTION ( 'NONE',  ( 0.000000000000000000, 0.9910827722268042983, 0.1332476588733639278 ) ) ;
#196253=EDGE_CURVE ( 'NONE', #195803, #51994, #243399, .T. ) ;
#196274=DIRECTION ( 'NONE',  ( 1.000000000000000000, 0.000000000000000000, 0.000000000000000000 ) ) ;
#196305=VERTEX_POINT ( 'NONE', #170338 ) ;
#196330=ORIENTED_EDGE ( 'NONE', *, *, #189550, .T. ) ;
#196354=CIRCLE ( 'NONE', #158985, 0.09999999999999939493 ) ;
#196390=ORIENTED_EDGE ( 'NONE', *, *, #215345, .T. ) ;
#196396=CARTESIAN_POINT ( 'NONE',  ( -21.14999999999994174, 76.00000000001119815, -3.123107484524795474 ) ) ;
#196411=CARTESIAN_POINT ( 'NONE',  ( 23.40000000000005542, 77.36076146337680370, -43.99645795275012006 ) ) ;
#196414=AXIS2_PLACEMENT_3D ( 'NONE', #8971, #168094, #106776 ) ;
#196420=ORIENTED_EDGE ( 'NONE', *, *, #99728, .T. ) ;
#196559=AXIS2_PLACEMENT_3D ( 'NONE', #57587, #38065, #237535 ) ;
#196627=CARTESIAN_POINT ( 'NONE',  ( -23.49999999999994316, 77.16254490893143725, -44.02310748452479316 ) ) ;
#196634=EDGE_CURVE ( 'NONE', #24890, #26416, #53897, .T. ) ;
#196704=CARTESIAN_POINT ( 'NONE',  ( 23.40000000000005187, 77.83551161375991967, -47.62760213295649692 ) ) ;
#196713=CARTESIAN_POINT ( 'NONE',  ( 23.40000000000005542, 77.83551161375991967, -47.52760213295649550 ) ) ;
#196806=DIRECTION ( 'NONE',  ( 0.000000000000000000, 0.1575546449569757979, -0.9875102702516471709 ) ) ;
#196821=AXIS2_PLACEMENT_3D ( 'NONE', #154746, #80282, #174339 ) ;
#196851=EDGE_CURVE ( 'NONE', #82762, #184062, #76483, .T. ) ;
#196878=CARTESIAN_POINT ( 'NONE',  ( -23.39999999999994529, 87.50449464844290048, -34.18759587077607165 ) ) ;
#196911=AXIS2_PLACEMENT_3D ( 'NONE', #79217, #117092, #158807 ) ;
#196928=LINE ( 'NONE', #256852, #172684 ) ;
#196966=CARTESIAN_POINT ( 'NONE',  ( -21.14999999999994174, 64.25000000001119815, -51.02310748452479316 ) ) ;
#196972=CIRCLE ( 'NONE', #84501, 0.1000000000000028644 ) ;
#196975=EDGE_LOOP ( 'NONE', ( #148931, #7463, #7377, #200284 ) ) ;
#197029=ORIENTED_EDGE ( 'NONE', *, *, #242143, .F. ) ;
#197070=CARTESIAN_POINT ( 'NONE',  ( 20.95000000000005258, 67.65000000001118963, -25.49719488170504533 ) ) ;
#197085=CARTESIAN_POINT ( 'NONE',  ( -23.39999999999994529, 76.00000000001119815, -36.02310748452479316 ) ) ;
#197091=AXIS2_PLACEMENT_3D ( 'NONE', #205690, #213391, #212134 ) ;
#197245=ORIENTED_EDGE ( 'NONE', *, *, #219553, .F. ) ;
#197253=ORIENTED_EDGE ( 'NONE', *, *, #78514, .F. ) ;
#197281=ORIENTED_EDGE ( 'NONE', *, *, #104142, .F. ) ;
#197290=CARTESIAN_POINT ( 'NONE',  ( -5.999999999999938716, 64.35000000001120668, -22.12310748452479103 ) ) ;
#197321=ORIENTED_EDGE ( 'NONE', *, *, #112028, .F. ) ;
#197326=ADVANCED_FACE ( 'NONE', ( #79546 ), #159135, .T. ) ;
#197360=ORIENTED_EDGE ( 'NONE', *, *, #112274, .F. ) ;
#197467=CARTESIAN_POINT ( 'NONE',  ( 21.05000000000005400, 65.35000000001120668, -4.623107484524796362 ) ) ;
#197471=LINE ( 'NONE', #34580, #66251 ) ;
#197515=EDGE_CURVE ( 'NONE', #65513, #115551, #58376, .T. ) ;
#197543=VERTEX_POINT ( 'NONE', #255269 ) ;
#197575=DIRECTION ( 'NONE',  ( 0.000000000000000000, 0.000000000000000000, 1.000000000000000000 ) ) ;
#197603=CARTESIAN_POINT ( 'NONE',  ( 23.40000000000005542, 83.90000000001120384, -34.86056257560453986 ) ) ;
#197682=FACE_OUTER_BOUND ( 'NONE', #97298, .T. ) ;
#197695=EDGE_CURVE ( 'NONE', #122992, #10605, #143497, .T. ) ;
#197713=EDGE_CURVE ( 'NONE', #148669, #131851, #122682, .T. ) ;
#197755=FACE_OUTER_BOUND ( 'NONE', #216921, .T. ) ;
#197759=EDGE_LOOP ( 'NONE', ( #14572, #73200, #92865, #36637, #106914, #92505, #80305, #143683, #51189, #3099, #169835, #199615, #161561, #59791, #24523, #88964 ) ) ;
#197803=VECTOR ( 'NONE', #151576, 1000.000000000000000 ) ;
#197807=CARTESIAN_POINT ( 'NONE',  ( 13.40000000000005898, 67.75000000001118394, -18.42310748452479530 ) ) ;
#197820=DIRECTION ( 'NONE',  ( -1.000000000000000000, 0.000000000000000000, 0.000000000000000000 ) ) ;
#197824=EDGE_CURVE ( 'NONE', #58156, #10047, #52087, .T. ) ;
#197867=( GEOMETRIC_REPRESENTATION_CONTEXT ( 3 ) GLOBAL_UNCERTAINTY_ASSIGNED_CONTEXT ( ( #107780 ) ) GLOBAL_UNIT_ASSIGNED_CONTEXT ( ( #44766, #188127, #169900 ) ) REPRESENTATION_CONTEXT ( 'NONE', 'WORKASPACE' ) );
#197868=CARTESIAN_POINT ( 'NONE',  ( -23.49999999999994316, 64.25000000001119815, -36.02310748452479316 ) ) ;
#197879=VERTEX_POINT ( 'NONE', #138567 ) ;
#197891=FACE_OUTER_BOUND ( 'NONE', #98960, .T. ) ;
#197968=CARTESIAN_POINT ( 'NONE',  ( 6.100000000000049383, 64.35000000001120668, -51.02310748452480738 ) ) ;
#198019=LINE ( 'NONE', #79349, #152756 ) ;
#198037=FACE_OUTER_BOUND ( 'NONE', #130192, .T. ) ;
#198042=PLANE ( 'NONE',  #212222 ) ;
#198060=ORIENTED_EDGE ( 'NONE', *, *, #208286, .T. ) ;
#198151=PRODUCT_CONTEXT ( 'NONE', #212334, 'mechanical' ) ;
#198167=CARTESIAN_POINT ( 'NONE',  ( -21.14999999999994174, 74.16448838626247664, -47.52760213295649550 ) ) ;
#198188=ADVANCED_FACE ( 'NONE', ( #187582 ), #108027, .F. ) ;
#198235=AXIS2_PLACEMENT_3D ( 'NONE', #185967, #184673, #243365 ) ;
#198246=EDGE_CURVE ( 'NONE', #190938, #68335, #122461, .T. ) ;
#198272=DIRECTION ( 'NONE',  ( 0.000000000000000000, 0.000000000000000000, 1.000000000000000000 ) ) ;
#198424=DIRECTION ( 'NONE',  ( 1.000000000000000000, -0.000000000000000000, -0.000000000000000000 ) ) ;
#198482=EDGE_LOOP ( 'NONE', ( #184960, #22195, #210766, #147759 ) ) ;
#198506=ADVANCED_FACE ( 'NONE', ( #184997 ), #160474, .T. ) ;
#198526=DIRECTION ( 'NONE',  ( -1.000000000000000000, -0.000000000000000000, -0.000000000000000000 ) ) ;
#198579=CARTESIAN_POINT ( 'NONE',  ( -11.59999999999994458, 67.75000000001118394, -25.06452884076210452 ) ) ;
#198627=ORIENTED_EDGE ( 'NONE', *, *, #193369, .F. ) ;
#198636=ORIENTED_EDGE ( 'NONE', *, *, #115178, .F. ) ;
#198660=ORIENTED_EDGE ( 'NONE', *, *, #51549, .F. ) ;
#198668=DIRECTION ( 'NONE',  ( 0.000000000000000000, 0.000000000000000000, -1.000000000000000000 ) ) ;
#198732=CARTESIAN_POINT ( 'NONE',  ( -21.14999999999994174, 76.00000000001119815, -40.17310748452479174 ) ) ;
#198791=FACE_OUTER_BOUND ( 'NONE', #171868, .T. ) ;
#198800=CARTESIAN_POINT ( 'NONE',  ( -21.04999999999994387, 64.25000000001119815, -6.123107484524794586 ) ) ;
#198851=ORIENTED_EDGE ( 'NONE', *, *, #168166, .T. ) ;
#198891=EDGE_CURVE ( 'NONE', #107789, #73651, #10234, .T. ) ;
#198921=DIRECTION ( 'NONE',  ( 0.000000000000000000, -0.1332476588733448597, -0.9910827722268067408 ) ) ;
#198954=EDGE_LOOP ( 'NONE', ( #189270, #23866, #175601, #71812 ) ) ;
#198999=LINE ( 'NONE', #79019, #221768 ) ;
#199075=CARTESIAN_POINT ( 'NONE',  ( -23.39999999999994529, 74.94272479589878344, -8.023107484524793165 ) ) ;
#199126=CARTESIAN_POINT ( 'NONE',  ( -23.39999999999994529, 64.35000000001120668, -3.023107484524792277 ) ) ;
#199135=CARTESIAN_POINT ( 'NONE',  ( 21.15000000000005542, 64.35000000001120668, -3.123107484524795474 ) ) ;
#199168=AXIS2_PLACEMENT_3D ( 'NONE', #60240, #138475, #61540 ) ;
#199222=ORIENTED_EDGE ( 'NONE', *, *, #164989, .T. ) ;
#199261=CARTESIAN_POINT ( 'NONE',  ( -21.14999999999994174, 64.25000000001119815, -51.02310748452479316 ) ) ;
#199299=DIRECTION ( 'NONE',  ( -3.469446951953515108E-14, 4.163336342344217877E-13, -1.000000000000000000 ) ) ;
#199304=CIRCLE ( 'NONE', #61742, 0.09999999999999939493 ) ;
#199347=ORIENTED_EDGE ( 'NONE', *, *, #138717, .F. ) ;
#199352=DIRECTION ( 'NONE',  ( 0.000000000000000000, 0.000000000000000000, 1.000000000000000000 ) ) ;
#199353=ORIENTED_EDGE ( 'NONE', *, *, #19244, .T. ) ;
#199379=EDGE_LOOP ( 'NONE', ( #50271, #247965, #19854, #157265 ) ) ;
#199391=DIRECTION ( 'NONE',  ( 0.000000000000000000, -1.000000000000000000, 0.000000000000000000 ) ) ;
#199424=DIRECTION ( 'NONE',  ( 0.000000000000000000, 0.000000000000000000, -1.000000000000000000 ) ) ;
#199433=ORIENTED_EDGE ( 'NONE', *, *, #56260, .T. ) ;
#199475=CARTESIAN_POINT ( 'NONE',  ( 20.95000000000005258, 65.15000000001120384, -3.123107484524795474 ) ) ;
#199533=EDGE_CURVE ( 'NONE', #139324, #169843, #188888, .T. ) ;
#199535=CARTESIAN_POINT ( 'NONE',  ( 20.95000000000005258, 64.25000000001119815, -29.92310748452479174 ) ) ;
#199563=CARTESIAN_POINT ( 'NONE',  ( 23.50000000000005684, 87.50449464844290048, -34.18759587077607165 ) ) ;
#199568=CIRCLE ( 'NONE', #87088, 0.1000000000000028644 ) ;
#199609=EDGE_CURVE ( 'NONE', #111962, #26247, #46788, .T. ) ;
#199615=ORIENTED_EDGE ( 'NONE', *, *, #256615, .T. ) ;
#199632=CARTESIAN_POINT ( 'NONE',  ( 20.95000000000005258, 66.15000000001120384, -5.923107484524795296 ) ) ;
#199645=ORIENTED_EDGE ( 'NONE', *, *, #98346, .T. ) ;
#199670=AXIS2_PLACEMENT_3D ( 'NONE', #199135, #242100, #37510 ) ;
#199723=DIRECTION ( 'NONE',  ( 0.000000000000000000, 0.000000000000000000, -1.000000000000000000 ) ) ;
#199748=EDGE_CURVE ( 'NONE', #139130, #82762, #27187, .T. ) ;
#199755=AXIS2_PLACEMENT_3D ( 'NONE', #203563, #224396, #45767 ) ;
#199806=CARTESIAN_POINT ( 'NONE',  ( -5.999999999999938716, 64.65000000001120384, -22.12310748452479103 ) ) ;
#199831=CIRCLE ( 'NONE', #45681, 0.09999999999999530098 ) ;
#199839=EDGE_CURVE ( 'NONE', #239496, #35839, #80446, .T. ) ;
#199882=EDGE_CURVE ( 'NONE', #104351, #21018, #106412, .T. ) ;
#200003=ORIENTED_EDGE ( 'NONE', *, *, #64526, .T. ) ;
#200032=AXIS2_PLACEMENT_3D ( 'NONE', #91150, #52005, #213666 ) ;
#200077=DIRECTION ( 'NONE',  ( 0.000000000000000000, 1.000000000000000000, 0.000000000000000000 ) ) ;
#200096=CARTESIAN_POINT ( 'NONE',  ( -21.04999999999994387, 74.94272479589878344, -8.023107484524793165 ) ) ;
#200117=DIRECTION ( 'NONE',  ( 0.000000000000000000, 1.000000000000000000, 0.000000000000000000 ) ) ;
#200124=EDGE_CURVE ( 'NONE', #222419, #144818, #134994, .T. ) ;
#200176=ORIENTED_EDGE ( 'NONE', *, *, #191514, .F. ) ;
#200185=DIRECTION ( 'NONE',  ( 0.000000000000000000, 0.1332476588733448597, 0.9910827722268067408 ) ) ;
#200250=ORIENTED_EDGE ( 'NONE', *, *, #204974, .F. ) ;
#200284=ORIENTED_EDGE ( 'NONE', *, *, #1262, .F. ) ;
#200332=EDGE_CURVE ( 'NONE', #57819, #84546, #201407, .T. ) ;
#200341=VERTEX_POINT ( 'NONE', #47458 ) ;
#200357=ORIENTED_EDGE ( 'NONE', *, *, #253496, .F. ) ;
#200385=DIRECTION ( 'NONE',  ( 0.000000000000000000, -0.1332476588733448597, 0.9910827722268067408 ) ) ;
#200451=AXIS2_PLACEMENT_3D ( 'NONE', #246986, #48790, #128347 ) ;
#200459=ORIENTED_EDGE ( 'NONE', *, *, #6253, .F. ) ;
#200461=AXIS2_PLACEMENT_3D ( 'NONE', #228114, #89860, #49464 ) ;
#200476=CYLINDRICAL_SURFACE ( 'NONE', #66799, 0.09999999999999850675 ) ;
#200547=DIRECTION ( 'NONE',  ( 1.000000000000000000, 0.000000000000000000, -0.000000000000000000 ) ) ;
#200561=ORIENTED_EDGE ( 'NONE', *, *, #204291, .T. ) ;
#200564=EDGE_CURVE ( 'NONE', #32708, #255703, #140104, .T. ) ;
#200616=CARTESIAN_POINT ( 'NONE',  ( 5.900000000000060751, 64.35000000001120668, -22.12310748452479103 ) ) ;
#200717=ADVANCED_BREP_SHAPE_REPRESENTATION ( '', ( #190377, #2425 ), #197867 ) ;
#200755=DIRECTION ( 'NONE',  ( 0.000000000000000000, -0.7071067811865479058, -0.7071067811865472397 ) ) ;
#200844=AXIS2_PLACEMENT_3D ( 'NONE', #109257, #46717, #68883 ) ;
#200850=CARTESIAN_POINT ( 'NONE',  ( 21.15000000000005542, 73.94408376456904364, -49.16694968567509250 ) ) ;
#200899=EDGE_LOOP ( 'NONE', ( #11786, #88122, #102516, #150790 ) ) ;
#200936=DIRECTION ( 'NONE',  ( 1.000000000000000000, 0.000000000000000000, 0.000000000000000000 ) ) ;
#200986=DIRECTION ( 'NONE',  ( 1.000000000000000000, -0.000000000000000000, -0.000000000000000000 ) ) ;
#201013=EDGE_CURVE ( 'NONE', #228476, #80209, #94637, .T. ) ;
#201024=CARTESIAN_POINT ( 'NONE',  ( 20.95000000000005613, 67.85000000001119247, -3.123107484524795474 ) ) ;
#201051=CARTESIAN_POINT ( 'NONE',  ( 23.50000000000004263, 83.90000000001120384, -34.86056257560453986 ) ) ;
#201062=VERTEX_POINT ( 'NONE', #136307 ) ;
#201094=CARTESIAN_POINT ( 'NONE',  ( 21.05000000000005400, 83.97335046823651794, -34.66234602115918051 ) ) ;
#201097=CARTESIAN_POINT ( 'NONE',  ( -13.39999999999993996, 67.72071067812984779, -24.99381816264344991 ) ) ;
#201190=AXIS2_PLACEMENT_3D ( 'NONE', #160991, #140110, #240519 ) ;
#201223=ORIENTED_EDGE ( 'NONE', *, *, #219553, .T. ) ;
#201324=DIRECTION ( 'NONE',  ( -1.000000000000000000, 0.000000000000000000, 0.000000000000000000 ) ) ;
#201407=LINE ( 'NONE', #3193, #210858 ) ;
#201424=EDGE_LOOP ( 'NONE', ( #187528, #63789, #232163, #243115 ) ) ;
#201466=DIRECTION ( 'NONE',  ( 0.000000000000000000, 0.9910827722268055195, 0.1332476588733540468 ) ) ;
#201487=VERTEX_POINT ( 'NONE', #81181 ) ;
#201543=DIRECTION ( 'NONE',  ( -0.000000000000000000, -0.1332476588733589318, 0.9910827722268049644 ) ) ;
#201661=ORIENTED_EDGE ( 'NONE', *, *, #242816, .F. ) ;
#201686=CARTESIAN_POINT ( 'NONE',  ( 21.15000000000005542, 74.26359666348515987, -47.54092689884382850 ) ) ;
#201688=DIRECTION ( 'NONE',  ( 0.000000000000000000, 0.000000000000000000, 1.000000000000000000 ) ) ;
#201715=DIRECTION ( 'NONE',  ( 1.000000000000000000, -0.000000000000000000, 0.000000000000000000 ) ) ;
#201787=DIRECTION ( 'NONE',  ( 0.000000000000000000, 0.000000000000000000, 1.000000000000000000 ) ) ;
#201800=CIRCLE ( 'NONE', #239409, 0.1000000000000028644 ) ;
#201804=DIRECTION ( 'NONE',  ( 0.000000000000000000, 0.000000000000000000, -1.000000000000000000 ) ) ;
#201808=CARTESIAN_POINT ( 'NONE',  ( 23.40000000000005187, 74.25000000001119815, -47.64205752314703801 ) ) ;
#201822=DIRECTION ( 'NONE',  ( -0.000000000000000000, 0.4856429311786307212, 0.8741572761215384846 ) ) ;
#201849=DIRECTION ( 'NONE',  ( 0.000000000000000000, 0.000000000000000000, -1.000000000000000000 ) ) ;
#201882=DIRECTION ( 'NONE',  ( 0.000000000000000000, 0.000000000000000000, -1.000000000000000000 ) ) ;
#201937=VERTEX_POINT ( 'NONE', #177230 ) ;
#201940=EDGE_CURVE ( 'NONE', #99842, #29322, #7384, .T. ) ;
#201979=EDGE_CURVE ( 'NONE', #81245, #172317, #11891, .T. ) ;
#202013=AXIS2_PLACEMENT_3D ( 'NONE', #212995, #248276, #228732 ) ;
#202017=DIRECTION ( 'NONE',  ( 1.000000000000000000, 0.000000000000000000, 0.000000000000000000 ) ) ;
#202060=CIRCLE ( 'NONE', #131310, 11.65000000000000036 ) ;
#202073=DIRECTION ( 'NONE',  ( 0.000000000000000000, 0.000000000000000000, -1.000000000000000000 ) ) ;
#202074=EDGE_CURVE ( 'NONE', #214650, #50827, #102767, .T. ) ;
#202121=DIRECTION ( 'NONE',  ( 0.000000000000000000, 1.000000000000000000, -1.156482317317873105E-15 ) ) ;
#202212=CYLINDRICAL_SURFACE ( 'NONE', #65526, 0.1000000000000028644 ) ;
#202257=DIRECTION ( 'NONE',  ( 0.000000000000000000, -1.000000000000000000, 0.000000000000000000 ) ) ;
#202267=ORIENTED_EDGE ( 'NONE', *, *, #99980, .T. ) ;
#202314=ORIENTED_EDGE ( 'NONE', *, *, #20749, .F. ) ;
#202331=CARTESIAN_POINT ( 'NONE',  ( 0.9000000000000554223, 63.75000000001118394, -10.02310748452479139 ) ) ;
#202351=DIRECTION ( 'NONE',  ( 0.000000000000000000, 0.000000000000000000, -1.000000000000000000 ) ) ;
#202382=DIRECTION ( 'NONE',  ( 1.000000000000000000, 0.000000000000000000, 0.000000000000000000 ) ) ;
#202440=CIRCLE ( 'NONE', #235737, 0.09999999999999530098 ) ;
#202458=CIRCLE ( 'NONE', #23427, 0.09999999999999635569 ) ;
#202463=DIRECTION ( 'NONE',  ( 0.000000000000000000, 0.000000000000000000, -1.000000000000000000 ) ) ;
#202492=VERTEX_POINT ( 'NONE', #167612 ) ;
#202500=ORIENTED_EDGE ( 'NONE', *, *, #88840, .F. ) ;
#202502=EDGE_LOOP ( 'NONE', ( #5527, #188323, #188754, #10448 ) ) ;
#202518=AXIS2_PLACEMENT_3D ( 'NONE', #136405, #192569, #75211 ) ;
#202553=VERTEX_POINT ( 'NONE', #20084 ) ;
#202584=CARTESIAN_POINT ( 'NONE',  ( 23.40000000000005187, 76.00000000001119815, -36.02310748452479316 ) ) ;
#202638=CARTESIAN_POINT ( 'NONE',  ( -23.49999999999994316, 76.00000000001119815, -36.02310748452479316 ) ) ;
#202639=DIRECTION ( 'NONE',  ( -1.000000000000000000, 0.000000000000000000, 0.000000000000000000 ) ) ;
#202672=CARTESIAN_POINT ( 'NONE',  ( 5.900000000000059863, 64.75000000001119815, -25.92310748452479174 ) ) ;
#202787=DIRECTION ( 'NONE',  ( -0.000000000000000000, 1.000000000000000000, -0.000000000000000000 ) ) ;
#202820=ORIENTED_EDGE ( 'NONE', *, *, #254311, .F. ) ;
#202829=DIRECTION ( 'NONE',  ( -0.000000000000000000, 0.000000000000000000, 1.000000000000000000 ) ) ;
#202846=ORIENTED_EDGE ( 'NONE', *, *, #195755, .F. ) ;
#202888=ORIENTED_EDGE ( 'NONE', *, *, #235000, .F. ) ;
#202897=ORIENTED_EDGE ( 'NONE', *, *, #24505, .F. ) ;
#202916=TOROIDAL_SURFACE ( 'NONE', #227854, 4.150000000000000355, 0.1000000000000000056 ) ;
#202919=LINE ( 'NONE', #122109, #225250 ) ;
#202924=CARTESIAN_POINT ( 'NONE',  ( -23.39999999999994529, 74.16448838626247664, -47.52760213295649550 ) ) ;
#202934=FACE_OUTER_BOUND ( 'NONE', #129651, .T. ) ;
#202943=ORIENTED_EDGE ( 'NONE', *, *, #110636, .T. ) ;
#202991=CARTESIAN_POINT ( 'NONE',  ( 23.40000000000005542, 87.50449464844290048, -37.85861909827351468 ) ) ;
#203018=ADVANCED_FACE ( 'NONE', ( #134560 ), #177600, .T. ) ;
#203090=MECHANICAL_DESIGN_GEOMETRIC_PRESENTATION_REPRESENTATION('',(#136421),#190648);
#203100=CARTESIAN_POINT ( 'NONE',  ( 5.551115123125782702E-14, 64.75000000001119815, -22.12310748452479103 ) ) ;
#203103=AXIS2_PLACEMENT_3D ( 'NONE', #94468, #33262, #34533 ) ;
#203117=VECTOR ( 'NONE', #135514, 1000.000000000000000 ) ;
#203122=ORIENTED_EDGE ( 'NONE', *, *, #210810, .F. ) ;
#203165=ORIENTED_EDGE ( 'NONE', *, *, #68647, .T. ) ;
#203186=CARTESIAN_POINT ( 'NONE',  ( 21.15000000000005187, 76.00000000001119815, -36.02310748452479316 ) ) ;
#203215=DIRECTION ( 'NONE',  ( -1.000000000000000000, 0.000000000000000000, 0.000000000000000000 ) ) ;
#203296=PLANE ( 'NONE',  #5205 ) ;
#203414=DIRECTION ( 'NONE',  ( 0.000000000000000000, -0.1480365673253004333, 0.9889818879709283417 ) ) ;
#203434=EDGE_LOOP ( 'NONE', ( #127220, #254946, #138950, #246498 ) ) ;
#203495=EDGE_LOOP ( 'NONE', ( #7255, #8988, #156070, #246312, #107438, #231574, #6254, #185785, #96662, #48301, #6019, #79533, #23932, #100788, #191637, #223685, #257813, #34473, #252769, #15078, #11704, #121327, #101365 ) ) ;
#203496=VECTOR ( 'NONE', #26548, 1000.000000000000000 ) ;
#203498=AXIS2_PLACEMENT_3D ( 'NONE', #69334, #148873, #228408 ) ;
#203515=CYLINDRICAL_SURFACE ( 'NONE', #181455, 0.1000000000000021844 ) ;
#203523=AXIS2_PLACEMENT_3D ( 'NONE', #86833, #107698, #188521 ) ;
#203537=LINE ( 'NONE', #223087, #107871 ) ;
#203563=CARTESIAN_POINT ( 'NONE',  ( 23.40000000000005187, 64.35000000001120668, -36.02310748452479316 ) ) ;
#203582=DIRECTION ( 'NONE',  ( -1.000000000000000000, -0.000000000000000000, -0.000000000000000000 ) ) ;
#203593=EDGE_CURVE ( 'NONE', #169497, #40979, #8336, .T. ) ;
#203660=DIRECTION ( 'NONE',  ( 0.000000000000000000, 0.000000000000000000, 1.000000000000000000 ) ) ;
#203768=DIRECTION ( 'NONE',  ( 0.000000000000000000, -1.000000000000000000, -0.000000000000000000 ) ) ;
#203780=AXIS2_PLACEMENT_3D ( 'NONE', #186363, #66404, #3861 ) ;
#203851=DIRECTION ( 'NONE',  ( 0.000000000000000000, 0.000000000000000000, 1.000000000000000000 ) ) ;
#203867=AXIS2_PLACEMENT_3D ( 'NONE', #97906, #220472, #43110 ) ;
#203888=EDGE_CURVE ( 'NONE', #121144, #168296, #103481, .T. ) ;
#203894=DIRECTION ( 'NONE',  ( -1.000000000000000000, 0.000000000000000000, -0.000000000000000000 ) ) ;
#203917=DIRECTION ( 'NONE',  ( 1.000000000000000000, 0.000000000000000000, 0.000000000000000000 ) ) ;
#203933=FACE_OUTER_BOUND ( 'NONE', #18690, .T. ) ;
#203941=AXIS2_PLACEMENT_3D ( 'NONE', #252634, #231822, #34928 ) ;
#203991=CIRCLE ( 'NONE', #96213, 2.700000000000001066 ) ;
#204008=DIRECTION ( 'NONE',  ( 0.000000000000000000, 0.1332476588733589318, -0.9910827722268049644 ) ) ;
#204027=ORIENTED_EDGE ( 'NONE', *, *, #117874, .T. ) ;
#204034=VERTEX_POINT ( 'NONE', #178925 ) ;
#204047=EDGE_CURVE ( 'NONE', #179805, #109234, #3842, .T. ) ;
#204094=AXIS2_PLACEMENT_3D ( 'NONE', #171896, #252661, #37497 ) ;
#204100=ADVANCED_FACE ( 'NONE', ( #215440 ), #137187, .T. ) ;
#204129=CARTESIAN_POINT ( 'NONE',  ( 23.40000000000005542, 62.43959356634987046, -37.55748533175129467 ) ) ;
#204178=ADVANCED_FACE ( 'NONE', ( #214165 ), #103180, .T. ) ;
#204213=ORIENTED_EDGE ( 'NONE', *, *, #47424, .T. ) ;
#204278=CARTESIAN_POINT ( 'NONE',  ( 23.50000000000004263, 77.16254490893143725, -43.92310748452479885 ) ) ;
#204291=EDGE_CURVE ( 'NONE', #89464, #179303, #257856, .T. ) ;
#204318=DIRECTION ( 'NONE',  ( 0.000000000000000000, 0.000000000000000000, -1.000000000000000000 ) ) ;
#204320=DIRECTION ( 'NONE',  ( 0.000000000000000000, 0.9910827722268048534, -0.1332476588733589040 ) ) ;
#204340=DIRECTION ( 'NONE',  ( 0.000000000000000000, 1.000000000000000000, -0.000000000000000000 ) ) ;
#204377=CARTESIAN_POINT ( 'NONE',  ( 23.50000000000005684, 77.83551161375993388, -47.52760213295649550 ) ) ;
#204460=AXIS2_PLACEMENT_3D ( 'NONE', #126620, #53175, #245294 ) ;
#204488=FACE_OUTER_BOUND ( 'NONE', #9117, .T. ) ;
#204503=VECTOR ( 'NONE', #248196, 1000.000000000000000 ) ;
#204560=CARTESIAN_POINT ( 'NONE',  ( -20.94999999999994600, 66.15000000001120384, -5.923107484524795296 ) ) ;
#204569=FACE_OUTER_BOUND ( 'NONE', #186192, .T. ) ;
#204597=DIRECTION ( 'NONE',  ( 0.000000000000000000, 0.000000000000000000, 1.000000000000000000 ) ) ;
#204636=DIRECTION ( 'NONE',  ( 0.000000000000000000, 0.1332476588733448597, -0.9910827722268067408 ) ) ;
#204649=ADVANCED_FACE ( 'NONE', ( #122474 ), #174764, .T. ) ;
#204659=EDGE_CURVE ( 'NONE', #40901, #69129, #29193, .T. ) ;
#204709=CARTESIAN_POINT ( 'NONE',  ( 21.05000000000005400, 76.00000000001119815, -36.02310748452479316 ) ) ;
#204770=ORIENTED_EDGE ( 'NONE', *, *, #1769, .F. ) ;
#204817=SPHERICAL_SURFACE ( 'NONE', #164467, 0.1000000000000000056 ) ;
#204819=CARTESIAN_POINT ( 'NONE',  ( 20.95000000000005613, 67.85000000001119247, -25.49719488170504533 ) ) ;
#204872=CARTESIAN_POINT ( 'NONE',  ( 11.60000000000006004, 67.75000000001118394, -16.98168612828748891 ) ) ;
#204906=ORIENTED_EDGE ( 'NONE', *, *, #170169, .F. ) ;
#204910=CIRCLE ( 'NONE', #229867, 0.09999999999999982514 ) ;
#204927=ORIENTED_EDGE ( 'NONE', *, *, #166224, .T. ) ;
#204931=ORIENTED_EDGE ( 'NONE', *, *, #194843, .T. ) ;
#204943=EDGE_CURVE ( 'NONE', #144437, #24890, #195764, .T. ) ;
#204974=EDGE_CURVE ( 'NONE', #12197, #186900, #4191, .T. ) ;
#204993=VECTOR ( 'NONE', #38450, 1000.000000000000000 ) ;
#205002=ORIENTED_EDGE ( 'NONE', *, *, #244093, .F. ) ;
#205039=AXIS2_PLACEMENT_3D ( 'NONE', #44423, #104356, #5251 ) ;
#205045=ORIENTED_EDGE ( 'NONE', *, *, #137418, .T. ) ;
#205049=DIRECTION ( 'NONE',  ( 0.000000000000000000, 0.1480365673253023762, -0.9889818879709281196 ) ) ;
#205065=EDGE_CURVE ( 'NONE', #184662, #197543, #120937, .T. ) ;
#205096=DIRECTION ( 'NONE',  ( 0.000000000000000000, -0.9889818879709260102, -0.1480365673253158931 ) ) ;
#205099=AXIS2_PLACEMENT_3D ( 'NONE', #86764, #45094, #8539 ) ;
#205114=VERTEX_POINT ( 'NONE', #257753 ) ;
#205145=DIRECTION ( 'NONE',  ( 0.000000000000000000, 0.000000000000000000, -1.000000000000000000 ) ) ;
#205195=CYLINDRICAL_SURFACE ( 'NONE', #232191, 0.1000000000000002554 ) ;
#205276=CARTESIAN_POINT ( 'NONE',  ( -23.49999999999994316, 76.00000000001119815, -36.02310748452479316 ) ) ;
#205297=DIRECTION ( 'NONE',  ( 0.000000000000000000, 0.9910827722268055195, -0.1332476588733540468 ) ) ;
#205342=FACE_OUTER_BOUND ( 'NONE', #32508, .T. ) ;
#205352=CARTESIAN_POINT ( 'NONE',  ( 20.95000000000005258, 65.35000000001120668, -4.423107484524790856 ) ) ;
#205358=DIRECTION ( 'NONE',  ( -0.000000000000000000, 1.000000000000000000, -0.000000000000000000 ) ) ;
#205362=DIRECTION ( 'NONE',  ( 0.000000000000000000, -1.000000000000000000, 0.000000000000000000 ) ) ;
#205403=DIRECTION ( 'NONE',  ( 1.000000000000000000, -0.000000000000000000, -0.000000000000000000 ) ) ;
#205434=CARTESIAN_POINT ( 'NONE',  ( -21.04999999999994387, 66.25000000001119815, -4.623107484524796362 ) ) ;
#205481=CARTESIAN_POINT ( 'NONE',  ( 23.40000000000005187, 87.60324567546805952, -34.17184040628037422 ) ) ;
#205492=CARTESIAN_POINT ( 'NONE',  ( 21.15000000000005542, 64.35000000001120668, -30.12310748452479103 ) ) ;
#205499=EDGE_CURVE ( 'NONE', #228476, #60596, #212867, .T. ) ;
#205550=CARTESIAN_POINT ( 'NONE',  ( -23.39999999999994529, 82.74366731733570646, -26.36310895752070138 ) ) ;
#205588=CARTESIAN_POINT ( 'NONE',  ( -5.999999999999938716, 64.35000000001120668, -26.02310748452479316 ) ) ;
#205659=CARTESIAN_POINT ( 'NONE',  ( 21.05000000000005400, 61.72892516158560028, -36.56695479651062186 ) ) ;
#205671=ADVANCED_FACE ( 'NONE', ( #172566 ), #189518, .T. ) ;
#205690=CARTESIAN_POINT ( 'NONE',  ( -5.899999999999938183, 64.65000000001120384, -25.92310748452479174 ) ) ;
#205711=ORIENTED_EDGE ( 'NONE', *, *, #217306, .T. ) ;
#205775=EDGE_CURVE ( 'NONE', #144437, #133820, #96129, .T. ) ;
#205808=CARTESIAN_POINT ( 'NONE',  ( -20.94999999999994245, 67.75000000001118394, -3.023107484524792277 ) ) ;
#205871=DIRECTION ( 'NONE',  ( -0.000000000000000000, -1.000000000000000000, -0.000000000000000000 ) ) ;
#205911=TOROIDAL_SURFACE ( 'NONE', #110057, 4.150000000000000355, 0.1000000000000000056 ) ;
#205966=ORIENTED_EDGE ( 'NONE', *, *, #199882, .T. ) ;
#205981=EDGE_CURVE ( 'NONE', #33613, #50040, #184274, .T. ) ;
#206010=ORIENTED_EDGE ( 'NONE', *, *, #218913, .T. ) ;
#206041=DIRECTION ( 'NONE',  ( -1.284434275755705296E-16, 0.7071067811865471286, 0.7071067811865479058 ) ) ;
#206178=CIRCLE ( 'NONE', #39622, 0.1000000000000002554 ) ;
#206191=AXIS2_PLACEMENT_3D ( 'NONE', #121440, #21048, #96666 ) ;
#206221=ORIENTED_EDGE ( 'NONE', *, *, #120573, .F. ) ;
#206234=CARTESIAN_POINT ( 'NONE',  ( 21.15000000000005187, 64.35000000001120668, -51.02310748452479316 ) ) ;
#206260=CIRCLE ( 'NONE', #81314, 0.1000000000000021844 ) ;
#206268=ADVANCED_FACE ( 'NONE', ( #15731 ), #155246, .F. ) ;
#206276=TOROIDAL_SURFACE ( 'NONE', #81328, 0.2000000000000000111, 0.1000000000000000056 ) ;
#206284=ORIENTED_EDGE ( 'NONE', *, *, #182822, .T. ) ;
#206337=CIRCLE ( 'NONE', #239651, 0.1999999999999987899 ) ;
#206439=ADVANCED_FACE ( 'NONE', ( #214535 ), #228023, .T. ) ;
#206442=EDGE_LOOP ( 'NONE', ( #160760, #237489, #31694, #26757 ) ) ;
#206541=ORIENTED_EDGE ( 'NONE', *, *, #48843, .T. ) ;
#206596=FACE_OUTER_BOUND ( 'NONE', #165290, .T. ) ;
#206627=ORIENTED_EDGE ( 'NONE', *, *, #221486, .T. ) ;
#206633=AXIS2_PLACEMENT_3D ( 'NONE', #11296, #32164, #68703 ) ;
#206636=TOROIDAL_SURFACE ( 'NONE', #81703, 11.65000000000000036, 0.1000000000000000056 ) ;
#206641=AXIS2_PLACEMENT_3D ( 'NONE', #98777, #220053, #242175 ) ;
#206740=LINE ( 'NONE', #5948, #147299 ) ;
#206801=CIRCLE ( 'NONE', #244193, 0.1000000000000028644 ) ;
#206805=EDGE_CURVE ( 'NONE', #96904, #44045, #50840, .T. ) ;
#206839=ORIENTED_EDGE ( 'NONE', *, *, #171534, .F. ) ;
#206903=ORIENTED_EDGE ( 'NONE', *, *, #85416, .T. ) ;
#206904=DIRECTION ( 'NONE',  ( -0.000000000000000000, 0.000000000000000000, -1.000000000000000000 ) ) ;
#206917=AXIS2_PLACEMENT_3D ( 'NONE', #57624, #175071, #74678 ) ;
#206962=DIRECTION ( 'NONE',  ( 1.000000000000000000, -0.000000000000000000, -0.000000000000000000 ) ) ;
#206989=EDGE_CURVE ( 'NONE', #76432, #89464, #64166, .T. ) ;
#207031=CARTESIAN_POINT ( 'NONE',  ( -23.39999999999994529, 74.94272479589878344, -8.023107484524793165 ) ) ;
#207098=ADVANCED_FACE ( 'NONE', ( #211381 ), #34334, .T. ) ;
#207111=DIRECTION ( 'NONE',  ( 1.000000000000000000, 0.000000000000000000, 0.000000000000000000 ) ) ;
#207119=CARTESIAN_POINT ( 'NONE',  ( 20.95000000000005258, 65.25000000001119815, -3.023107484524792277 ) ) ;
#207121=DIRECTION ( 'NONE',  ( 0.000000000000000000, 0.1332476588733448597, 0.9910827722268067408 ) ) ;
#207123=AXIS2_PLACEMENT_3D ( 'NONE', #102020, #162047, #62926 ) ;
#207144=ORIENTED_EDGE ( 'NONE', *, *, #43457, .T. ) ;
#207147=DIRECTION ( 'NONE',  ( -1.000000000000000000, -0.000000000000000000, -0.000000000000000000 ) ) ;
#207179=EDGE_CURVE ( 'NONE', #139562, #62001, #37894, .T. ) ;
#207247=AXIS2_PLACEMENT_3D ( 'NONE', #86517, #85228, #47407 ) ;
#207300=ORIENTED_EDGE ( 'NONE', *, *, #182822, .F. ) ;
#207312=LINE ( 'NONE', #169493, #154213 ) ;
#207347=EDGE_LOOP ( 'NONE', ( #111842, #171465, #115044, #82223 ) ) ;
#207391=ORIENTED_EDGE ( 'NONE', *, *, #203593, .T. ) ;
#207479=CARTESIAN_POINT ( 'NONE',  ( 21.05000000000003979, 74.83745509109094485, -43.92310748452479885 ) ) ;
#207517=AXIS2_PLACEMENT_3D ( 'NONE', #200616, #101460, #127495 ) ;
#207525=CARTESIAN_POINT ( 'NONE',  ( 23.40000000000005542, 87.50449464844290048, -34.18759587077607165 ) ) ;
#207579=CIRCLE ( 'NONE', #186730, 0.09999999999999939493 ) ;
#207608=AXIS2_PLACEMENT_3D ( 'NONE', #182494, #165492, #101609 ) ;
#207653=CARTESIAN_POINT ( 'NONE',  ( 5.551115123125782702E-14, 64.35000000001120668, -3.023107484524792277 ) ) ;
#207662=ORIENTED_EDGE ( 'NONE', *, *, #15219, .F. ) ;
#207731=DIRECTION ( 'NONE',  ( 0.000000000000000000, 0.000000000000000000, -1.000000000000000000 ) ) ;
#207734=EDGE_CURVE ( 'NONE', #144818, #97476, #150781, .T. ) ;
#207746=DIRECTION ( 'NONE',  ( 2.889348024582214003E-16, -0.1332476588733650935, -0.9910827722268042983 ) ) ;
#207750=VERTEX_POINT ( 'NONE', #92084 ) ;
#207779=ORIENTED_EDGE ( 'NONE', *, *, #78503, .F. ) ;
#207810=FACE_OUTER_BOUND ( 'NONE', #233795, .T. ) ;
#207814=DIRECTION ( 'NONE',  ( -0.000000000000000000, 0.1332476588733589318, 0.9910827722268049644 ) ) ;
#207913=EDGE_CURVE ( 'NONE', #90293, #113629, #184676, .T. ) ;
#207955=SPHERICAL_SURFACE ( 'NONE', #210978, 0.1000000000000000056 ) ;
#208030=DIRECTION ( 'NONE',  ( -1.000000000000000000, 0.000000000000000000, 0.000000000000000000 ) ) ;
#208102=EDGE_CURVE ( 'NONE', #187156, #135372, #13811, .T. ) ;
#208188=FACE_OUTER_BOUND ( 'NONE', #154219, .T. ) ;
#208237=CARTESIAN_POINT ( 'NONE',  ( -0.8999999999999435119, 66.35000000001119247, -12.62310748452479281 ) ) ;
#208286=EDGE_CURVE ( 'NONE', #86047, #213499, #130579, .T. ) ;
#208331=DIRECTION ( 'NONE',  ( 1.000000000000000000, -0.000000000000000000, -0.000000000000000000 ) ) ;
#208363=DIRECTION ( 'NONE',  ( 1.000000000000000000, 0.000000000000000000, 0.000000000000000000 ) ) ;
#208394=CIRCLE ( 'NONE', #16843, 0.1999999999999987899 ) ;
#208447=EDGE_LOOP ( 'NONE', ( #9633, #92696, #237526, #31370 ) ) ;
#208465=LINE ( 'NONE', #128911, #48950 ) ;
#208471=ADVANCED_FACE ( 'NONE', ( #23060 ), #59551, .T. ) ;
#208544=CARTESIAN_POINT ( 'NONE',  ( -23.39999999999994529, 77.26165318615413469, -44.00978271863746016 ) ) ;
#208639=DIRECTION ( 'NONE',  ( -1.000000000000000000, -0.000000000000000000, 0.000000000000000000 ) ) ;
#208735=FACE_OUTER_BOUND ( 'NONE', #51528, .T. ) ;
#208754=DIRECTION ( 'NONE',  ( 1.000000000000000000, -0.000000000000000000, -0.000000000000000000 ) ) ;
#208814=ORIENTED_EDGE ( 'NONE', *, *, #235454, .F. ) ;
#208820=EDGE_CURVE ( 'NONE', #154033, #210105, #194232, .T. ) ;
#208955=DIRECTION ( 'NONE',  ( 0.000000000000000000, -0.1332476588733589040, 0.9910827722268048534 ) ) ;
#208975=CARTESIAN_POINT ( 'NONE',  ( -11.59999999999994458, 67.75000000001118394, -21.02310748452479316 ) ) ;
#209000=CARTESIAN_POINT ( 'NONE',  ( -5.899999999999938183, 64.65000000001120384, -25.92310748452479174 ) ) ;
#209037=CARTESIAN_POINT ( 'NONE',  ( -23.39999999999994529, 64.35000000001120668, -3.123107484524795474 ) ) ;
#209060=CARTESIAN_POINT ( 'NONE',  ( -23.39999999999994529, 83.97335046823651794, -37.38386894789040582 ) ) ;
#209063=ORIENTED_EDGE ( 'NONE', *, *, #29093, .F. ) ;
#209121=CARTESIAN_POINT ( 'NONE',  ( -5.899999999999938183, 64.35000000001120668, -25.92310748452479174 ) ) ;
#209133=VERTEX_POINT ( 'NONE', #135183 ) ;
#209134=DIRECTION ( 'NONE',  ( -1.000000000000000000, 0.000000000000000000, 0.000000000000000000 ) ) ;
#209142=DIRECTION ( 'NONE',  ( 1.000000000000000000, -0.000000000000000000, -0.000000000000000000 ) ) ;
#209335=AXIS2_PLACEMENT_3D ( 'NONE', #146672, #29369, #68462 ) ;
#209362=AXIS2_PLACEMENT_3D ( 'NONE', #22228, #65, #198272 ) ;
#209385=DIRECTION ( 'NONE',  ( -0.000000000000000000, 1.000000000000000000, -0.000000000000000000 ) ) ;
#209453=DIRECTION ( 'NONE',  ( -1.690361071372200435E-14, 0.1332476588733650935, -0.9910827722268042983 ) ) ;
#209501=FACE_OUTER_BOUND ( 'NONE', #176356, .T. ) ;
#209581=DIRECTION ( 'NONE',  ( 0.000000000000000000, 1.000000000000000000, 0.000000000000000000 ) ) ;
#209590=ORIENTED_EDGE ( 'NONE', *, *, #73536, .F. ) ;
#209623=ORIENTED_EDGE ( 'NONE', *, *, #161700, .T. ) ;
#209636=AXIS2_PLACEMENT_3D ( 'NONE', #220120, #200547, #63603 ) ;
#209667=CARTESIAN_POINT ( 'NONE',  ( 23.50000000000005684, 82.72707916847673459, -26.51159310135756897 ) ) ;
#209679=DIRECTION ( 'NONE',  ( 0.000000000000000000, 0.1332476588733589040, -0.9910827722268048534 ) ) ;
#209683=EDGE_CURVE ( 'NONE', #228476, #238440, #234931, .T. ) ;
#209728=AXIS2_PLACEMENT_3D ( 'NONE', #215138, #37809, #36533 ) ;
#209732=CARTESIAN_POINT ( 'NONE',  ( 21.05000000000005400, 83.80000000001119531, -34.86056257560453986 ) ) ;
#209750=SPHERICAL_SURFACE ( 'NONE', #58592, 0.1000000000000000056 ) ;
#209832=VECTOR ( 'NONE', #110745, 1000.000000000000000 ) ;
#209853=ORIENTED_EDGE ( 'NONE', *, *, #217050, .F. ) ;
#209872=DIRECTION ( 'NONE',  ( 0.000000000000000000, 1.000000000000000000, -8.673617379884042375E-16 ) ) ;
#209873=ORIENTED_EDGE ( 'NONE', *, *, #85416, .F. ) ;
#209906=EDGE_CURVE ( 'NONE', #42311, #184620, #80780, .T. ) ;
#209965=ORIENTED_EDGE ( 'NONE', *, *, #35005, .T. ) ;
#210105=VERTEX_POINT ( 'NONE', #83255 ) ;
#210121=VECTOR ( 'NONE', #255391, 1000.000000000000114 ) ;
#210128=CYLINDRICAL_SURFACE ( 'NONE', #94032, 0.1000000000000028644 ) ;
#210191=ORIENTED_EDGE ( 'NONE', *, *, #207734, .T. ) ;
#210203=EDGE_CURVE ( 'NONE', #61669, #134771, #66298, .T. ) ;
#210293=DIRECTION ( 'NONE',  ( 0.000000000000000000, -0.000000000000000000, 1.000000000000000000 ) ) ;
#210359=ORIENTED_EDGE ( 'NONE', *, *, #42886, .F. ) ;
#210422=EDGE_LOOP ( 'NONE', ( #161937, #210359, #112500, #180085 ) ) ;
#210435=ORIENTED_EDGE ( 'NONE', *, *, #4449, .T. ) ;
#210527=EDGE_LOOP ( 'NONE', ( #231496, #65477, #225283, #131131 ) ) ;
#210531=ORIENTED_EDGE ( 'NONE', *, *, #185293, .T. ) ;
#210574=VERTEX_POINT ( 'NONE', #148089 ) ;
#210591=ORIENTED_EDGE ( 'NONE', *, *, #195755, .T. ) ;
#210711=ORIENTED_EDGE ( 'NONE', *, *, #83809, .T. ) ;
#210730=AXIS2_PLACEMENT_3D ( 'NONE', #80821, #142091, #118707 ) ;
#210736=CARTESIAN_POINT ( 'NONE',  ( 23.40000000000005187, 76.00000000001119815, -36.02310748452479316 ) ) ;
#210766=ORIENTED_EDGE ( 'NONE', *, *, #196851, .F. ) ;
#210768=ORIENTED_EDGE ( 'NONE', *, *, #182245, .T. ) ;
#210784=VERTEX_POINT ( 'NONE', #197467 ) ;
#210790=DIRECTION ( 'NONE',  ( 0.000000000000000000, 0.000000000000000000, -1.000000000000000000 ) ) ;
#210810=EDGE_CURVE ( 'NONE', #210784, #230912, #60483, .T. ) ;
#210845=DIRECTION ( 'NONE',  ( -1.000000000000000000, 0.000000000000000000, 0.000000000000000000 ) ) ;
#210856=ORIENTED_EDGE ( 'NONE', *, *, #146774, .F. ) ;
#210858=VECTOR ( 'NONE', #196274, 1000.000000000000000 ) ;
#210869=ORIENTED_EDGE ( 'NONE', *, *, #64847, .F. ) ;
#210873=FACE_OUTER_BOUND ( 'NONE', #56492, .T. ) ;
#210880=DIRECTION ( 'NONE',  ( 0.000000000000000000, 0.000000000000000000, -1.000000000000000000 ) ) ;
#210891=DIRECTION ( 'NONE',  ( 0.000000000000000000, 0.000000000000000000, -1.000000000000000000 ) ) ;
#210897=CARTESIAN_POINT ( 'NONE',  ( -23.39999999999994529, 87.60324567546805952, -34.17184040628037422 ) ) ;
#210930=CARTESIAN_POINT ( 'NONE',  ( -23.49999999999994316, 82.78482233730476025, -26.42994920107286916 ) ) ;
#210977=DIRECTION ( 'NONE',  ( 1.000000000000000000, 0.000000000000000000, 0.000000000000000000 ) ) ;
#210978=AXIS2_PLACEMENT_3D ( 'NONE', #69723, #172712, #29335 ) ;
#211077=AXIS2_PLACEMENT_3D ( 'NONE', #202672, #200117, #142686 ) ;
#211082=TOROIDAL_SURFACE ( 'NONE', #102907, 0.2000000000000000111, 0.1000000000000000056 ) ;
#211118=LINE ( 'NONE', #147287, #105236 ) ;
#211140=VERTEX_POINT ( 'NONE', #95500 ) ;
#211143=ORIENTED_EDGE ( 'NONE', *, *, #17389, .F. ) ;
#211178=CARTESIAN_POINT ( 'NONE',  ( -21.04999999999994387, 67.75000000001118394, -5.923107484524791744 ) ) ;
#211183=VERTEX_POINT ( 'NONE', #10224 ) ;
#211243=ORIENTED_EDGE ( 'NONE', *, *, #223332, .F. ) ;
#211269=AXIS2_PLACEMENT_3D ( 'NONE', #255878, #17333, #35639 ) ;
#211289=VECTOR ( 'NONE', #205358, 1000.000000000000000 ) ;
#211329=DIRECTION ( 'NONE',  ( 0.000000000000000000, 0.000000000000000000, -1.000000000000000000 ) ) ;
#211381=FACE_OUTER_BOUND ( 'NONE', #17729, .T. ) ;
#211382=DIRECTION ( 'NONE',  ( 0.000000000000000000, 0.000000000000000000, -1.000000000000000000 ) ) ;
#211417=CARTESIAN_POINT ( 'NONE',  ( 21.15000000000005187, 79.88763423575340994, -7.282924647898262549 ) ) ;
#211438=ORIENTED_EDGE ( 'NONE', *, *, #164619, .T. ) ;
#211446=VERTEX_POINT ( 'NONE', #222498 ) ;
#211462=VERTEX_POINT ( 'NONE', #160010 ) ;
#211522=LINE ( 'NONE', #12057, #197803 ) ;
#211537=ADVANCED_FACE ( 'NONE', ( #20495 ), #123429, .T. ) ;
#211566=CARTESIAN_POINT ( 'NONE',  ( -23.39999999999994529, 77.16254490893143725, -44.02310748452479316 ) ) ;
#211576=CARTESIAN_POINT ( 'NONE',  ( -23.39999999999994529, 74.94272479589878344, -3.023107484524792277 ) ) ;
#211652=CIRCLE ( 'NONE', #99178, 4.049999999999998046 ) ;
#211771=LINE ( 'NONE', #112668, #105468 ) ;
#211803=CIRCLE ( 'NONE', #186686, 0.1000000000000032391 ) ;
#211889=CARTESIAN_POINT ( 'NONE',  ( -5.899999999999938183, 64.65000000001120384, -26.02310748452479316 ) ) ;
#211896=CARTESIAN_POINT ( 'NONE',  ( -23.49999999999994316, 74.25000000001119815, -47.64205752314703801 ) ) ;
#211955=CYLINDRICAL_SURFACE ( 'NONE', #120352, 2.599999999999998312 ) ;
#212006=DIRECTION ( 'NONE',  ( 0.000000000000000000, 1.000000000000000000, 0.000000000000000000 ) ) ;
#212113=FACE_OUTER_BOUND ( 'NONE', #86174, .T. ) ;
#212134=DIRECTION ( 'NONE',  ( 1.000000000000000000, 0.000000000000000000, 0.000000000000000000 ) ) ;
#212153=EDGE_CURVE ( 'NONE', #183226, #141859, #61238, .T. ) ;
#212155=ORIENTED_EDGE ( 'NONE', *, *, #255338, .T. ) ;
#212166=ORIENTED_EDGE ( 'NONE', *, *, #243225, .T. ) ;
#212191=FACE_OUTER_BOUND ( 'NONE', #125700, .T. ) ;
#212193=ADVANCED_FACE ( 'NONE', ( #49559 ), #225595, .F. ) ;
#212197=FACE_OUTER_BOUND ( 'NONE', #180242, .T. ) ;
#212222=AXIS2_PLACEMENT_3D ( 'NONE', #19424, #216323, #199352 ) ;
#212322=VECTOR ( 'NONE', #28486, 1000.000000000000000 ) ;
#212334=APPLICATION_CONTEXT ( 'automotive_design' ) ;
#212439=VECTOR ( 'NONE', #230852, 1000.000000000000000 ) ;
#212445=DIRECTION ( 'NONE',  ( 0.000000000000000000, 0.9875102702516490583, 0.1575546449569643070 ) ) ;
#212487=CARTESIAN_POINT ( 'NONE',  ( 23.50000000000005684, 85.84984265665381997, -47.78991727088349251 ) ) ;
#212514=EDGE_CURVE ( 'NONE', #183226, #10605, #227747, .T. ) ;
#212558=CARTESIAN_POINT ( 'NONE',  ( 6.000000000000060396, 64.65000000001120384, -26.02310748452479316 ) ) ;
#212611=DIRECTION ( 'NONE',  ( 0.000000000000000000, 0.9875102702516471709, 0.1575546449569757979 ) ) ;
#212656=DIRECTION ( 'NONE',  ( 1.000000000000000000, 0.000000000000000000, 0.000000000000000000 ) ) ;
#212719=DIRECTION ( 'NONE',  ( -1.000000000000000000, 0.000000000000000000, 0.000000000000000000 ) ) ;
#212790=EDGE_LOOP ( 'NONE', ( #71672, #226198, #19257, #225304 ) ) ;
#212830=ORIENTED_EDGE ( 'NONE', *, *, #26990, .F. ) ;
#212867=CIRCLE ( 'NONE', #87755, 0.09999999999999939493 ) ;
#212995=CARTESIAN_POINT ( 'NONE',  ( -20.94999999999994600, 65.19115966511134275, -29.92310748452479174 ) ) ;
#213005=EDGE_CURVE ( 'NONE', #202492, #211140, #228750, .T. ) ;
#213007=ADVANCED_FACE ( 'NONE', ( #107494 ), #187064, .F. ) ;
#213046=DIRECTION ( 'NONE',  ( 1.000000000000000000, 0.000000000000000000, -0.000000000000000000 ) ) ;
#213060=DIRECTION ( 'NONE',  ( 0.000000000000000000, 0.000000000000000000, -1.000000000000000000 ) ) ;
#213061=FACE_OUTER_BOUND ( 'NONE', #223887, .T. ) ;
#213070=PLANE ( 'NONE',  #26363 ) ;
#213075=LINE ( 'NONE', #113971, #62748 ) ;
#213263=AXIS2_PLACEMENT_3D ( 'NONE', #65975, #235939, #183366 ) ;
#213391=DIRECTION ( 'NONE',  ( 0.000000000000000000, -0.000000000000000000, 1.000000000000000000 ) ) ;
#213443=VECTOR ( 'NONE', #192652, 1000.000000000000000 ) ;
#213499=VERTEX_POINT ( 'NONE', #156640 ) ;
#213501=AXIS2_PLACEMENT_3D ( 'NONE', #126657, #104496, #180229 ) ;
#213513=LINE ( 'NONE', #191432, #220523 ) ;
#213569=CIRCLE ( 'NONE', #246704, 0.1000000000000028644 ) ;
#213591=AXIS2_PLACEMENT_3D ( 'NONE', #44774, #147730, #48615 ) ;
#213623=DIRECTION ( 'NONE',  ( 0.000000000000000000, 0.000000000000000000, 1.000000000000000000 ) ) ;
#213665=EDGE_LOOP ( 'NONE', ( #30760, #164891, #165503, #190167 ) ) ;
#213666=DIRECTION ( 'NONE',  ( 0.000000000000000000, 0.000000000000000000, 1.000000000000000000 ) ) ;
#213756=EDGE_CURVE ( 'NONE', #111921, #108159, #36879, .T. ) ;
#213854=CARTESIAN_POINT ( 'NONE',  ( -0.8999999999999438449, 67.65000000001120384, -14.06452884076210275 ) ) ;
#213899=DIRECTION ( 'NONE',  ( -0.000000000000000000, 0.4856429311786307768, 0.8741572761215384846 ) ) ;
#213974=AXIS2_PLACEMENT_3D ( 'NONE', #116182, #155325, #13230 ) ;
#214031=EDGE_LOOP ( 'NONE', ( #159162, #189533, #116764, #8423 ) ) ;
#214035=EDGE_LOOP ( 'NONE', ( #125230, #198060, #86917, #231961 ) ) ;
#214069=ORIENTED_EDGE ( 'NONE', *, *, #21887, .F. ) ;
#214165=FACE_OUTER_BOUND ( 'NONE', #138738, .T. ) ;
#214193=ORIENTED_EDGE ( 'NONE', *, *, #207913, .T. ) ;
#214215=DIRECTION ( 'NONE',  ( -0.000000000000000000, 1.000000000000000000, -0.000000000000000000 ) ) ;
#214230=CARTESIAN_POINT ( 'NONE',  ( 21.15000000000005542, 85.52235250936195143, -34.45408804175119144 ) ) ;
#214257=DIRECTION ( 'NONE',  ( 0.000000000000000000, 0.000000000000000000, 1.000000000000000000 ) ) ;
#214264=DIRECTION ( 'NONE',  ( 0.000000000000000000, -0.1332476588733448597, -0.9910827722268067408 ) ) ;
#214343=CIRCLE ( 'NONE', #101885, 0.1000000000000028644 ) ;
#214532=ORIENTED_EDGE ( 'NONE', *, *, #163051, .F. ) ;
#214535=FACE_OUTER_BOUND ( 'NONE', #45566, .T. ) ;
#214577=DIRECTION ( 'NONE',  ( 1.000000000000000000, 0.000000000000000000, 0.000000000000000000 ) ) ;
#214578=ADVANCED_FACE ( 'NONE', ( #52379 ), #71973, .F. ) ;
#214588=DIRECTION ( 'NONE',  ( 0.000000000000000000, -1.000000000000000000, 8.673617379884043361E-16 ) ) ;
#214596=DIRECTION ( 'NONE',  ( -0.000000000000000000, 0.9910827722268048534, 0.1332476588733589040 ) ) ;
#214617=CARTESIAN_POINT ( 'NONE',  ( -23.49999999999994316, 76.00000000001119815, -36.02310748452479316 ) ) ;
#214633=ORIENTED_EDGE ( 'NONE', *, *, #247672, .F. ) ;
#214650=VERTEX_POINT ( 'NONE', #116243 ) ;
#214676=EDGE_CURVE ( 'NONE', #153832, #134771, #82569, .T. ) ;
#214682=DIRECTION ( 'NONE',  ( -1.927189404645529861E-14, 0.9875102702516478370, -0.1575546449569727725 ) ) ;
#214727=CARTESIAN_POINT ( 'NONE',  ( -23.39999999999994529, 77.25000000001119815, -43.92310748452479885 ) ) ;
#214755=EDGE_CURVE ( 'NONE', #26051, #114106, #211803, .T. ) ;
#214886=EDGE_LOOP ( 'NONE', ( #134006, #38317, #164362, #137936 ) ) ;
#214901=EDGE_CURVE ( 'NONE', #151679, #121144, #3486, .T. ) ;
#214924=AXIS2_PLACEMENT_3D ( 'NONE', #111817, #208363, #190064 ) ;
#214942=CARTESIAN_POINT ( 'NONE',  ( -21.14999999999994174, 64.35000000001120668, -51.02310748452479316 ) ) ;
#214964=DIRECTION ( 'NONE',  ( 0.000000000000000000, 0.000000000000000000, 1.000000000000000000 ) ) ;
#215019=EDGE_CURVE ( 'NONE', #61669, #153040, #103616, .T. ) ;
#215023=LINE ( 'NONE', #76794, #114691 ) ;
#215027=ORIENTED_EDGE ( 'NONE', *, *, #162810, .T. ) ;
#215036=CARTESIAN_POINT ( 'NONE',  ( 23.40000000000005542, 83.97335046823651794, -37.38386894789040582 ) ) ;
#215089=AXIS2_PLACEMENT_3D ( 'NONE', #121842, #179261, #3143 ) ;
#215108=DIRECTION ( 'NONE',  ( -4.336808689942017736E-16, 0.000000000000000000, -1.000000000000000000 ) ) ;
#215138=CARTESIAN_POINT ( 'NONE',  ( -21.14999999999994174, 82.84256550613280012, -26.34830530078816935 ) ) ;
#215142=VERTEX_POINT ( 'NONE', #21965 ) ;
#215189=ORIENTED_EDGE ( 'NONE', *, *, #151172, .F. ) ;
#215201=AXIS2_PLACEMENT_3D ( 'NONE', #227415, #209134, #27975 ) ;
#215224=CIRCLE ( 'NONE', #194403, 0.09999999999999530098 ) ;
#215228=CARTESIAN_POINT ( 'NONE',  ( -23.39999999999994529, 83.90000000001120384, -37.18565239344504647 ) ) ;
#215284=ORIENTED_EDGE ( 'NONE', *, *, #167427, .F. ) ;
#215310=CIRCLE ( 'NONE', #102864, 0.09999999999999982514 ) ;
#215326=CARTESIAN_POINT ( 'NONE',  ( -21.14999999999994174, 76.00000000001119815, -3.023107484524792277 ) ) ;
#215345=EDGE_CURVE ( 'NONE', #23181, #173183, #12090, .T. ) ;
#215361=CARTESIAN_POINT ( 'NONE',  ( -23.49999999999994316, 87.51781941433023349, -34.28670414799875488 ) ) ;
#215398=EDGE_CURVE ( 'NONE', #211446, #297, #50297, .T. ) ;
#215440=FACE_OUTER_BOUND ( 'NONE', #49817, .T. ) ;
#215456=VECTOR ( 'NONE', #132142, 1000.000000000000000 ) ;
#215659=CIRCLE ( 'NONE', #28273, 0.1000000000000045852 ) ;
#215818=EDGE_CURVE ( 'NONE', #40557, #28383, #89823, .T. ) ;
#215836=CIRCLE ( 'NONE', #103408, 0.1000000000000028644 ) ;
#215860=ORIENTED_EDGE ( 'NONE', *, *, #19328, .F. ) ;
#215934=ORIENTED_EDGE ( 'NONE', *, *, #196253, .T. ) ;
#215977=EDGE_CURVE ( 'NONE', #80879, #26247, #121280, .T. ) ;
#216024=CARTESIAN_POINT ( 'NONE',  ( -5.999999999999938716, 64.65000000001120384, -26.02310748452479316 ) ) ;
#216036=VERTEX_POINT ( 'NONE', #204377 ) ;
#216047=ORIENTED_EDGE ( 'NONE', *, *, #24841, .F. ) ;
#216183=FACE_OUTER_BOUND ( 'NONE', #119867, .T. ) ;
#216200=AXIS2_PLACEMENT_3D ( 'NONE', #158090, #18533, #74695 ) ;
#216224=DIRECTION ( 'NONE',  ( 0.000000000000000000, -0.9910827722268055195, -0.1332476588733540468 ) ) ;
#216225=EDGE_LOOP ( 'NONE', ( #205711, #74569, #250761, #31849 ) ) ;
#216259=ORIENTED_EDGE ( 'NONE', *, *, #204659, .T. ) ;
#216272=DIRECTION ( 'NONE',  ( -1.000000000000000000, -4.624352451196580357E-15, 3.439547145395922042E-14 ) ) ;
#216291=ORIENTED_EDGE ( 'NONE', *, *, #108189, .F. ) ;
#216323=DIRECTION ( 'NONE',  ( 0.000000000000000000, 1.000000000000000000, -0.000000000000000000 ) ) ;
#216327=CARTESIAN_POINT ( 'NONE',  ( 5.900000000000061640, 64.65000000001120384, -22.12310748452479103 ) ) ;
#216357=SPHERICAL_SURFACE ( 'NONE', #238102, 0.1000000000000000056 ) ;
#216400=ORIENTED_EDGE ( 'NONE', *, *, #6134, .T. ) ;
#216453=LINE ( 'NONE', #74426, #27144 ) ;
#216495=DIRECTION ( 'NONE',  ( 0.000000000000000000, 0.000000000000000000, -1.000000000000000000 ) ) ;
#216561=EDGE_CURVE ( 'NONE', #30313, #238821, #26400, .T. ) ;
#216605=CARTESIAN_POINT ( 'NONE',  ( 21.15000000000005187, 76.00000000001119815, -36.02310748452479316 ) ) ;
#216809=EDGE_LOOP ( 'NONE', ( #18243, #196390, #2698 ) ) ;
#216833=AXIS2_PLACEMENT_3D ( 'NONE', #150991, #110568, #190121 ) ;
#216846=CARTESIAN_POINT ( 'NONE',  ( -20.94999999999994600, 64.35000000001120668, -6.123107484524794586 ) ) ;
#216876=DIRECTION ( 'NONE',  ( 1.000000000000000000, -0.000000000000000000, -0.000000000000000000 ) ) ;
#216921=EDGE_LOOP ( 'NONE', ( #98956, #67801, #81843, #193705 ) ) ;
#216940=CARTESIAN_POINT ( 'NONE',  ( -23.49999999999994316, 82.84256550613280012, -26.34830530078816935 ) ) ;
#216962=VERTEX_POINT ( 'NONE', #1064 ) ;
#216999=AXIS2_PLACEMENT_3D ( 'NONE', #130002, #71355, #68773 ) ;
#217003=EDGE_CURVE ( 'NONE', #59396, #144177, #76437, .T. ) ;
#217049=DIRECTION ( 'NONE',  ( 0.000000000000000000, -1.000000000000000000, 0.000000000000000000 ) ) ;
#217050=EDGE_CURVE ( 'NONE', #40901, #23353, #100161, .T. ) ;
#217147=EDGE_CURVE ( 'NONE', #41849, #33512, #105649, .T. ) ;
#217204=CIRCLE ( 'NONE', #196559, 0.1000000000000002554 ) ;
#217255=DIRECTION ( 'NONE',  ( 1.284434275755705296E-16, -0.7071067811865471286, -0.7071067811865479058 ) ) ;
#217300=CARTESIAN_POINT ( 'NONE',  ( -0.8999999999999430678, 63.75000000001118394, -10.02310748452479139 ) ) ;
#217306=EDGE_CURVE ( 'NONE', #114442, #243775, #72554, .T. ) ;
#217317=AXIS2_PLACEMENT_3D ( 'NONE', #49531, #190338, #29995 ) ;
#217333=VECTOR ( 'NONE', #72255, 1000.000000000000114 ) ;
#217338=AXIS2_PLACEMENT_3D ( 'NONE', #76593, #57005, #113160 ) ;
#217357=CARTESIAN_POINT ( 'NONE',  ( -23.49999999999994316, 83.90000000001120384, -37.27310748452479316 ) ) ;
#217363=PLANE ( 'NONE',  #42084 ) ;
#217397=CARTESIAN_POINT ( 'NONE',  ( -21.04999999999994387, 74.83745509109094485, -44.02310748452479316 ) ) ;
#217415=DIRECTION ( 'NONE',  ( -0.000000000000000000, 0.000000000000000000, -1.000000000000000000 ) ) ;
#217443=AXIS2_PLACEMENT_3D ( 'NONE', #25793, #46617, #144427 ) ;
#217485=DIRECTION ( 'NONE',  ( 1.000000000000000000, -0.000000000000000000, -0.000000000000000000 ) ) ;
#217515=CARTESIAN_POINT ( 'NONE',  ( -13.39999999999994529, 67.72071067812984779, -21.02310748452479316 ) ) ;
#217531=AXIS2_PLACEMENT_3D ( 'NONE', #240589, #184458, #200185 ) ;
#217536=EDGE_LOOP ( 'NONE', ( #95448, #4299, #21649, #128775 ) ) ;
#217603=DIRECTION ( 'NONE',  ( 0.000000000000000000, 1.000000000000000000, 0.000000000000000000 ) ) ;
#217626=EDGE_LOOP ( 'NONE', ( #98263, #234395, #49804, #103257 ) ) ;
#217661=ORIENTED_EDGE ( 'NONE', *, *, #210810, .T. ) ;
#217782=TOROIDAL_SURFACE ( 'NONE', #38749, 4.041421356237310469, 0.1000000000000000056 ) ;
#217802=LINE ( 'NONE', #178739, #248895 ) ;
#217865=DIRECTION ( 'NONE',  ( -1.000000000000000000, 0.000000000000000000, 0.000000000000000000 ) ) ;
#217904=ADVANCED_FACE ( 'NONE', ( #181696 ), #242938, .F. ) ;
#217905=DIRECTION ( 'NONE',  ( 0.000000000000000000, 0.000000000000000000, -1.000000000000000000 ) ) ;
#218000=AXIS2_PLACEMENT_3D ( 'NONE', #9621, #31796, #68325 ) ;
#218031=EDGE_CURVE ( 'NONE', #249805, #189336, #27786, .T. ) ;
#218103=DIRECTION ( 'NONE',  ( 0.000000000000000000, 0.000000000000000000, 1.000000000000000000 ) ) ;
#218111=VERTEX_POINT ( 'NONE', #177577 ) ;
#218194=ORIENTED_EDGE ( 'NONE', *, *, #26610, .F. ) ;
#218205=FACE_OUTER_BOUND ( 'NONE', #160355, .T. ) ;
#218227=ADVANCED_FACE ( 'NONE', ( #77145 ), #138930, .T. ) ;
#218287=DIRECTION ( 'NONE',  ( 0.000000000000000000, 0.000000000000000000, -1.000000000000000000 ) ) ;
#218295=DIRECTION ( 'NONE',  ( -0.000000000000000000, -0.000000000000000000, 1.000000000000000000 ) ) ;
#218327=CARTESIAN_POINT ( 'NONE',  ( -21.14999999999994174, 77.83551161375991967, -47.52760213295649550 ) ) ;
#218359=ORIENTED_EDGE ( 'NONE', *, *, #56260, .F. ) ;
#218405=ORIENTED_EDGE ( 'NONE', *, *, #98773, .T. ) ;
#218447=ORIENTED_EDGE ( 'NONE', *, *, #93583, .F. ) ;
#218458=FACE_OUTER_BOUND ( 'NONE', #12025, .T. ) ;
#218510=DIRECTION ( 'NONE',  ( 0.000000000000000000, -1.000000000000000000, 0.000000000000000000 ) ) ;
#218587=TOROIDAL_SURFACE ( 'NONE', #168598, 2.699999999999999734, 0.1000000000000000056 ) ;
#218605=CARTESIAN_POINT ( 'NONE',  ( -23.49999999999994316, 83.90000000001120384, -34.77310748452479316 ) ) ;
#218622=DIRECTION ( 'NONE',  ( -1.000000000000000000, 0.000000000000000000, 0.000000000000000000 ) ) ;
#218647=CARTESIAN_POINT ( 'NONE',  ( -21.04999999999994387, 74.73834681386826162, -44.00978271863746016 ) ) ;
#218683=FACE_OUTER_BOUND ( 'NONE', #16113, .T. ) ;
#218729=FACE_OUTER_BOUND ( 'NONE', #238807, .T. ) ;
#218774=DIRECTION ( 'NONE',  ( 0.000000000000000000, 0.000000000000000000, -1.000000000000000000 ) ) ;
#218852=ORIENTED_EDGE ( 'NONE', *, *, #204659, .F. ) ;
#218863=AXIS2_PLACEMENT_3D ( 'NONE', #195938, #39444, #255839 ) ;
#218887=AXIS2_PLACEMENT_3D ( 'NONE', #222145, #224729, #29162 ) ;
#218913=EDGE_CURVE ( 'NONE', #106796, #73651, #247498, .T. ) ;
#218972=CARTESIAN_POINT ( 'NONE',  ( 21.15000000000005187, 64.35000000001120668, -3.123107484524795474 ) ) ;
#218992=EDGE_CURVE ( 'NONE', #84197, #179303, #141321, .T. ) ;
#219017=CIRCLE ( 'NONE', #214924, 0.1999999999999987899 ) ;
#219032=ORIENTED_EDGE ( 'NONE', *, *, #61929, .F. ) ;
#219051=DIRECTION ( 'NONE',  ( 0.000000000000000000, 0.000000000000000000, 1.000000000000000000 ) ) ;
#219084=DIRECTION ( 'NONE',  ( 0.000000000000000000, 0.000000000000000000, -1.000000000000000000 ) ) ;
#219129=ORIENTED_EDGE ( 'NONE', *, *, #99439, .T. ) ;
#219151=DIRECTION ( 'NONE',  ( 0.000000000000000000, 0.000000000000000000, -1.000000000000000000 ) ) ;
#219232=CARTESIAN_POINT ( 'NONE',  ( -20.94999999999994600, 65.35000000001120668, -3.023107484524792277 ) ) ;
#219235=CARTESIAN_POINT ( 'NONE',  ( 20.95000000000005613, 67.85000000001119247, -51.02310748452479316 ) ) ;
#219249=CARTESIAN_POINT ( 'NONE',  ( -21.04999999999994387, 76.00000000001119815, -40.17310748452479174 ) ) ;
#219250=CARTESIAN_POINT ( 'NONE',  ( -23.49999999999994316, 74.83745509109094485, -44.02310748452479316 ) ) ;
#219305=ORIENTED_EDGE ( 'NONE', *, *, #164724, .F. ) ;
#219336=CARTESIAN_POINT ( 'NONE',  ( 20.95000000000005613, 67.75000000001118394, -3.123107484524795474 ) ) ;
#219417=EDGE_LOOP ( 'NONE', ( #157351, #143436, #94825, #61904 ) ) ;
#219458=ORIENTED_EDGE ( 'NONE', *, *, #113053, .T. ) ;
#219515=AXIS2_PLACEMENT_3D ( 'NONE', #147080, #127537, #227921 ) ;
#219553=EDGE_CURVE ( 'NONE', #62069, #21878, #147135, .T. ) ;
#219587=CARTESIAN_POINT ( 'NONE',  ( -21.04999999999994387, 65.15000000001120384, -51.02310748452479316 ) ) ;
#219641=DIRECTION ( 'NONE',  ( 0.000000000000000000, 0.000000000000000000, -1.000000000000000000 ) ) ;
#219646=ORIENTED_EDGE ( 'NONE', *, *, #254311, .T. ) ;
#219660=CARTESIAN_POINT ( 'NONE',  ( -20.94999999999994600, 67.73741572762334329, -25.54575917482290848 ) ) ;
#219673=FACE_OUTER_BOUND ( 'NONE', #73412, .T. ) ;
#219686=CONICAL_SURFACE ( 'NONE', #103160, 4.000000000000000000, 0.7853981633974489451 ) ;
#219748=ORIENTED_EDGE ( 'NONE', *, *, #193118, .F. ) ;
#219760=DIRECTION ( 'NONE',  ( 0.000000000000000000, -0.9910827722268050755, 0.1332476588733589318 ) ) ;
#219796=DIRECTION ( 'NONE',  ( -0.000000000000000000, 1.000000000000000000, 0.000000000000000000 ) ) ;
#219855=EDGE_LOOP ( 'NONE', ( #39179, #157095, #33561, #244271 ) ) ;
#219938=DIRECTION ( 'NONE',  ( 0.000000000000000000, 1.000000000000000000, 0.000000000000000000 ) ) ;
#220027=EDGE_CURVE ( 'NONE', #26416, #89909, #202440, .T. ) ;
#220053=DIRECTION ( 'NONE',  ( 1.000000000000000000, 0.000000000000000000, 0.000000000000000000 ) ) ;
#220082=CARTESIAN_POINT ( 'NONE',  ( 0.9000000000000546452, 67.72071067812984779, -6.052396806406134644 ) ) ;
#220119=DIRECTION ( 'NONE',  ( 0.000000000000000000, 0.000000000000000000, 1.000000000000000000 ) ) ;
#220120=CARTESIAN_POINT ( 'NONE',  ( 20.95000000000005258, 65.35000000001120668, -3.123107484524795474 ) ) ;
#220403=ORIENTED_EDGE ( 'NONE', *, *, #67883, .F. ) ;
#220434=ORIENTED_EDGE ( 'NONE', *, *, #55293, .T. ) ;
#220441=AXIS2_PLACEMENT_3D ( 'NONE', #80850, #60006, #219084 ) ;
#220444=DIRECTION ( 'NONE',  ( 0.000000000000000000, 0.000000000000000000, -1.000000000000000000 ) ) ;
#220472=DIRECTION ( 'NONE',  ( 1.000000000000000000, 0.000000000000000000, 0.000000000000000000 ) ) ;
#220517=LINE ( 'NONE', #215361, #52230 ) ;
#220523=VECTOR ( 'NONE', #209679, 1000.000000000000114 ) ;
#220550=CARTESIAN_POINT ( 'NONE',  ( 23.40000000000004476, 84.00000000001119815, -37.18565239344504647 ) ) ;
#220729=DIRECTION ( 'NONE',  ( 1.000000000000000000, 0.000000000000000000, -0.000000000000000000 ) ) ;
#220746=AXIS2_PLACEMENT_3D ( 'NONE', #63095, #141358, #142624 ) ;
#220820=CARTESIAN_POINT ( 'NONE',  ( -21.14999999999994174, 64.35000000001120668, -30.12310748452479103 ) ) ;
#220836=FACE_OUTER_BOUND ( 'NONE', #173212, .T. ) ;
#220909=ORIENTED_EDGE ( 'NONE', *, *, #208820, .T. ) ;
#221055=CARTESIAN_POINT ( 'NONE',  ( 21.15000000000005542, 83.98667523412385094, -34.76145429838185663 ) ) ;
#221094=AXIS2_PLACEMENT_3D ( 'NONE', #149507, #64800, #183479 ) ;
#221116=DIRECTION ( 'NONE',  ( -0.000000000000000000, 1.000000000000000000, -0.000000000000000000 ) ) ;
#221188=DIRECTION ( 'NONE',  ( -0.000000000000000000, 1.000000000000000000, -0.000000000000000000 ) ) ;
#221217=DIRECTION ( 'NONE',  ( -0.000000000000000000, -1.000000000000000000, 8.673617379884045333E-16 ) ) ;
#221248=AXIS2_PLACEMENT_3D ( 'NONE', #51879, #68922, #48046 ) ;
#221278=VERTEX_POINT ( 'NONE', #29525 ) ;
#221456=AXIS2_PLACEMENT_3D ( 'NONE', #43368, #163316, #147595 ) ;
#221486=EDGE_CURVE ( 'NONE', #173183, #167224, #155888, .T. ) ;
#221495=VECTOR ( 'NONE', #202257, 1000.000000000000000 ) ;
#221516=ORIENTED_EDGE ( 'NONE', *, *, #172205, .F. ) ;
#221587=CARTESIAN_POINT ( 'NONE',  ( -23.49999999999994316, 74.83745509109094485, -44.02310748452479316 ) ) ;
#221601=CARTESIAN_POINT ( 'NONE',  ( -0.8999999999999437339, 64.35000000001120668, -7.323107484524790323 ) ) ;
#221692=CONICAL_SURFACE ( 'NONE', #21815, 4.000000000000000000, 0.7853981633974487231 ) ;
#221693=ORIENTED_EDGE ( 'NONE', *, *, #24505, .T. ) ;
#221709=VECTOR ( 'NONE', #185393, 1000.000000000000000 ) ;
#221768=VECTOR ( 'NONE', #217255, 1000.000000000000000 ) ;
#221818=AXIS2_PLACEMENT_3D ( 'NONE', #204709, #185167, #229432 ) ;
#221956=CARTESIAN_POINT ( 'NONE',  ( 23.40000000000005542, 74.94272479589878344, -3.123107484524795474 ) ) ;
#222145=CARTESIAN_POINT ( 'NONE',  ( 21.05000000000005400, 65.35000000001120668, -4.423107484524790856 ) ) ;
#222170=CARTESIAN_POINT ( 'NONE',  ( 21.15000000000005187, 82.78482233730476025, -26.42994920107286916 ) ) ;
#222212=DIRECTION ( 'NONE',  ( 1.000000000000000000, 0.000000000000000000, 0.000000000000000000 ) ) ;
#222243=CARTESIAN_POINT ( 'NONE',  ( -11.59999999999994458, 67.72071067812984779, -17.05239680640613642 ) ) ;
#222248=TOROIDAL_SURFACE ( 'NONE', #109839, 4.041421356237307805, 0.1000000000000000056 ) ;
#222337=CARTESIAN_POINT ( 'NONE',  ( -20.94999999999994245, 67.85000000001119247, -3.123107484524795474 ) ) ;
#222342=CARTESIAN_POINT ( 'NONE',  ( 21.15000000000005187, 77.85126707825561709, -47.62635315998165453 ) ) ;
#222356=LINE ( 'NONE', #164982, #26622 ) ;
#222418=ADVANCED_FACE ( 'NONE', ( #244710 ), #183478, .T. ) ;
#222419=VERTEX_POINT ( 'NONE', #66087 ) ;
#222480=LINE ( 'NONE', #148109, #237442 ) ;
#222486=DIRECTION ( 'NONE',  ( 0.000000000000000000, -0.9910827722268049644, 0.1332476588733589318 ) ) ;
#222498=CARTESIAN_POINT ( 'NONE',  ( -21.04999999999994387, 65.35000000001120668, -4.623107484524796362 ) ) ;
#222528=CYLINDRICAL_SURFACE ( 'NONE', #115083, 0.1000000000000028644 ) ;
#222615=DIRECTION ( 'NONE',  ( 1.000000000000000000, 0.000000000000000000, 0.000000000000000000 ) ) ;
#222627=FACE_OUTER_BOUND ( 'NONE', #28872, .T. ) ;
#222658=CYLINDRICAL_SURFACE ( 'NONE', #102929, 0.1000000000000002554 ) ;
#222671=EDGE_LOOP ( 'NONE', ( #185384, #215027, #36743 ) ) ;
#222738=DIRECTION ( 'NONE',  ( -0.000000000000000000, 1.000000000000000000, -0.000000000000000000 ) ) ;
#222834=EDGE_CURVE ( 'NONE', #241392, #255132, #245713, .T. ) ;
#222844=CARTESIAN_POINT ( 'NONE',  ( -20.94999999999994600, 65.15000000001120384, -3.123107484524795474 ) ) ;
#222850=DIRECTION ( 'NONE',  ( 1.000000000000000000, -0.000000000000000000, -0.000000000000000000 ) ) ;
#222890=CIRCLE ( 'NONE', #256151, 0.1999999999999987899 ) ;
#222909=CARTESIAN_POINT ( 'NONE',  ( -23.39999999999994529, 76.00000000001119815, -36.02310748452479316 ) ) ;
#222910=EDGE_LOOP ( 'NONE', ( #258073, #173390, #186359, #82381 ) ) ;
#222944=ORIENTED_EDGE ( 'NONE', *, *, #132758, .T. ) ;
#222972=VECTOR ( 'NONE', #83291, 1000.000000000000000 ) ;
#223043=DIRECTION ( 'NONE',  ( 0.000000000000000000, 0.9910827722268055195, 0.1332476588733540468 ) ) ;
#223087=CARTESIAN_POINT ( 'NONE',  ( 0.9000000000000535350, 64.25000000001119815, -7.323107484524790323 ) ) ;
#223093=DIRECTION ( 'NONE',  ( 0.000000000000000000, -0.8164390028469705740, 0.5774316882803059992 ) ) ;
#223120=VECTOR ( 'NONE', #60801, 1000.000000000000000 ) ;
#223133=EDGE_CURVE ( 'NONE', #149012, #249539, #115192, .T. ) ;
#223138=DIRECTION ( 'NONE',  ( 0.000000000000000000, 1.000000000000000000, 0.000000000000000000 ) ) ;
#223259=DIRECTION ( 'NONE',  ( 0.000000000000000000, 0.000000000000000000, 1.000000000000000000 ) ) ;
#223313=LINE ( 'NONE', #145066, #255450 ) ;
#223323=DIRECTION ( 'NONE',  ( 1.000000000000000000, 0.000000000000000000, 0.000000000000000000 ) ) ;
#223326=ORIENTED_EDGE ( 'NONE', *, *, #208820, .F. ) ;
#223332=EDGE_CURVE ( 'NONE', #64966, #245973, #16942, .T. ) ;
#223362=CYLINDRICAL_SURFACE ( 'NONE', #102247, 0.1000000000000028644 ) ;
#223392=VECTOR ( 'NONE', #219796, 1000.000000000000000 ) ;
#223422=AXIS2_PLACEMENT_3D ( 'NONE', #63274, #41180, #166272 ) ;
#223469=FACE_OUTER_BOUND ( 'NONE', #187760, .T. ) ;
#223480=CARTESIAN_POINT ( 'NONE',  ( 6.000000000000061284, 64.75000000001119815, -22.12310748452479103 ) ) ;
#223504=VERTEX_POINT ( 'NONE', #121967 ) ;
#223512=DIRECTION ( 'NONE',  ( 0.000000000000000000, 1.000000000000000000, 0.000000000000000000 ) ) ;
#223538=AXIS2_PLACEMENT_3D ( 'NONE', #244933, #66307, #174440 ) ;
#223548=VECTOR ( 'NONE', #242672, 1000.000000000000000 ) ;
#223557=AXIS2_PLACEMENT_3D ( 'NONE', #248294, #68381, #205297 ) ;
#223589=DIRECTION ( 'NONE',  ( 0.000000000000000000, 0.1332476588733448597, 0.9910827722268067408 ) ) ;
#223631=DIRECTION ( 'NONE',  ( 0.000000000000000000, 1.000000000000000000, 0.000000000000000000 ) ) ;
#223678=EDGE_CURVE ( 'NONE', #74886, #227850, #74870, .T. ) ;
#223685=ORIENTED_EDGE ( 'NONE', *, *, #242490, .T. ) ;
#223704=ORIENTED_EDGE ( 'NONE', *, *, #200124, .F. ) ;
#223716=ORIENTED_EDGE ( 'NONE', *, *, #112274, .T. ) ;
#223760=AXIS2_PLACEMENT_3D ( 'NONE', #6318, #148422, #244937 ) ;
#223767=DIRECTION ( 'NONE',  ( 0.000000000000000000, 0.000000000000000000, 1.000000000000000000 ) ) ;
#223785=DIRECTION ( 'NONE',  ( -1.000000000000000000, 0.000000000000000000, 0.000000000000000000 ) ) ;
#223801=CARTESIAN_POINT ( 'NONE',  ( 23.40000000000005187, 64.35000000001120668, -51.02310748452479316 ) ) ;
#223831=AXIS2_PLACEMENT_3D ( 'NONE', #27224, #127577, #207121 ) ;
#223880=DIRECTION ( 'NONE',  ( 0.000000000000000000, 0.000000000000000000, 1.000000000000000000 ) ) ;
#223887=EDGE_LOOP ( 'NONE', ( #80270, #77396, #48860, #52528 ) ) ;
#223932=LINE ( 'NONE', #203100, #156658 ) ;
#223998=DIRECTION ( 'NONE',  ( 1.000000000000000000, -0.000000000000000000, -0.000000000000000000 ) ) ;
#224041=VERTEX_POINT ( 'NONE', #167243 ) ;
#224060=ORIENTED_EDGE ( 'NONE', *, *, #205775, .T. ) ;
#224133=CLOSED_SHELL ( 'NONE', ( #93897, #47892, #33653, #170708, #97719, #139357, #64147, #80802, #7186, #51314, #182074, #120636, #213007, #179478, #100553, #2770, #17306, #181923, #191589, #169559, #44640, #9334, #66194, #198188, #48023, #94882, #121358, #108761, #19307, #258021, #193846, #211537, #11068, #11001, #241014, #208471, #4014, #86740, #197326, #164529, #44662, #183888, #186011, #205671, #119718, #13122, #224532, #171339, #163535, #70517, #190255, #154595, #115889, #118161, #191048, #179096, #122679, #258020, #94552, #163372, #61318, #94738, #139505, #57481, #69428, #89839, #99120, #2628, #92925, #86458, #206268, #233916, #103919, #185211, #1940, #100690, #68652, #56422, #65402, #81514, #59692, #42662, #188399, #222418, #149592, #137074, #67560, #94021, #19654, #138162, #32751, #242608, #159916, #231090, #174871, #37111, #18072, #49478, #113408, #138811, #101697, #153954, #189282, #22296, #172687, #182188, #37556, #71753, #189242, #27508, #120858, #15639, #42922, #71572, #137581, #54086, #51408, #90143, #191102, #64823, #81975, #76630, #127970, #192267, #182708, #140081, #204178, #162066, #119834, #186235, #139084, #50499, #153976, #33444, #217904, #212193, #58763, #148720, #123805, #97289, #118623, #204649, #236510, #12695, #159095, #98391, #237860, #139395, #7836, #46428, #242785, #17858, #140897, #147112, #70115, #61441, #214578, #96858, #91979, #227760, #65331, #45270, #37992, #92245, #207098, #232717, #35664, #48202, #227511, #246503, #69526, #131837, #17048, #154468, #29554, #156589, #7195, #25598, #62841, #188049, #167470, #95644, #175490, #186716, #159322, #100201, #251266, #31939, #80523, #47469, #33054, #56734, #147879, #152926, #57846, #62765, #253991, #99107, #241167, #29631, #125646, #54997, #204100, #11762, #176744, #141176, #88574, #176264, #74765, #179137, #131958, #89495, #165784, #150158, #78273, #203018, #70292, #71787, #101958, #128554, #257949, #191055, #57699, #158952, #244493, #97946, #248633, #117888, #38320, #62649, #127439, #70202, #186045, #167916, #159473, #112352, #257709, #255235, #101123, #169155, #159750, #218227, #225111, #230087, #147758, #101059, #125203, #198506, #230127, #206439, #121734, #114503, #71374, #108850, #80934, #59645, #18701, #190458, #7990, #237126, #98754, #94791, #145853, #184515, #194053, #169381, #19869, #81736, #102231, #126012, #167876, #87145, #51905, #228676, #89373, #113604, #244780, #60641, #51797, #100852, #241339, #147934, #70066, #179579, #39348, #178031, #150587 ) ) ;
#224194=DIRECTION ( 'NONE',  ( -1.000000000000000000, 0.000000000000000000, 0.000000000000000000 ) ) ;
#224199=EDGE_CURVE ( 'NONE', #218111, #187553, #58100, .T. ) ;
#224220=CARTESIAN_POINT ( 'NONE',  ( -5.999999999999938716, 64.65000000001120384, -22.02310748452479316 ) ) ;
#224235=VERTEX_POINT ( 'NONE', #163077 ) ;
#224246=DIRECTION ( 'NONE',  ( -1.000000000000000000, 0.000000000000000000, 0.000000000000000000 ) ) ;
#224261=DIRECTION ( 'NONE',  ( 0.000000000000000000, 0.000000000000000000, -1.000000000000000000 ) ) ;
#224280=EDGE_CURVE ( 'NONE', #80961, #222419, #99607, .T. ) ;
#224290=ORIENTED_EDGE ( 'NONE', *, *, #47048, .T. ) ;
#224310=VECTOR ( 'NONE', #76152, 1000.000000000000000 ) ;
#224332=DIRECTION ( 'NONE',  ( 0.000000000000000000, 0.000000000000000000, -1.000000000000000000 ) ) ;
#224392=DIRECTION ( 'NONE',  ( 0.000000000000000000, 0.000000000000000000, 1.000000000000000000 ) ) ;
#224396=DIRECTION ( 'NONE',  ( -0.000000000000000000, 0.000000000000000000, 1.000000000000000000 ) ) ;
#224441=CARTESIAN_POINT ( 'NONE',  ( -23.39999999999994529, 74.14873292176677921, -47.62635315998165453 ) ) ;
#224453=CARTESIAN_POINT ( 'NONE',  ( -23.39999999999994529, 64.35000000001120668, -51.02310748452479316 ) ) ;
#224455=CIRCLE ( 'NONE', #228577, 0.1000000000000002554 ) ;
#224520=ORIENTED_EDGE ( 'NONE', *, *, #210203, .T. ) ;
#224532=ADVANCED_FACE ( 'NONE', ( #16834 ), #254125, .F. ) ;
#224538=DIRECTION ( 'NONE',  ( -1.000000000000000000, -0.000000000000000000, -0.000000000000000000 ) ) ;
#224618=DIRECTION ( 'NONE',  ( 1.000000000000000000, 0.000000000000000000, 0.000000000000000000 ) ) ;
#224621=VERTEX_POINT ( 'NONE', #23264 ) ;
#224651=CARTESIAN_POINT ( 'NONE',  ( 21.15000000000005542, 83.80000000001119531, -51.02310748452479316 ) ) ;
#224720=EDGE_CURVE ( 'NONE', #122419, #119288, #4148, .T. ) ;
#224729=DIRECTION ( 'NONE',  ( -1.000000000000000000, 0.000000000000000000, -0.000000000000000000 ) ) ;
#224857=ORIENTED_EDGE ( 'NONE', *, *, #171534, .T. ) ;
#224879=CARTESIAN_POINT ( 'NONE',  ( -23.39999999999994529, 87.50449464844290048, -37.85861909827351468 ) ) ;
#224917=DIRECTION ( 'NONE',  ( 0.000000000000000000, 0.000000000000000000, 1.000000000000000000 ) ) ;
#224967=DIRECTION ( 'NONE',  ( -0.000000000000000000, 0.9910827722268050755, 0.1332476588733589318 ) ) ;
#225099=CARTESIAN_POINT ( 'NONE',  ( -5.999999999999938716, 64.25000000001119815, -22.12310748452479103 ) ) ;
#225100=CARTESIAN_POINT ( 'NONE',  ( -23.49999999999994316, 87.75000000001119815, -3.123107484524795474 ) ) ;
#225111=ADVANCED_FACE ( 'NONE', ( #168587 ), #162573, .T. ) ;
#225138=UNCERTAINTY_MEASURE_WITH_UNIT (LENGTH_MEASURE( 1.000000000000000082E-05 ), #185556, 'distance_accuracy_value', 'NONE');
#225139=DIRECTION ( 'NONE',  ( 0.000000000000000000, 0.9910827722268055195, 0.1332476588733540468 ) ) ;
#225140=CYLINDRICAL_SURFACE ( 'NONE', #221094, 0.1000000000000028644 ) ;
#225183=ORIENTED_EDGE ( 'NONE', *, *, #148924, .T. ) ;
#225192=CARTESIAN_POINT ( 'NONE',  ( 23.40000000000005542, 74.26359666348515987, -47.54092689884382850 ) ) ;
#225196=EDGE_LOOP ( 'NONE', ( #198851, #231591, #35823, #190871 ) ) ;
#225250=VECTOR ( 'NONE', #20456, 1000.000000000000000 ) ;
#225258=DIRECTION ( 'NONE',  ( 1.000000000000000000, -0.000000000000000000, 0.000000000000000000 ) ) ;
#225270=VERTEX_POINT ( 'NONE', #236203 ) ;
#225283=ORIENTED_EDGE ( 'NONE', *, *, #157293, .T. ) ;
#225293=ORIENTED_EDGE ( 'NONE', *, *, #163938, .T. ) ;
#225304=ORIENTED_EDGE ( 'NONE', *, *, #149141, .T. ) ;
#225314=EDGE_CURVE ( 'NONE', #165490, #61312, #91994, .T. ) ;
#225337=ORIENTED_EDGE ( 'NONE', *, *, #105775, .F. ) ;
#225363=CARTESIAN_POINT ( 'NONE',  ( -23.49999999999994316, 64.35000000001120668, -21.92310748452479174 ) ) ;
#225434=EDGE_CURVE ( 'NONE', #223504, #150828, #166870, .T. ) ;
#225511=LINE ( 'NONE', #149881, #242866 ) ;
#225526=AXIS2_PLACEMENT_3D ( 'NONE', #97408, #197820, #193999 ) ;
#225558=AXIS2_PLACEMENT_3D ( 'NONE', #167075, #52211, #150068 ) ;
#225587=ORIENTED_EDGE ( 'NONE', *, *, #16409, .T. ) ;
#225595=CYLINDRICAL_SURFACE ( 'NONE', #248493, 0.1000000000000028644 ) ;
#225733=CARTESIAN_POINT ( 'NONE',  ( 11.60000000000006004, 67.75000000001118394, -25.06452884076210097 ) ) ;
#225762=LINE ( 'NONE', #165834, #125369 ) ;
#225793=ORIENTED_EDGE ( 'NONE', *, *, #190134, .T. ) ;
#225796=CARTESIAN_POINT ( 'NONE',  ( 23.40000000000005187, 74.16448838626247664, -47.52760213295649550 ) ) ;
#225804=AXIS2_PLACEMENT_3D ( 'NONE', #71879, #230963, #148847 ) ;
#225928=ORIENTED_EDGE ( 'NONE', *, *, #249137, .F. ) ;
#225934=VECTOR ( 'NONE', #124639, 1000.000000000000000 ) ;
#225949=CARTESIAN_POINT ( 'NONE',  ( 23.50000000000004263, 74.73834681386826162, -44.00978271863746016 ) ) ;
#226011=VECTOR ( 'NONE', #61568, 1000.000000000000000 ) ;
#226081=EDGE_LOOP ( 'NONE', ( #235278, #14135 ) ) ;
#226105=AXIS2_PLACEMENT_3D ( 'NONE', #162686, #184801, #124844 ) ;
#226114=CYLINDRICAL_SURFACE ( 'NONE', #115967, 5.000000000000000888 ) ;
#226198=ORIENTED_EDGE ( 'NONE', *, *, #71480, .T. ) ;
#226270=VERTEX_POINT ( 'NONE', #59491 ) ;
#226272=VECTOR ( 'NONE', #256487, 1000.000000000000000 ) ;
#226321=CARTESIAN_POINT ( 'NONE',  ( -0.8999999999999437339, 64.25000000001119815, -12.72310748452478890 ) ) ;
#226367=EDGE_CURVE ( 'NONE', #9346, #63115, #206740, .T. ) ;
#226436=CARTESIAN_POINT ( 'NONE',  ( 20.95000000000005613, 65.15000000001120384, -4.423107484524790856 ) ) ;
#226445=AXIS2_PLACEMENT_3D ( 'NONE', #119785, #20678, #234566 ) ;
#226448=EDGE_CURVE ( 'NONE', #158981, #90057, #107632, .T. ) ;
#226498=EDGE_CURVE ( 'NONE', #80255, #100189, #80633, .T. ) ;
#226526=CIRCLE ( 'NONE', #30957, 2.599999999999998312 ) ;
#226542=ORIENTED_EDGE ( 'NONE', *, *, #141265, .T. ) ;
#226585=DIRECTION ( 'NONE',  ( 0.000000000000000000, 0.000000000000000000, 1.000000000000000000 ) ) ;
#226632=AXIS2_PLACEMENT_3D ( 'NONE', #51463, #131028, #94461 ) ;
#226635=AXIS2_PLACEMENT_3D ( 'NONE', #180253, #241504, #165837 ) ;
#226645=DIRECTION ( 'NONE',  ( -0.000000000000000000, 0.000000000000000000, 1.000000000000000000 ) ) ;
#226658=LINE ( 'NONE', #207119, #58158 ) ;
#226662=AXIS2_PLACEMENT_3D ( 'NONE', #155082, #117209, #136752 ) ;
#226784=EDGE_CURVE ( 'NONE', #36158, #133767, #39183, .T. ) ;
#226924=DIRECTION ( 'NONE',  ( 0.000000000000000000, 0.9910827722268050755, 0.1332476588733589318 ) ) ;
#227002=ORIENTED_EDGE ( 'NONE', *, *, #61072, .F. ) ;
#227042=DIRECTION ( 'NONE',  ( 1.000000000000000000, -0.000000000000000000, -0.000000000000000000 ) ) ;
#227123=CARTESIAN_POINT ( 'NONE',  ( 20.95000000000005258, 64.35000000001120668, -30.02310748452479316 ) ) ;
#227189=ORIENTED_EDGE ( 'NONE', *, *, #157839, .T. ) ;
#227207=EDGE_LOOP ( 'NONE', ( #206541, #39172, #202500, #207300 ) ) ;
#227292=DIRECTION ( 'NONE',  ( -1.000000000000000000, 0.000000000000000000, 0.000000000000000000 ) ) ;
#227314=ORIENTED_EDGE ( 'NONE', *, *, #119766, .T. ) ;
#227406=DIRECTION ( 'NONE',  ( 0.000000000000000000, -1.000000000000000000, 0.000000000000000000 ) ) ;
#227415=CARTESIAN_POINT ( 'NONE',  ( -23.39999999999994529, 76.00000000001119815, -36.02310748452479316 ) ) ;
#227425=DIRECTION ( 'NONE',  ( 1.000000000000000000, -0.000000000000000000, 0.000000000000000000 ) ) ;
#227473=CIRCLE ( 'NONE', #181707, 11.74999999999999645 ) ;
#227511=ADVANCED_FACE ( 'NONE', ( #51697 ), #43618, .T. ) ;
#227678=DIRECTION ( 'NONE',  ( 1.000000000000000000, 0.000000000000000000, 0.000000000000000000 ) ) ;
#227718=DIRECTION ( 'NONE',  ( 1.000000000000000000, 0.000000000000000000, 0.000000000000000000 ) ) ;
#227719=CARTESIAN_POINT ( 'NONE',  ( -23.39999999999994529, 77.84910827723388138, -47.62873275725970501 ) ) ;
#227747=LINE ( 'NONE', #129921, #77967 ) ;
#227760=ADVANCED_FACE ( 'NONE', ( #161110 ), #243189, .T. ) ;
#227803=CARTESIAN_POINT ( 'NONE',  ( -23.39999999999994529, 74.26359666348515987, -47.54092689884382850 ) ) ;
#227826=TOROIDAL_SURFACE ( 'NONE', #223538, 4.900000000000000355, 0.1000000000000000056 ) ;
#227850=VERTEX_POINT ( 'NONE', #171411 ) ;
#227854=AXIS2_PLACEMENT_3D ( 'NONE', #61336, #224246, #5177 ) ;
#227921=DIRECTION ( 'NONE',  ( 0.000000000000000000, 0.000000000000000000, 1.000000000000000000 ) ) ;
#227966=ORIENTED_EDGE ( 'NONE', *, *, #68832, .F. ) ;
#227971=EDGE_CURVE ( 'NONE', #73109, #21187, #231262, .T. ) ;
#227973=DIRECTION ( 'NONE',  ( 0.000000000000000000, 0.000000000000000000, -1.000000000000000000 ) ) ;
#228023=CYLINDRICAL_SURFACE ( 'NONE', #196414, 0.09999999999999939493 ) ;
#228028=VECTOR ( 'NONE', #5000, 1000.000000000000000 ) ;
#228114=CARTESIAN_POINT ( 'NONE',  ( 21.15000000000005542, 79.78873604695631627, -7.297728304630792806 ) ) ;
#228120=ORIENTED_EDGE ( 'NONE', *, *, #199748, .T. ) ;
#228141=VECTOR ( 'NONE', #74072, 1000.000000000000000 ) ;
#228143=LINE ( 'NONE', #46905, #209832 ) ;
#228202=ORIENTED_EDGE ( 'NONE', *, *, #157382, .T. ) ;
#228307=DIRECTION ( 'NONE',  ( 0.000000000000000000, 0.000000000000000000, 1.000000000000000000 ) ) ;
#228408=DIRECTION ( 'NONE',  ( 0.000000000000000000, 0.000000000000000000, -1.000000000000000000 ) ) ;
#228453=AXIS2_PLACEMENT_3D ( 'NONE', #13376, #92890, #172495 ) ;
#228458=EDGE_CURVE ( 'NONE', #115551, #170938, #39907, .T. ) ;
#228468=CIRCLE ( 'NONE', #65564, 0.1999999999999987899 ) ;
#228476=VERTEX_POINT ( 'NONE', #231705 ) ;
#228570=CARTESIAN_POINT ( 'NONE',  ( 23.40000000000005187, 79.88763423575340994, -7.282924647898262549 ) ) ;
#228577=AXIS2_PLACEMENT_3D ( 'NONE', #7939, #224392, #165740 ) ;
#228592=EDGE_CURVE ( 'NONE', #20544, #89909, #27638, .T. ) ;
#228645=CARTESIAN_POINT ( 'NONE',  ( 21.15000000000005542, 87.50449464844290048, -37.85861909827351468 ) ) ;
#228676=ADVANCED_FACE ( 'NONE', ( #197682 ), #79000, .F. ) ;
#228678=ORIENTED_EDGE ( 'NONE', *, *, #28897, .F. ) ;
#228693=ORIENTED_EDGE ( 'NONE', *, *, #63929, .T. ) ;
#228715=AXIS2_PLACEMENT_3D ( 'NONE', #201024, #22403, #144879 ) ;
#228732=DIRECTION ( 'NONE',  ( 0.000000000000000000, 0.000000000000000000, -1.000000000000000000 ) ) ;
#228750=LINE ( 'NONE', #48805, #257183 ) ;
#228765=ORIENTED_EDGE ( 'NONE', *, *, #4449, .F. ) ;
#228769=DIRECTION ( 'NONE',  ( 1.000000000000000000, -0.000000000000000000, -0.000000000000000000 ) ) ;
#228811=LINE ( 'NONE', #129698, #60519 ) ;
#228876=DIRECTION ( 'NONE',  ( 0.000000000000000000, -1.000000000000000000, 0.000000000000000000 ) ) ;
#228921=EDGE_CURVE ( 'NONE', #103163, #239496, #15130, .T. ) ;
#228943=DIRECTION ( 'NONE',  ( 1.000000000000000000, -0.000000000000000000, -0.000000000000000000 ) ) ;
#229003=DIRECTION ( 'NONE',  ( 0.000000000000000000, 0.000000000000000000, -1.000000000000000000 ) ) ;
#229150=ORIENTED_EDGE ( 'NONE', *, *, #235505, .T. ) ;
#229177=ORIENTED_EDGE ( 'NONE', *, *, #228921, .F. ) ;
#229186=VECTOR ( 'NONE', #49311, 1000.000000000000000 ) ;
#229188=DIRECTION ( 'NONE',  ( 1.444674012291107001E-15, -0.1332476588733650935, -0.9910827722268042983 ) ) ;
#229271=FACE_OUTER_BOUND ( 'NONE', #143862, .T. ) ;
#229330=EDGE_CURVE ( 'NONE', #135971, #60723, #190704, .T. ) ;
#229333=CIRCLE ( 'NONE', #216833, 0.09999999999999939493 ) ;
#229334=CIRCLE ( 'NONE', #237700, 0.1000000000000028644 ) ;
#229380=DIRECTION ( 'NONE',  ( -1.000000000000000000, 0.000000000000000000, -0.000000000000000000 ) ) ;
#229432=DIRECTION ( 'NONE',  ( 0.000000000000000000, 0.000000000000000000, -1.000000000000000000 ) ) ;
#229445=CARTESIAN_POINT ( 'NONE',  ( 20.95000000000005969, 67.73741572762334329, -25.54575917482290848 ) ) ;
#229461=VECTOR ( 'NONE', #162562, 1000.000000000000000 ) ;
#229540=FACE_OUTER_BOUND ( 'NONE', #126449, .T. ) ;
#229558=DIRECTION ( 'NONE',  ( 0.000000000000000000, 0.000000000000000000, 1.000000000000000000 ) ) ;
#229638=AXIS2_PLACEMENT_3D ( 'NONE', #67000, #106099, #146517 ) ;
#229671=CIRCLE ( 'NONE', #79790, 0.1000000000000002554 ) ;
#229702=DIRECTION ( 'NONE',  ( 0.000000000000000000, 1.387778780781406043E-13, 1.000000000000000000 ) ) ;
#229710=ORIENTED_EDGE ( 'NONE', *, *, #6253, .T. ) ;
#229790=CARTESIAN_POINT ( 'NONE',  ( -0.8999999999999437339, 66.35000000001119247, -7.423107484524793520 ) ) ;
#229804=ORIENTED_EDGE ( 'NONE', *, *, #36412, .T. ) ;
#229805=ORIENTED_EDGE ( 'NONE', *, *, #39273, .F. ) ;
#229835=DIRECTION ( 'NONE',  ( -0.000000000000000000, 1.000000000000000000, -0.000000000000000000 ) ) ;
#229847=LINE ( 'NONE', #29127, #116532 ) ;
#229851=EDGE_CURVE ( 'NONE', #12214, #150828, #144655, .T. ) ;
#229867=AXIS2_PLACEMENT_3D ( 'NONE', #65767, #227406, #10948 ) ;
#229928=DIRECTION ( 'NONE',  ( 0.000000000000000000, -0.000000000000000000, 1.000000000000000000 ) ) ;
#229940=CYLINDRICAL_SURFACE ( 'NONE', #31049, 0.1000000000000021844 ) ;
#229975=DIRECTION ( 'NONE',  ( 0.000000000000000000, -1.000000000000000000, 0.000000000000000000 ) ) ;
#229977=EDGE_CURVE ( 'NONE', #244869, #37851, #161436, .T. ) ;
#229998=CARTESIAN_POINT ( 'NONE',  ( 0.9000000000000547562, 64.35000000001120668, -7.323107484524793875 ) ) ;
#230087=ADVANCED_FACE ( 'NONE', ( #52769 ), #11100, .T. ) ;
#230118=CARTESIAN_POINT ( 'NONE',  ( 20.95000000000005613, 67.65000000001118963, -3.023107484524792277 ) ) ;
#230127=ADVANCED_FACE ( 'NONE', ( #14962 ), #54063, .T. ) ;
#230189=CIRCLE ( 'NONE', #205039, 0.1000000000000002554 ) ;
#230231=CIRCLE ( 'NONE', #113710, 0.1000000000000032391 ) ;
#230235=ORIENTED_EDGE ( 'NONE', *, *, #98346, .F. ) ;
#230246=ORIENTED_EDGE ( 'NONE', *, *, #169312, .T. ) ;
#230416=CIRCLE ( 'NONE', #197091, 0.1000000000000002554 ) ;
#230430=EDGE_CURVE ( 'NONE', #179524, #150828, #124325, .T. ) ;
#230447=ORIENTED_EDGE ( 'NONE', *, *, #187811, .F. ) ;
#230475=CARTESIAN_POINT ( 'NONE',  ( -21.14999999999994174, 74.14873292176677921, -47.62635315998165453 ) ) ;
#230483=EDGE_LOOP ( 'NONE', ( #9838, #154867, #118458 ) ) ;
#230489=CARTESIAN_POINT ( 'NONE',  ( -23.49999999999994316, 87.50449464844290048, -34.18759587077607165 ) ) ;
#230533=DIRECTION ( 'NONE',  ( -1.155739209832885601E-15, -0.9910827722268042983, 0.1332476588733650935 ) ) ;
#230547=CYLINDRICAL_SURFACE ( 'NONE', #38569, 0.1000000000000028644 ) ;
#230635=VERTEX_POINT ( 'NONE', #156755 ) ;
#230641=AXIS2_PLACEMENT_3D ( 'NONE', #238646, #59984, #139529 ) ;
#230663=DIRECTION ( 'NONE',  ( 1.000000000000000000, -0.000000000000000000, -0.000000000000000000 ) ) ;
#230672=CYLINDRICAL_SURFACE ( 'NONE', #194854, 0.1000000000000002554 ) ;
#230707=CARTESIAN_POINT ( 'NONE',  ( -23.39999999999994529, 87.51781941433023349, -37.75951082105083145 ) ) ;
#230720=ORIENTED_EDGE ( 'NONE', *, *, #207179, .T. ) ;
#230726=CARTESIAN_POINT ( 'NONE',  ( -23.39999999999994529, 87.60324567546805952, -37.87437456276921210 ) ) ;
#230761=AXIS2_PLACEMENT_3D ( 'NONE', #238386, #59725, #62324 ) ;
#230765=LINE ( 'NONE', #135476, #98610 ) ;
#230772=DIRECTION ( 'NONE',  ( 0.000000000000000000, -1.000000000000000000, 0.000000000000000000 ) ) ;
#230793=EDGE_CURVE ( 'NONE', #107651, #150745, #65322, .T. ) ;
#230835=DIRECTION ( 'NONE',  ( -1.000000000000000000, -0.000000000000000000, -0.000000000000000000 ) ) ;
#230847=EDGE_LOOP ( 'NONE', ( #48561, #170877, #24842, #125219 ) ) ;
#230852=DIRECTION ( 'NONE',  ( -1.000000000000000000, 0.000000000000000000, -0.000000000000000000 ) ) ;
#230912=VERTEX_POINT ( 'NONE', #57539 ) ;
#230914=ORIENTED_EDGE ( 'NONE', *, *, #38183, .F. ) ;
#230955=CARTESIAN_POINT ( 'NONE',  ( -5.899999999999938183, 64.65000000001120384, -22.12310748452479103 ) ) ;
#230960=VERTEX_POINT ( 'NONE', #139638 ) ;
#230963=DIRECTION ( 'NONE',  ( 0.000000000000000000, -1.000000000000000000, 0.000000000000000000 ) ) ;
#231038=EDGE_LOOP ( 'NONE', ( #17923, #79947, #55207, #221516 ) ) ;
#231090=ADVANCED_FACE ( 'NONE', ( #83506 ), #202212, .T. ) ;
#231099=DIRECTION ( 'NONE',  ( 1.000000000000000000, -0.000000000000000000, -0.000000000000000000 ) ) ;
#231118=AXIS2_PLACEMENT_3D ( 'NONE', #156936, #99474, #180329 ) ;
#231262=CIRCLE ( 'NONE', #185449, 0.09999999999999939493 ) ;
#231347=ORIENTED_EDGE ( 'NONE', *, *, #28897, .T. ) ;
#231351=PLANE ( 'NONE',  #148064 ) ;
#231379=VERTEX_POINT ( 'NONE', #158946 ) ;
#231414=CARTESIAN_POINT ( 'NONE',  ( -20.94999999999994600, 67.65000000001118963, -25.49719488170504533 ) ) ;
#231440=ORIENTED_EDGE ( 'NONE', *, *, #252133, .F. ) ;
#231496=ORIENTED_EDGE ( 'NONE', *, *, #164789, .T. ) ;
#231529=FACE_OUTER_BOUND ( 'NONE', #23762, .T. ) ;
#231549=EDGE_LOOP ( 'NONE', ( #210531, #191960, #240922, #142203 ) ) ;
#231574=ORIENTED_EDGE ( 'NONE', *, *, #83837, .F. ) ;
#231591=ORIENTED_EDGE ( 'NONE', *, *, #148987, .F. ) ;
#231705=CARTESIAN_POINT ( 'NONE',  ( -23.39999999999994529, 82.78482233730476025, -26.42994920107286916 ) ) ;
#231713=AXIS2_PLACEMENT_3D ( 'NONE', #100424, #203414, #24805 ) ;
#231820=CARTESIAN_POINT ( 'NONE',  ( 21.15000000000005542, 76.00000000001119815, -3.023107484524792277 ) ) ;
#231822=DIRECTION ( 'NONE',  ( 0.000000000000000000, -1.000000000000000000, -0.000000000000000000 ) ) ;
#231834=TOROIDAL_SURFACE ( 'NONE', #65211, 0.2000000000000000111, 0.1000000000000000056 ) ;
#231870=VERTEX_POINT ( 'NONE', #70775 ) ;
#231961=ORIENTED_EDGE ( 'NONE', *, *, #239154, .T. ) ;
#231965=CARTESIAN_POINT ( 'NONE',  ( 23.50000000000005684, 83.80000000001119531, -37.18565239344504647 ) ) ;
#232003=CARTESIAN_POINT ( 'NONE',  ( -11.59999999999994458, 67.75000000001118394, -25.06452884076210452 ) ) ;
#232068=ORIENTED_EDGE ( 'NONE', *, *, #74182, .F. ) ;
#232072=AXIS2_PLACEMENT_3D ( 'NONE', #179057, #53936, #133479 ) ;
#232114=CARTESIAN_POINT ( 'NONE',  ( 21.15000000000005187, 76.00000000001119815, -36.02310748452479316 ) ) ;
#232118=DIRECTION ( 'NONE',  ( 0.000000000000000000, 0.1332476588733448597, -0.9910827722268067408 ) ) ;
#232129=CARTESIAN_POINT ( 'NONE',  ( -23.49999999999994316, 83.90000000001120384, -37.18565239344504647 ) ) ;
#232163=ORIENTED_EDGE ( 'NONE', *, *, #212514, .T. ) ;
#232191=AXIS2_PLACEMENT_3D ( 'NONE', #184353, #7009, #24030 ) ;
#232208=CARTESIAN_POINT ( 'NONE',  ( -0.8999999999999437339, 64.35000000001120668, -12.72310748452478890 ) ) ;
#232253=CARTESIAN_POINT ( 'NONE',  ( -21.04999999999994387, 77.36076146337680370, -43.99645795275012006 ) ) ;
#232296=CARTESIAN_POINT ( 'NONE',  ( 21.15000000000005187, 76.00000000001119815, -36.02310748452479316 ) ) ;
#232304=DIRECTION ( 'NONE',  ( 0.000000000000000000, -0.9910827722268048534, 0.1332476588733589040 ) ) ;
#232320=ORIENTED_EDGE ( 'NONE', *, *, #224720, .F. ) ;
#232366=CARTESIAN_POINT ( 'NONE',  ( 11.60000000000006004, 64.35000000001120668, -23.62310748452479103 ) ) ;
#232412=CARTESIAN_POINT ( 'NONE',  ( 21.05000000000005400, 87.50449464844290048, -37.85861909827351468 ) ) ;
#232454=AXIS2_PLACEMENT_3D ( 'NONE', #209060, #64416, #143938 ) ;
#232529=CARTESIAN_POINT ( 'NONE',  ( 0.9000000000000547562, 67.65000000001118963, -10.02310748452479139 ) ) ;
#232579=EDGE_LOOP ( 'NONE', ( #230720, #229150, #203122, #175626, #83563, #69023, #37603 ) ) ;
#232601=CARTESIAN_POINT ( 'NONE',  ( 5.900000000000059863, 64.65000000001120384, -25.92310748452479174 ) ) ;
#232670=AXIS2_PLACEMENT_3D ( 'NONE', #232208, #53550, #150104 ) ;
#232676=AXIS2_PLACEMENT_3D ( 'NONE', #65153, #156913, #165563 ) ;
#232717=ADVANCED_FACE ( 'NONE', ( #36155 ), #178743, .T. ) ;
#232800=CIRCLE ( 'NONE', #120386, 0.1000000000000021844 ) ;
#232837=DIRECTION ( 'NONE',  ( 1.000000000000000000, 0.000000000000000000, 0.000000000000000000 ) ) ;
#232857=FACE_OUTER_BOUND ( 'NONE', #247109, .T. ) ;
#232858=CARTESIAN_POINT ( 'NONE',  ( 11.60000000000006004, 63.75000000001119815, -21.02310748452479316 ) ) ;
#232903=ORIENTED_EDGE ( 'NONE', *, *, #120573, .T. ) ;
#232914=LINE ( 'NONE', #251144, #90103 ) ;
#232928=EDGE_LOOP ( 'NONE', ( #19891, #115515, #141002, #215284 ) ) ;
#232944=EDGE_LOOP ( 'NONE', ( #165749, #173470, #21531, #111648 ) ) ;
#232955=DIRECTION ( 'NONE',  ( 0.000000000000000000, 0.000000000000000000, 1.000000000000000000 ) ) ;
#233012=DIRECTION ( 'NONE',  ( 0.000000000000000000, 0.000000000000000000, 1.000000000000000000 ) ) ;
#233100=ORIENTED_EDGE ( 'NONE', *, *, #157839, .F. ) ;
#233213=CARTESIAN_POINT ( 'NONE',  ( -20.94999999999994600, 66.25000000001119815, -5.923107484524795296 ) ) ;
#233275=DIRECTION ( 'NONE',  ( -1.000000000000000000, -0.000000000000000000, -0.000000000000000000 ) ) ;
#233278=ORIENTED_EDGE ( 'NONE', *, *, #246286, .T. ) ;
#233328=CARTESIAN_POINT ( 'NONE',  ( 23.40000000000005187, 77.25000000001119815, -43.92310748452479885 ) ) ;
#233329=EDGE_CURVE ( 'NONE', #201937, #96904, #132056, .T. ) ;
#233339=ORIENTED_EDGE ( 'NONE', *, *, #106728, .F. ) ;
#233356=CARTESIAN_POINT ( 'NONE',  ( 21.15000000000005187, 76.00000000001119815, -31.97310748452479601 ) ) ;
#233362=EDGE_CURVE ( 'NONE', #118259, #197543, #29267, .T. ) ;
#233423=CIRCLE ( 'NONE', #25303, 0.09999999999999939493 ) ;
#233446=AXIS2_PLACEMENT_3D ( 'NONE', #244477, #202787, #243190 ) ;
#233555=ORIENTED_EDGE ( 'NONE', *, *, #61233, .T. ) ;
#233596=ORIENTED_EDGE ( 'NONE', *, *, #125405, .F. ) ;
#233658=ORIENTED_EDGE ( 'NONE', *, *, #234929, .T. ) ;
#233709=AXIS2_PLACEMENT_3D ( 'NONE', #244412, #124487, #85316 ) ;
#233734=CARTESIAN_POINT ( 'NONE',  ( -23.39999999999994529, 87.50449464844290048, -37.85861909827351468 ) ) ;
#233743=CIRCLE ( 'NONE', #229638, 0.09999999999999939493 ) ;
#233762=EDGE_LOOP ( 'NONE', ( #114460, #61967, #47887, #160007 ) ) ;
#233795=EDGE_LOOP ( 'NONE', ( #8835, #8469, #190997, #11841 ) ) ;
#233875=CARTESIAN_POINT ( 'NONE',  ( -13.39999999999994351, 67.75000000001118394, -18.42310748452479174 ) ) ;
#233916=ADVANCED_FACE ( 'NONE', ( #37479 ), #217363, .F. ) ;
#233996=DIRECTION ( 'NONE',  ( 0.000000000000000000, 0.000000000000000000, -1.000000000000000000 ) ) ;
#233997=TOROIDAL_SURFACE ( 'NONE', #242375, 0.2000000000000000111, 0.1000000000000000056 ) ;
#234028=ORIENTED_EDGE ( 'NONE', *, *, #68912, .F. ) ;
#234036=CARTESIAN_POINT ( 'NONE',  ( -13.39999999999994351, 66.35000000001119247, -18.42310748452479174 ) ) ;
#234113=AXIS2_PLACEMENT_3D ( 'NONE', #241865, #125766, #25411 ) ;
#234116=EDGE_LOOP ( 'NONE', ( #177533, #152687, #113963, #129806 ) ) ;
#234147=DIRECTION ( 'NONE',  ( 1.000000000000000000, -0.000000000000000000, -0.000000000000000000 ) ) ;
#234155=ORIENTED_EDGE ( 'NONE', *, *, #62349, .F. ) ;
#234340=EDGE_CURVE ( 'NONE', #61312, #73109, #256130, .T. ) ;
#234380=CIRCLE ( 'NONE', #101048, 0.1000000000000032391 ) ;
#234395=ORIENTED_EDGE ( 'NONE', *, *, #196051, .T. ) ;
#234433=ORIENTED_EDGE ( 'NONE', *, *, #2812, .T. ) ;
#234566=DIRECTION ( 'NONE',  ( 0.000000000000000000, 0.000000000000000000, 1.000000000000000000 ) ) ;
#234589=ORIENTED_EDGE ( 'NONE', *, *, #38735, .T. ) ;
#234611=DIRECTION ( 'NONE',  ( 1.284434275755705789E-16, -0.7071067811865472397, -0.7071067811865479058 ) ) ;
#234616=EDGE_CURVE ( 'NONE', #168532, #117140, #83883, .T. ) ;
#234666=FACE_OUTER_BOUND ( 'NONE', #8462, .T. ) ;
#234673=DIRECTION ( 'NONE',  ( 1.000000000000000000, 0.000000000000000000, 0.000000000000000000 ) ) ;
#234699=EDGE_CURVE ( 'NONE', #128131, #40157, #70277, .T. ) ;
#234749=CYLINDRICAL_SURFACE ( 'NONE', #114134, 0.09999999999999850675 ) ;
#234760=VECTOR ( 'NONE', #32820, 1000.000000000000114 ) ;
#234836=VERTEX_POINT ( 'NONE', #76318 ) ;
#234884=EDGE_CURVE ( 'NONE', #103754, #81962, #250700, .T. ) ;
#234917=ORIENTED_EDGE ( 'NONE', *, *, #167214, .F. ) ;
#234929=EDGE_CURVE ( 'NONE', #60123, #139562, #204910, .T. ) ;
#234931=CIRCLE ( 'NONE', #122515, 0.1000000000000016709 ) ;
#235000=EDGE_CURVE ( 'NONE', #58156, #81962, #46198, .T. ) ;
#235066=EDGE_LOOP ( 'NONE', ( #130064, #220403, #195090, #170725 ) ) ;
#235069=DIRECTION ( 'NONE',  ( -1.000000000000000000, -0.000000000000000000, -0.000000000000000000 ) ) ;
#235129=AXIS2_PLACEMENT_3D ( 'NONE', #28655, #70329, #229380 ) ;
#235227=CARTESIAN_POINT ( 'NONE',  ( -21.04999999999994387, 82.84256550613280012, -26.34830530078816935 ) ) ;
#235245=ORIENTED_EDGE ( 'NONE', *, *, #51549, .T. ) ;
#235278=ORIENTED_EDGE ( 'NONE', *, *, #242143, .T. ) ;
#235317=EDGE_CURVE ( 'NONE', #34352, #74170, #163293, .T. ) ;
#235335=VERTEX_POINT ( 'NONE', #82425 ) ;
#235373=VECTOR ( 'NONE', #5035, 1000.000000000000000 ) ;
#235389=DIRECTION ( 'NONE',  ( 1.000000000000000000, 0.000000000000000000, 0.000000000000000000 ) ) ;
#235400=DIRECTION ( 'NONE',  ( 0.000000000000000000, -0.9910827722268048534, -0.1332476588733589040 ) ) ;
#235430=ORIENTED_EDGE ( 'NONE', *, *, #72982, .F. ) ;
#235454=EDGE_CURVE ( 'NONE', #243775, #33512, #25310, .T. ) ;
#235479=ORIENTED_EDGE ( 'NONE', *, *, #239062, .F. ) ;
#235505=EDGE_CURVE ( 'NONE', #62001, #230912, #251801, .T. ) ;
#235522=PLANE ( 'NONE',  #72218 ) ;
#235560=AXIS2_PLACEMENT_3D ( 'NONE', #12981, #112068, #254113 ) ;
#235564=ORIENTED_EDGE ( 'NONE', *, *, #245727, .F. ) ;
#235737=AXIS2_PLACEMENT_3D ( 'NONE', #25299, #146490, #143934 ) ;
#235761=CARTESIAN_POINT ( 'NONE',  ( -21.04999999999994387, 66.15000000001120384, -4.623107484524796362 ) ) ;
#235818=LINE ( 'NONE', #157617, #150450 ) ;
#235877=CARTESIAN_POINT ( 'NONE',  ( 20.95000000000005258, 64.35000000001120668, -30.12310748452479103 ) ) ;
#235939=DIRECTION ( 'NONE',  ( 0.000000000000000000, 0.000000000000000000, -1.000000000000000000 ) ) ;
#235973=EDGE_CURVE ( 'NONE', #207750, #224041, #130248, .T. ) ;
#235976=ORIENTED_EDGE ( 'NONE', *, *, #176658, .T. ) ;
#236129=EDGE_LOOP ( 'NONE', ( #257915, #243165, #87045, #130972 ) ) ;
#236203=CARTESIAN_POINT ( 'NONE',  ( 23.40000000000005187, 74.14873292176677921, -47.62635315998165453 ) ) ;
#236348=CIRCLE ( 'NONE', #69764, 11.74999999999999645 ) ;
#236443=ORIENTED_EDGE ( 'NONE', *, *, #217147, .F. ) ;
#236510=ADVANCED_FACE ( 'NONE', ( #88898 ), #126755, .T. ) ;
#236566=EDGE_CURVE ( 'NONE', #514, #251797, #37956, .T. ) ;
#236576=CARTESIAN_POINT ( 'NONE',  ( -21.04999999999994387, 76.00000000001119815, -36.02310748452479316 ) ) ;
#236637=CIRCLE ( 'NONE', #11824, 0.1000000000000002554 ) ;
#236714=AXIS2_PLACEMENT_3D ( 'NONE', #60819, #145498, #103784 ) ;
#236721=AXIS2_PLACEMENT_3D ( 'NONE', #163238, #227042, #202351 ) ;
#236733=CARTESIAN_POINT ( 'NONE',  ( 23.40000000000005187, 76.00000000001119815, -31.97310748452479601 ) ) ;
#236807=FACE_OUTER_BOUND ( 'NONE', #60974, .T. ) ;
#236841=ORIENTED_EDGE ( 'NONE', *, *, #177797, .T. ) ;
#236855=DIRECTION ( 'NONE',  ( 1.000000000000000000, 0.000000000000000000, 0.000000000000000000 ) ) ;
#236881=EDGE_CURVE ( 'NONE', #135540, #34933, #64446, .T. ) ;
#236933=CARTESIAN_POINT ( 'NONE',  ( -23.49999999999994316, 76.00000000001119815, -40.17310748452479174 ) ) ;
#236943=FACE_OUTER_BOUND ( 'NONE', #201424, .T. ) ;
#236988=DIRECTION ( 'NONE',  ( 1.000000000000000000, 0.000000000000000000, 0.000000000000000000 ) ) ;
#236998=CARTESIAN_POINT ( 'NONE',  ( 21.05000000000005400, 66.25000000001119815, -4.623107484524796362 ) ) ;
#237000=CIRCLE ( 'NONE', #220441, 0.1999999999999987899 ) ;
#237032=CARTESIAN_POINT ( 'NONE',  ( -23.49999999999994316, 74.16448838626247664, -47.52760213295649550 ) ) ;
#237074=EDGE_CURVE ( 'NONE', #109860, #80961, #181347, .T. ) ;
#237079=CYLINDRICAL_SURFACE ( 'NONE', #46299, 0.09999999999999530098 ) ;
#237126=ADVANCED_FACE ( 'NONE', ( #180994 ), #18052, .T. ) ;
#237127=LINE ( 'NONE', #19367, #66857 ) ;
#237132=VECTOR ( 'NONE', #23100, 1000.000000000000000 ) ;
#237220=CARTESIAN_POINT ( 'NONE',  ( -23.49999999999994316, 76.00000000001119815, -40.07310748452479032 ) ) ;
#237244=CARTESIAN_POINT ( 'NONE',  ( 21.15000000000005542, 77.83551161375991967, -47.52760213295649550 ) ) ;
#237315=VECTOR ( 'NONE', #193071, 1000.000000000000000 ) ;
#237339=VECTOR ( 'NONE', #152404, 1000.000000000000000 ) ;
#237413=CIRCLE ( 'NONE', #8457, 0.1000000000000002554 ) ;
#237431=DIRECTION ( 'NONE',  ( -1.000000000000000000, 0.000000000000000000, 0.000000000000000000 ) ) ;
#237442=VECTOR ( 'NONE', #23050, 1000.000000000000000 ) ;
#237489=ORIENTED_EDGE ( 'NONE', *, *, #189678, .T. ) ;
#237526=ORIENTED_EDGE ( 'NONE', *, *, #193481, .F. ) ;
#237535=DIRECTION ( 'NONE',  ( 0.000000000000000000, 0.000000000000000000, -1.000000000000000000 ) ) ;
#237543=CARTESIAN_POINT ( 'NONE',  ( -23.49999999999994316, 87.50449464844290048, -37.85861909827351468 ) ) ;
#237567=VECTOR ( 'NONE', #75289, 1000.000000000000114 ) ;
#237583=DIRECTION ( 'NONE',  ( 0.000000000000000000, 0.000000000000000000, -1.000000000000000000 ) ) ;
#237598=ORIENTED_EDGE ( 'NONE', *, *, #214755, .F. ) ;
#237656=DIRECTION ( 'NONE',  ( 0.000000000000000000, -0.9875102702516471709, 0.1575546449569757979 ) ) ;
#237700=AXIS2_PLACEMENT_3D ( 'NONE', #211566, #258019, #18179 ) ;
#237733=VECTOR ( 'NONE', #69836, 1000.000000000000000 ) ;
#237791=CIRCLE ( 'NONE', #133725, 4.041421356237306917 ) ;
#237793=AXIS2_PLACEMENT_3D ( 'NONE', #152603, #250382, #234673 ) ;
#237860=ADVANCED_FACE ( 'NONE', ( #125404 ), #65417, .F. ) ;
#237928=DIRECTION ( 'NONE',  ( 1.000000000000000000, 0.000000000000000000, 0.000000000000000000 ) ) ;
#238000=ORIENTED_EDGE ( 'NONE', *, *, #107280, .T. ) ;
#238006=DIRECTION ( 'NONE',  ( -1.000000000000000000, 0.000000000000000000, 0.000000000000000000 ) ) ;
#238084=EDGE_LOOP ( 'NONE', ( #22615, #141525, #76436, #247268 ) ) ;
#238089=CARTESIAN_POINT ( 'NONE',  ( -23.49999999999994316, 64.25000000001119815, -51.02310748452479316 ) ) ;
#238102=AXIS2_PLACEMENT_3D ( 'NONE', #117272, #58552, #37752 ) ;
#238141=ORIENTED_EDGE ( 'NONE', *, *, #35042, .F. ) ;
#238283=EDGE_LOOP ( 'NONE', ( #58623, #32566, #50531, #105281 ) ) ;
#238300=EDGE_CURVE ( 'NONE', #230635, #514, #52679, .T. ) ;
#238345=ORIENTED_EDGE ( 'NONE', *, *, #254559, .F. ) ;
#238360=DIRECTION ( 'NONE',  ( 0.000000000000000000, -0.1332476588733650935, 0.9910827722268042983 ) ) ;
#238386=CARTESIAN_POINT ( 'NONE',  ( -21.14999999999994174, 67.75000000001118394, -43.82310748452479743 ) ) ;
#238440=VERTEX_POINT ( 'NONE', #99349 ) ;
#238457=DIRECTION ( 'NONE',  ( -0.000000000000000000, 1.000000000000000000, -0.000000000000000000 ) ) ;
#238516=ORIENTED_EDGE ( 'NONE', *, *, #66157, .T. ) ;
#238521=CARTESIAN_POINT ( 'NONE',  ( -6.099999999999939249, 64.25000000001119815, -22.12310748452479103 ) ) ;
#238541=ORIENTED_EDGE ( 'NONE', *, *, #108446, .F. ) ;
#238646=CARTESIAN_POINT ( 'NONE',  ( -23.49999999999994316, 83.90000000001120384, -37.27310748452479316 ) ) ;
#238727=AXIS2_PLACEMENT_3D ( 'NONE', #88811, #115780, #168431 ) ;
#238761=ORIENTED_EDGE ( 'NONE', *, *, #150792, .T. ) ;
#238784=ORIENTED_EDGE ( 'NONE', *, *, #171891, .T. ) ;
#238802=CIRCLE ( 'NONE', #155625, 0.09999999999999939493 ) ;
#238807=EDGE_LOOP ( 'NONE', ( #239782, #115922, #118917, #33161 ) ) ;
#238819=DIRECTION ( 'NONE',  ( 0.000000000000000000, -0.5774316882803290918, -0.8164390028469542537 ) ) ;
#238821=VERTEX_POINT ( 'NONE', #92639 ) ;
#238827=FACE_OUTER_BOUND ( 'NONE', #222671, .T. ) ;
#238854=CARTESIAN_POINT ( 'NONE',  ( -11.59999999999994458, 66.35000000001119247, -21.02310748452479316 ) ) ;
#238861=CIRCLE ( 'NONE', #209636, 0.09999999999999982514 ) ;
#238937=AXIS2_PLACEMENT_3D ( 'NONE', #106416, #185980, #107723 ) ;
#238942=EDGE_CURVE ( 'NONE', #167224, #99338, #244404, .T. ) ;
#238965=CIRCLE ( 'NONE', #209728, 0.09999999999999939493 ) ;
#239062=EDGE_CURVE ( 'NONE', #202553, #62001, #161411, .T. ) ;
#239093=DIRECTION ( 'NONE',  ( 0.000000000000000000, 0.000000000000000000, -1.000000000000000000 ) ) ;
#239117=CARTESIAN_POINT ( 'NONE',  ( -23.39999999999994529, 83.90000000001120384, -37.27310748452479316 ) ) ;
#239128=SPHERICAL_SURFACE ( 'NONE', #4262, 0.1000000000000000056 ) ;
#239154=EDGE_CURVE ( 'NONE', #160549, #53673, #208465, .T. ) ;
#239205=CARTESIAN_POINT ( 'NONE',  ( -5.899999999999938183, 64.65000000001120384, -22.02310748452479316 ) ) ;
#239259=AXIS2_PLACEMENT_3D ( 'NONE', #102971, #5137, #44312 ) ;
#239284=CIRCLE ( 'NONE', #118499, 0.09999999999999982514 ) ;
#239328=EDGE_CURVE ( 'NONE', #150150, #90293, #40105, .T. ) ;
#239372=CARTESIAN_POINT ( 'NONE',  ( -21.14999999999994174, 83.80000000001119531, -51.02310748452479316 ) ) ;
#239395=DIRECTION ( 'NONE',  ( 1.000000000000000000, -0.000000000000000000, -0.000000000000000000 ) ) ;
#239398=DIRECTION ( 'NONE',  ( 1.000000000000000000, 0.000000000000000000, 0.000000000000000000 ) ) ;
#239409=AXIS2_PLACEMENT_3D ( 'NONE', #75827, #58800, #256974 ) ;
#239416=CARTESIAN_POINT ( 'NONE',  ( -21.14999999999994174, 65.15000000001120384, -3.023107484524792277 ) ) ;
#239441=CIRCLE ( 'NONE', #127014, 0.1000000000000028644 ) ;
#239496=VERTEX_POINT ( 'NONE', #130841 ) ;
#239506=EDGE_CURVE ( 'NONE', #256542, #106794, #170021, .T. ) ;
#239648=CARTESIAN_POINT ( 'NONE',  ( 21.15000000000005187, 76.00000000001119815, -36.02310748452479316 ) ) ;
#239651=AXIS2_PLACEMENT_3D ( 'NONE', #3263, #684, #121955 ) ;
#239698=CARTESIAN_POINT ( 'NONE',  ( -21.14999999999994174, 76.00000000001119815, -36.02310748452479316 ) ) ;
#239704=CARTESIAN_POINT ( 'NONE',  ( 23.40000000000005187, 76.00000000001119815, -36.02310748452479316 ) ) ;
#239774=CARTESIAN_POINT ( 'NONE',  ( -21.04999999999994387, 74.16448838626247664, -47.52760213295649550 ) ) ;
#239782=ORIENTED_EDGE ( 'NONE', *, *, #209906, .T. ) ;
#239909=CIRCLE ( 'NONE', #77548, 0.1999999999999987899 ) ;
#239959=DIRECTION ( 'NONE',  ( 0.000000000000000000, 0.000000000000000000, -1.000000000000000000 ) ) ;
#239971=PLANE ( 'NONE',  #90650 ) ;
#240069=CARTESIAN_POINT ( 'NONE',  ( -0.8999999999999437339, 64.25000000001119815, -12.72310748452478890 ) ) ;
#240082=DIRECTION ( 'NONE',  ( 0.000000000000000000, 0.000000000000000000, -1.000000000000000000 ) ) ;
#240083=LINE ( 'NONE', #39332, #94978 ) ;
#240084=DIRECTION ( 'NONE',  ( 0.000000000000000000, 0.000000000000000000, 1.000000000000000000 ) ) ;
#240175=AXIS2_PLACEMENT_3D ( 'NONE', #198732, #256076, #257359 ) ;
#240181=EDGE_LOOP ( 'NONE', ( #49833, #138323, #192849, #180801 ) ) ;
#240186=FACE_OUTER_BOUND ( 'NONE', #198482, .T. ) ;
#240203=FACE_OUTER_BOUND ( 'NONE', #2254, .T. ) ;
#240240=DIRECTION ( 'NONE',  ( 1.000000000000000000, -0.000000000000000000, -0.000000000000000000 ) ) ;
#240345=ORIENTED_EDGE ( 'NONE', *, *, #95561, .F. ) ;
#240519=DIRECTION ( 'NONE',  ( 0.000000000000000000, 0.000000000000000000, 1.000000000000000000 ) ) ;
#240543=AXIS2_PLACEMENT_3D ( 'NONE', #123693, #203215, #184936 ) ;
#240556=EDGE_LOOP ( 'NONE', ( #158142, #58370, #140248, #73919, #240345, #25532, #145053, #143103 ) ) ;
#240581=DIRECTION ( 'NONE',  ( -0.000000000000000000, 0.9910827722268049644, -0.1332476588733589318 ) ) ;
#240589=CARTESIAN_POINT ( 'NONE',  ( 21.15000000000005542, 89.48413628383013929, -38.12477508515532065 ) ) ;
#240602=CARTESIAN_POINT ( 'NONE',  ( 23.50000000000005684, 74.16448838626247664, -47.52760213295649550 ) ) ;
#240676=DIRECTION ( 'NONE',  ( -1.000000000000000000, 8.673617379884087537E-15, 0.000000000000000000 ) ) ;
#240703=EDGE_CURVE ( 'NONE', #133767, #36158, #144788, .T. ) ;
#240782=ORIENTED_EDGE ( 'NONE', *, *, #113053, .F. ) ;
#240885=PRODUCT_DEFINITION_CONTEXT ( 'detailed design', #255667, 'design' ) ;
#240922=ORIENTED_EDGE ( 'NONE', *, *, #24211, .F. ) ;
#240949=LINE ( 'NONE', #199261, #251722 ) ;
#241005=DIRECTION ( 'NONE',  ( 0.000000000000000000, 0.000000000000000000, 1.000000000000000000 ) ) ;
#241014=ADVANCED_FACE ( 'NONE', ( #125748 ), #226114, .T. ) ;
#241026=EDGE_CURVE ( 'NONE', #114442, #216036, #147907, .T. ) ;
#241090=AXIS2_PLACEMENT_3D ( 'NONE', #17470, #18753, #94435 ) ;
#241147=EDGE_LOOP ( 'NONE', ( #115725, #39369, #46770, #135208 ) ) ;
#241154=EDGE_LOOP ( 'NONE', ( #108972, #48660, #107814, #2069 ) ) ;
#241167=ADVANCED_FACE ( 'NONE', ( #176468 ), #36884, .T. ) ;
#241177=ORIENTED_EDGE ( 'NONE', *, *, #168710, .F. ) ;
#241184=AXIS2_PLACEMENT_3D ( 'NONE', #117628, #115063, #237583 ) ;
#241218=FACE_OUTER_BOUND ( 'NONE', #232928, .T. ) ;
#241222=CARTESIAN_POINT ( 'NONE',  ( -23.49999999999994316, 76.00000000001119815, -31.97310748452479601 ) ) ;
#241339=ADVANCED_FACE ( 'NONE', ( #6464 ), #85976, .T. ) ;
#241392=VERTEX_POINT ( 'NONE', #208544 ) ;
#241406=DIRECTION ( 'NONE',  ( 1.000000000000000000, 0.000000000000000000, 0.000000000000000000 ) ) ;
#241410=CARTESIAN_POINT ( 'NONE',  ( 21.15000000000005187, 64.25000000001119815, -51.02310748452479316 ) ) ;
#241417=LINE ( 'NONE', #178904, #60349 ) ;
#241436=DIRECTION ( 'NONE',  ( 1.000000000000000000, -0.000000000000000000, 0.000000000000000000 ) ) ;
#241471=CARTESIAN_POINT ( 'NONE',  ( 21.15000000000005187, 64.25000000001119815, -5.923107484524795296 ) ) ;
#241484=CARTESIAN_POINT ( 'NONE',  ( 21.15000000000005542, 74.73834681386826162, -44.00978271863746016 ) ) ;
#241498=ORIENTED_EDGE ( 'NONE', *, *, #152205, .T. ) ;
#241504=DIRECTION ( 'NONE',  ( 0.000000000000000000, -0.7071067811865479058, 0.7071067811865472397 ) ) ;
#241529=CARTESIAN_POINT ( 'NONE',  ( -21.14999999999994174, 77.83551161375991967, -47.52760213295649550 ) ) ;
#241580=DIRECTION ( 'NONE',  ( -0.000000000000000000, 0.000000000000000000, -1.000000000000000000 ) ) ;
#241634=ORIENTED_EDGE ( 'NONE', *, *, #83809, .F. ) ;
#241665=ORIENTED_EDGE ( 'NONE', *, *, #157087, .F. ) ;
#241704=CIRCLE ( 'NONE', #254160, 0.1000000000000028644 ) ;
#241709=DIRECTION ( 'NONE',  ( 0.000000000000000000, 0.000000000000000000, -1.000000000000000000 ) ) ;
#241728=CARTESIAN_POINT ( 'NONE',  ( 11.60000000000006004, 66.35000000001119247, -21.02310748452479316 ) ) ;
#241742=FACE_OUTER_BOUND ( 'NONE', #153959, .T. ) ;
#241808=DIRECTION ( 'NONE',  ( 0.000000000000000000, 0.000000000000000000, 1.000000000000000000 ) ) ;
#241862=CIRCLE ( 'NONE', #116976, 0.09999999999999530098 ) ;
#241865=CARTESIAN_POINT ( 'NONE',  ( -20.94999999999994600, 64.35000000001120668, -29.92310748452479174 ) ) ;
#241884=ORIENTED_EDGE ( 'NONE', *, *, #71196, .F. ) ;
#242056=DIRECTION ( 'NONE',  ( 0.000000000000000000, -0.1480365673253065117, 0.9889818879709273425 ) ) ;
#242066=LINE ( 'NONE', #218647, #229461 ) ;
#242076=EDGE_CURVE ( 'NONE', #238821, #11972, #36896, .T. ) ;
#242083=DIRECTION ( 'NONE',  ( -0.000000000000000000, 0.000000000000000000, 1.000000000000000000 ) ) ;
#242097=TOROIDAL_SURFACE ( 'NONE', #100434, 0.2000000000000000111, 0.1000000000000000056 ) ;
#242100=DIRECTION ( 'NONE',  ( 0.000000000000000000, 1.000000000000000000, 0.000000000000000000 ) ) ;
#242141=AXIS2_PLACEMENT_3D ( 'NONE', #174795, #155215, #156504 ) ;
#242143=EDGE_CURVE ( 'NONE', #136469, #184662, #166421, .T. ) ;
#242153=DIRECTION ( 'NONE',  ( 1.000000000000000000, -0.000000000000000000, -0.000000000000000000 ) ) ;
#242175=DIRECTION ( 'NONE',  ( 0.000000000000000000, 0.000000000000000000, -1.000000000000000000 ) ) ;
#242263=EDGE_CURVE ( 'NONE', #104351, #176509, #172259, .T. ) ;
#242270=AXIS2_PLACEMENT_3D ( 'NONE', #216605, #217865, #116245 ) ;
#242276=ORIENTED_EDGE ( 'NONE', *, *, #253187, .F. ) ;
#242302=EDGE_CURVE ( 'NONE', #168923, #122992, #113520, .T. ) ;
#242336=AXIS2_PLACEMENT_3D ( 'NONE', #152277, #94834, #36173 ) ;
#242368=CYLINDRICAL_SURFACE ( 'NONE', #162694, 0.09999999999999939493 ) ;
#242375=AXIS2_PLACEMENT_3D ( 'NONE', #147773, #227292, #128206 ) ;
#242386=ORIENTED_EDGE ( 'NONE', *, *, #157124, .T. ) ;
#242390=PLANE ( 'NONE',  #179595 ) ;
#242393=AXIS2_PLACEMENT_3D ( 'NONE', #168757, #94289, #173888 ) ;
#242438=FACE_OUTER_BOUND ( 'NONE', #129044, .T. ) ;
#242463=CIRCLE ( 'NONE', #46632, 0.09999999999999939493 ) ;
#242471=ORIENTED_EDGE ( 'NONE', *, *, #181547, .T. ) ;
#242478=EDGE_CURVE ( 'NONE', #23626, #88201, #135637, .T. ) ;
#242490=EDGE_CURVE ( 'NONE', #99842, #90507, #174828, .T. ) ;
#242527=CIRCLE ( 'NONE', #109422, 4.900000000000000355 ) ;
#242608=ADVANCED_FACE ( 'NONE', ( #242438 ), #87208, .T. ) ;
#242629=DIRECTION ( 'NONE',  ( -1.000000000000000000, 0.000000000000000000, 0.000000000000000000 ) ) ;
#242672=DIRECTION ( 'NONE',  ( 0.000000000000000000, 0.000000000000000000, -1.000000000000000000 ) ) ;
#242696=AXIS2_PLACEMENT_3D ( 'NONE', #98864, #136729, #181021 ) ;
#242755=ORIENTED_EDGE ( 'NONE', *, *, #151864, .T. ) ;
#242767=CARTESIAN_POINT ( 'NONE',  ( 23.40000000000005542, 83.80000000001119531, -51.02310748452479316 ) ) ;
#242785=ADVANCED_FACE ( 'NONE', ( #168099 ), #209750, .T. ) ;
#242816=EDGE_CURVE ( 'NONE', #186991, #113855, #233423, .T. ) ;
#242817=AXIS2_PLACEMENT_3D ( 'NONE', #99574, #138689, #257333 ) ;
#242819=CARTESIAN_POINT ( 'NONE',  ( 20.95000000000005258, 65.19115966511134275, -29.92310748452479174 ) ) ;
#242866=VECTOR ( 'NONE', #44352, 1000.000000000000000 ) ;
#242898=EDGE_LOOP ( 'NONE', ( #21627, #219129, #78225, #142168 ) ) ;
#242907=ORIENTED_EDGE ( 'NONE', *, *, #249965, .F. ) ;
#242938=CYLINDRICAL_SURFACE ( 'NONE', #251790, 0.1000000000000002554 ) ;
#243028=CARTESIAN_POINT ( 'NONE',  ( -21.14999999999994174, 76.00000000001119815, -31.87310748452479459 ) ) ;
#243048=DIRECTION ( 'NONE',  ( 0.000000000000000000, 0.000000000000000000, -1.000000000000000000 ) ) ;
#243115=ORIENTED_EDGE ( 'NONE', *, *, #49272, .T. ) ;
#243165=ORIENTED_EDGE ( 'NONE', *, *, #246410, .F. ) ;
#243189=CYLINDRICAL_SURFACE ( 'NONE', #85438, 0.09999999999999939493 ) ;
#243190=DIRECTION ( 'NONE',  ( 0.000000000000000000, 0.000000000000000000, -1.000000000000000000 ) ) ;
#243205=DIRECTION ( 'NONE',  ( 0.000000000000000000, 0.000000000000000000, -1.000000000000000000 ) ) ;
#243210=CARTESIAN_POINT ( 'NONE',  ( 20.95000000000005258, 64.25000000001119815, -30.12310748452479103 ) ) ;
#243225=EDGE_CURVE ( 'NONE', #113073, #6953, #49063, .T. ) ;
#243237=CIRCLE ( 'NONE', #84413, 11.65000000000000036 ) ;
#243281=ORIENTED_EDGE ( 'NONE', *, *, #138533, .T. ) ;
#243288=ORIENTED_EDGE ( 'NONE', *, *, #30228, .F. ) ;
#243337=CARTESIAN_POINT ( 'NONE',  ( 11.60000000000006004, 64.25000000001119815, -18.32310748452479388 ) ) ;
#243365=DIRECTION ( 'NONE',  ( -1.000000000000000000, 0.000000000000000000, 0.000000000000000000 ) ) ;
#243397=CARTESIAN_POINT ( 'NONE',  ( -21.14999999999994174, 76.00000000001119815, -3.023107484524792277 ) ) ;
#243399=LINE ( 'NONE', #225099, #51970 ) ;
#243401=LINE ( 'NONE', #225100, #245519 ) ;
#243504=CARTESIAN_POINT ( 'NONE',  ( 23.40000000000005187, 76.00000000001119815, -36.02310748452479316 ) ) ;
#243570=CIRCLE ( 'NONE', #47923, 0.09999999999999939493 ) ;
#243588=CARTESIAN_POINT ( 'NONE',  ( -21.04999999999994387, 67.75000000001118394, -3.123107484524795474 ) ) ;
#243589=FACE_OUTER_BOUND ( 'NONE', #249357, .T. ) ;
#243599=DIRECTION ( 'NONE',  ( -1.000000000000000000, 0.000000000000000000, 0.000000000000000000 ) ) ;
#243617=AXIS2_PLACEMENT_3D ( 'NONE', #784, #255085, #56907 ) ;
#243618=EDGE_CURVE ( 'NONE', #1657, #131459, #229671, .T. ) ;
#243646=AXIS2_PLACEMENT_3D ( 'NONE', #216846, #17380, #194756 ) ;
#243656=DIRECTION ( 'NONE',  ( 0.000000000000000000, 0.000000000000000000, 1.000000000000000000 ) ) ;
#243670=ORIENTED_EDGE ( 'NONE', *, *, #109112, .T. ) ;
#243702=CARTESIAN_POINT ( 'NONE',  ( 11.60000000000006182, 64.35000000001120668, -23.72310748452479601 ) ) ;
#243740=AXIS2_PLACEMENT_3D ( 'NONE', #3598, #66146, #145670 ) ;
#243775=VERTEX_POINT ( 'NONE', #147237 ) ;
#243934=DIRECTION ( 'NONE',  ( 1.000000000000000000, 0.000000000000000000, -0.000000000000000000 ) ) ;
#243985=VERTEX_POINT ( 'NONE', #118395 ) ;
#244032=DIRECTION ( 'NONE',  ( 1.000000000000000000, -0.000000000000000000, -0.000000000000000000 ) ) ;
#244093=EDGE_CURVE ( 'NONE', #255703, #105984, #180928, .T. ) ;
#244193=AXIS2_PLACEMENT_3D ( 'NONE', #167586, #191002, #90576 ) ;
#244252=CARTESIAN_POINT ( 'NONE',  ( -5.899999999999938183, 64.75000000001119815, -22.12310748452479103 ) ) ;
#244271=ORIENTED_EDGE ( 'NONE', *, *, #45667, .T. ) ;
#244323=ORIENTED_EDGE ( 'NONE', *, *, #64134, .F. ) ;
#244404=CIRCLE ( 'NONE', #48775, 0.1000000000000032391 ) ;
#244412=CARTESIAN_POINT ( 'NONE',  ( 21.15000000000005187, 76.00000000001119815, -36.02310748452479316 ) ) ;
#244477=CARTESIAN_POINT ( 'NONE',  ( 13.40000000000005898, 64.25000000001119815, -21.02310748452479316 ) ) ;
#244489=TOROIDAL_SURFACE ( 'NONE', #152962, 0.2000000000000000111, 0.1000000000000000056 ) ;
#244493=ADVANCED_FACE ( 'NONE', ( #253716 ), #104887, .T. ) ;
#244498=EDGE_CURVE ( 'NONE', #98456, #66524, #21755, .T. ) ;
#244501=EDGE_CURVE ( 'NONE', #190938, #173155, #150918, .T. ) ;
#244614=DIRECTION ( 'NONE',  ( -0.000000000000000000, -0.1332476588733647882, -0.9910827722268041873 ) ) ;
#244710=FACE_OUTER_BOUND ( 'NONE', #217536, .T. ) ;
#244780=ADVANCED_FACE ( 'NONE', ( #206596 ), #130718, .T. ) ;
#244827=DIRECTION ( 'NONE',  ( -0.000000000000000000, -0.1332476588733656764, 0.9910827722268041873 ) ) ;
#244869=VERTEX_POINT ( 'NONE', #198579 ) ;
#244933=CARTESIAN_POINT ( 'NONE',  ( -21.14999999999994174, 74.94272479589878344, -8.023107484524793165 ) ) ;
#244937=DIRECTION ( 'NONE',  ( 0.000000000000000000, -0.000000000000000000, 1.000000000000000000 ) ) ;
#244964=VECTOR ( 'NONE', #193225, 1000.000000000000000 ) ;
#245155=DIRECTION ( 'NONE',  ( 0.000000000000000000, 0.000000000000000000, 1.000000000000000000 ) ) ;
#245169=CIRCLE ( 'NONE', #241090, 0.09999999999999939493 ) ;
#245268=AXIS2_PLACEMENT_3D ( 'NONE', #47747, #84268, #227678 ) ;
#245286=CARTESIAN_POINT ( 'NONE',  ( 23.40000000000005542, 77.83551161375991967, -47.52760213295649550 ) ) ;
#245288=DIRECTION ( 'NONE',  ( 0.000000000000000000, 0.000000000000000000, 1.000000000000000000 ) ) ;
#245294=DIRECTION ( 'NONE',  ( 0.000000000000000000, -0.8741572761215442577, 0.4856429311786202851 ) ) ;
#245311=ORIENTED_EDGE ( 'NONE', *, *, #137079, .F. ) ;
#245476=AXIS2_PLACEMENT_3D ( 'NONE', #237543, #172477, #133307 ) ;
#245509=DIRECTION ( 'NONE',  ( 0.000000000000000000, -1.000000000000000000, 0.000000000000000000 ) ) ;
#245519=VECTOR ( 'NONE', #187301, 1000.000000000000000 ) ;
#245541=SURFACE_STYLE_FILL_AREA ( #89008 ) ;
#245550=FACE_OUTER_BOUND ( 'NONE', #101565, .T. ) ;
#245626=CARTESIAN_POINT ( 'NONE',  ( -23.49999999999994316, 82.74366731733570646, -26.36310895752070138 ) ) ;
#245698=AXIS2_PLACEMENT_3D ( 'NONE', #146463, #190781, #12138 ) ;
#245713=LINE ( 'NONE', #85320, #40695 ) ;
#245727=EDGE_CURVE ( 'NONE', #5207, #3259, #241417, .T. ) ;
#245736=AXIS2_PLACEMENT_3D ( 'NONE', #104595, #86318, #25119 ) ;
#245787=ORIENTED_EDGE ( 'NONE', *, *, #169515, .F. ) ;
#245819=CIRCLE ( 'NONE', #200032, 4.900000000000000355 ) ;
#245850=DIRECTION ( 'NONE',  ( -0.000000000000000000, 0.000000000000000000, -1.000000000000000000 ) ) ;
#245872=CIRCLE ( 'NONE', #16937, 0.1000000000000028644 ) ;
#245924=PLANE ( 'NONE',  #1008 ) ;
#245957=FACE_OUTER_BOUND ( 'NONE', #196095, .T. ) ;
#245973=VERTEX_POINT ( 'NONE', #92589 ) ;
#245978=SPHERICAL_SURFACE ( 'NONE', #107731, 0.1000000000000000056 ) ;
#245988=DIRECTION ( 'NONE',  ( 0.000000000000000000, -0.9910827722268055195, 0.1332476588733540468 ) ) ;
#246022=AXIS2_PLACEMENT_3D ( 'NONE', #217357, #3454, #222486 ) ;
#246117=ORIENTED_EDGE ( 'NONE', *, *, #6134, .F. ) ;
#246175=CARTESIAN_POINT ( 'NONE',  ( -21.14999999999994174, 74.16448838626247664, -47.52760213295649550 ) ) ;
#246214=ORIENTED_EDGE ( 'NONE', *, *, #233362, .F. ) ;
#246229=LINE ( 'NONE', #205808, #181814 ) ;
#246286=EDGE_CURVE ( 'NONE', #1657, #202553, #226658, .T. ) ;
#246312=ORIENTED_EDGE ( 'NONE', *, *, #47048, .F. ) ;
#246327=EDGE_CURVE ( 'NONE', #51994, #205114, #93574, .T. ) ;
#246345=EDGE_CURVE ( 'NONE', #139324, #8217, #41465, .T. ) ;
#246366=CARTESIAN_POINT ( 'NONE',  ( -21.04999999999994387, 67.85000000001119247, -25.52310748452479316 ) ) ;
#246408=CIRCLE ( 'NONE', #217338, 0.1999999999999987899 ) ;
#246410=EDGE_CURVE ( 'NONE', #28434, #230635, #213513, .T. ) ;
#246452=CARTESIAN_POINT ( 'NONE',  ( -23.49999999999994316, 77.26165318615413469, -44.00978271863746016 ) ) ;
#246485=CARTESIAN_POINT ( 'NONE',  ( -23.39999999999994529, 83.88667523412387084, -34.67399920730211704 ) ) ;
#246498=ORIENTED_EDGE ( 'NONE', *, *, #121247, .F. ) ;
#246503=ADVANCED_FACE ( 'NONE', ( #119578 ), #20477, .T. ) ;
#246585=DIRECTION ( 'NONE',  ( 0.000000000000000000, 0.000000000000000000, 1.000000000000000000 ) ) ;
#246596=DIRECTION ( 'NONE',  ( 0.000000000000000000, 1.000000000000000000, -0.000000000000000000 ) ) ;
#246607=ORIENTED_EDGE ( 'NONE', *, *, #103123, .F. ) ;
#246613=EDGE_LOOP ( 'NONE', ( #160537, #101000, #212166, #40584 ) ) ;
#246668=EDGE_CURVE ( 'NONE', #151679, #165490, #222480, .T. ) ;
#246704=AXIS2_PLACEMENT_3D ( 'NONE', #76959, #58660, #97779 ) ;
#246797=DIRECTION ( 'NONE',  ( 1.000000000000000000, 0.000000000000000000, 0.000000000000000000 ) ) ;
#246806=AXIS2_PLACEMENT_3D ( 'NONE', #7234, #85462, #166363 ) ;
#246833=DIRECTION ( 'NONE',  ( 0.000000000000000000, 2.362176648138631684E-15, -1.000000000000000000 ) ) ;
#246885=DIRECTION ( 'NONE',  ( 0.000000000000000000, 0.000000000000000000, -1.000000000000000000 ) ) ;
#246892=FACE_OUTER_BOUND ( 'NONE', #36008, .T. ) ;
#246929=VECTOR ( 'NONE', #152215, 1000.000000000000000 ) ;
#246975=EDGE_CURVE ( 'NONE', #86047, #38614, #146031, .T. ) ;
#246986=CARTESIAN_POINT ( 'NONE',  ( -23.49999999999994316, 64.35000000001120668, -18.32310748452480098 ) ) ;
#246999=CARTESIAN_POINT ( 'NONE',  ( -23.49999999999994316, 76.00000000001119815, -36.02310748452479316 ) ) ;
#247102=PRODUCT ( 'Moving End Attachment Flange', 'Moving End Attachment Flange', '', ( #198151 ) ) ;
#247109=EDGE_LOOP ( 'NONE', ( #5681, #181374, #75799, #85060 ) ) ;
#247232=DIRECTION ( 'NONE',  ( -0.000000000000000000, -1.000000000000000000, 0.000000000000000000 ) ) ;
#247236=DIRECTION ( 'NONE',  ( 0.000000000000000000, -0.5774316882803290918, -0.8164390028469542537 ) ) ;
#247268=ORIENTED_EDGE ( 'NONE', *, *, #27624, .F. ) ;
#247460=LINE ( 'NONE', #31021, #98177 ) ;
#247498=CIRCLE ( 'NONE', #55924, 11.65000000000000036 ) ;
#247545=ORIENTED_EDGE ( 'NONE', *, *, #2289, .T. ) ;
#247589=ORIENTED_EDGE ( 'NONE', *, *, #159184, .T. ) ;
#247597=DIRECTION ( 'NONE',  ( 1.000000000000000000, 0.000000000000000000, 0.000000000000000000 ) ) ;
#247672=EDGE_CURVE ( 'NONE', #112788, #187434, #67297, .T. ) ;
#247697=AXIS2_PLACEMENT_3D ( 'NONE', #107902, #147018, #192584 ) ;
#247735=ORIENTED_EDGE ( 'NONE', *, *, #44029, .F. ) ;
#247782=AXIS2_PLACEMENT_3D ( 'NONE', #64926, #223998, #45370 ) ;
#247863=CARTESIAN_POINT ( 'NONE',  ( 21.15000000000005187, 82.84256550613280012, -26.34830530078816935 ) ) ;
#247875=DIRECTION ( 'NONE',  ( 1.000000000000000000, 0.000000000000000000, 0.000000000000000000 ) ) ;
#247912=LINE ( 'NONE', #186680, #190442 ) ;
#247924=DIRECTION ( 'NONE',  ( -0.000000000000000000, 0.1480365673253065117, -0.9889818879709273425 ) ) ;
#247954=AXIS2_PLACEMENT_3D ( 'NONE', #33821, #113307, #74223 ) ;
#247965=ORIENTED_EDGE ( 'NONE', *, *, #156519, .T. ) ;
#247980=EDGE_LOOP ( 'NONE', ( #255686, #101324, #68006, #128854 ) ) ;
#248009=VECTOR ( 'NONE', #71003, 1000.000000000000000 ) ;
#248115=CARTESIAN_POINT ( 'NONE',  ( 20.95000000000005613, 66.15000000001120384, -5.923107484524795296 ) ) ;
#248124=CARTESIAN_POINT ( 'NONE',  ( -21.14999999999994174, 76.00000000001119815, -36.02310748452479316 ) ) ;
#248165=DIRECTION ( 'NONE',  ( 1.000000000000000000, 0.000000000000000000, 0.000000000000000000 ) ) ;
#248196=DIRECTION ( 'NONE',  ( -1.000000000000000000, 0.000000000000000000, 0.000000000000000000 ) ) ;
#248225=FACE_OUTER_BOUND ( 'NONE', #251103, .T. ) ;
#248236=VERTEX_POINT ( 'NONE', #41062 ) ;
#248256=AXIS2_PLACEMENT_3D ( 'NONE', #145952, #130237, #204636 ) ;
#248276=DIRECTION ( 'NONE',  ( 1.000000000000000000, 0.000000000000000000, 0.000000000000000000 ) ) ;
#248284=DIRECTION ( 'NONE',  ( 1.000000000000000000, 0.000000000000000000, 0.000000000000000000 ) ) ;
#248294=CARTESIAN_POINT ( 'NONE',  ( -21.14999999999994174, 74.16448838626247664, -47.52760213295649550 ) ) ;
#248382=AXIS2_PLACEMENT_3D ( 'NONE', #122290, #86976, #27066 ) ;
#248493=AXIS2_PLACEMENT_3D ( 'NONE', #148671, #46970, #69143 ) ;
#248495=ORIENTED_EDGE ( 'NONE', *, *, #98773, .F. ) ;
#248511=DIRECTION ( 'NONE',  ( 0.000000000000000000, 0.000000000000000000, 1.000000000000000000 ) ) ;
#248520=AXIS2_PLACEMENT_3D ( 'NONE', #163934, #49104, #223880 ) ;
#248568=EDGE_CURVE ( 'NONE', #169843, #23611, #225762, .T. ) ;
#248628=ORIENTED_EDGE ( 'NONE', *, *, #238942, .F. ) ;
#248633=ADVANCED_FACE ( 'NONE', ( #124133 ), #105807, .T. ) ;
#248706=ORIENTED_EDGE ( 'NONE', *, *, #45667, .F. ) ;
#248783=DIRECTION ( 'NONE',  ( -0.000000000000000000, 0.1332476588733589040, 0.9910827722268049644 ) ) ;
#248895=VECTOR ( 'NONE', #61325, 1000.000000000000114 ) ;
#249118=DIRECTION ( 'NONE',  ( 0.000000000000000000, 1.000000000000000000, 0.000000000000000000 ) ) ;
#249137=EDGE_CURVE ( 'NONE', #211183, #15261, #789, .T. ) ;
#249180=FACE_OUTER_BOUND ( 'NONE', #161298, .T. ) ;
#249202=LINE ( 'NONE', #169701, #159552 ) ;
#249282=VERTEX_POINT ( 'NONE', #23074 ) ;
#249297=TOROIDAL_SURFACE ( 'NONE', #28575, 0.2000000000000000111, 0.1000000000000000056 ) ;
#249340=ORIENTED_EDGE ( 'NONE', *, *, #70480, .F. ) ;
#249357=EDGE_LOOP ( 'NONE', ( #153843, #219646, #197245, #170599 ) ) ;
#249383=CARTESIAN_POINT ( 'NONE',  ( 21.05000000000005400, 78.47315729244128590, -52.27034697567518862 ) ) ;
#249411=PLANE ( 'NONE',  #156543 ) ;
#249434=LINE ( 'NONE', #172506, #77833 ) ;
#249501=CARTESIAN_POINT ( 'NONE',  ( -5.999999999999938716, 64.75000000001119815, -26.02310748452479316 ) ) ;
#249515=DIRECTION ( 'NONE',  ( -1.000000000000000000, 0.000000000000000000, -0.000000000000000000 ) ) ;
#249539=VERTEX_POINT ( 'NONE', #256144 ) ;
#249561=EDGE_CURVE ( 'NONE', #218111, #10047, #77549, .T. ) ;
#249622=CARTESIAN_POINT ( 'NONE',  ( -5.899999999999938183, 64.25000000001119815, -26.02310748452479316 ) ) ;
#249638=DIRECTION ( 'NONE',  ( -1.000000000000000000, 0.000000000000000000, 0.000000000000000000 ) ) ;
#249676=CARTESIAN_POINT ( 'NONE',  ( 23.40000000000005187, 74.16448838626247664, -47.62760213295649692 ) ) ;
#249695=DIRECTION ( 'NONE',  ( 0.000000000000000000, 0.9889818879709272315, 0.1480365673253073999 ) ) ;
#249805=VERTEX_POINT ( 'NONE', #112566 ) ;
#249879=ORIENTED_EDGE ( 'NONE', *, *, #246327, .T. ) ;
#249930=LINE ( 'NONE', #149568, #97050 ) ;
#249944=CARTESIAN_POINT ( 'NONE',  ( -23.39999999999994529, 83.98667523412385094, -37.28476067066772970 ) ) ;
#249953=CARTESIAN_POINT ( 'NONE',  ( -0.8999999999999430678, 63.75000000001118394, -10.02310748452479139 ) ) ;
#249965=EDGE_CURVE ( 'NONE', #170630, #126736, #25030, .T. ) ;
#249969=EDGE_LOOP ( 'NONE', ( #128431, #227002, #200176, #245787 ) ) ;
#250091=DIRECTION ( 'NONE',  ( -0.000000000000000000, -0.000000000000000000, -1.000000000000000000 ) ) ;
#250132=ORIENTED_EDGE ( 'NONE', *, *, #17355, .T. ) ;
#250135=ORIENTED_EDGE ( 'NONE', *, *, #223678, .T. ) ;
#250152=CIRCLE ( 'NONE', #187626, 2.700000000000001066 ) ;
#250175=VERTEX_POINT ( 'NONE', #251753 ) ;
#250178=LINE ( 'NONE', #118373, #128968 ) ;
#250204=EDGE_LOOP ( 'NONE', ( #85304, #161172, #34576, #160556 ) ) ;
#250244=EDGE_CURVE ( 'NONE', #104351, #169843, #213569, .T. ) ;
#250278=ORIENTED_EDGE ( 'NONE', *, *, #193118, .T. ) ;
#250283=CARTESIAN_POINT ( 'NONE',  ( 23.40000000000005542, 74.83745509109094485, -43.82310748452479743 ) ) ;
#250366=ORIENTED_EDGE ( 'NONE', *, *, #77710, .T. ) ;
#250382=DIRECTION ( 'NONE',  ( 0.000000000000000000, 1.000000000000000000, 0.000000000000000000 ) ) ;
#250515=CIRCLE ( 'NONE', #117257, 0.09999999999999939493 ) ;
#250544=ORIENTED_EDGE ( 'NONE', *, *, #112734, .F. ) ;
#250558=EDGE_CURVE ( 'NONE', #150745, #235335, #68020, .T. ) ;
#250560=CYLINDRICAL_SURFACE ( 'NONE', #131132, 0.09999999999999530098 ) ;
#250700=CIRCLE ( 'NONE', #54878, 0.1000000000000002554 ) ;
#250717=DIRECTION ( 'NONE',  ( 0.000000000000000000, 0.000000000000000000, -1.000000000000000000 ) ) ;
#250742=DIRECTION ( 'NONE',  ( 0.000000000000000000, 1.000000000000000000, 0.000000000000000000 ) ) ;
#250761=ORIENTED_EDGE ( 'NONE', *, *, #24991, .F. ) ;
#250769=EDGE_CURVE ( 'NONE', #192885, #141859, #122204, .T. ) ;
#250815=DIRECTION ( 'NONE',  ( 0.000000000000000000, 0.000000000000000000, -1.000000000000000000 ) ) ;
#250885=CIRCLE ( 'NONE', #146828, 0.09999999999999530098 ) ;
#250893=FACE_OUTER_BOUND ( 'NONE', #104775, .T. ) ;
#250953=CARTESIAN_POINT ( 'NONE',  ( 23.40000000000005187, 77.85126707825561709, -47.62635315998165453 ) ) ;
#250956=VECTOR ( 'NONE', #12912, 1000.000000000000000 ) ;
#250965=AXIS2_PLACEMENT_3D ( 'NONE', #135137, #98551, #178162 ) ;
#250977=DIRECTION ( 'NONE',  ( 1.000000000000000000, 0.000000000000000000, 0.000000000000000000 ) ) ;
#250986=ORIENTED_EDGE ( 'NONE', *, *, #18076, .T. ) ;
#250992=VERTEX_POINT ( 'NONE', #8670 ) ;
#251103=EDGE_LOOP ( 'NONE', ( #67053, #241665, #14046, #45396 ) ) ;
#251144=CARTESIAN_POINT ( 'NONE',  ( -21.04999999999994387, 65.87745128126655914, -37.09527722473000466 ) ) ;
#251170=ORIENTED_EDGE ( 'NONE', *, *, #153983, .F. ) ;
#251225=EDGE_CURVE ( 'NONE', #215142, #170938, #44616, .T. ) ;
#251266=ADVANCED_FACE ( 'NONE', ( #108437 ), #55877, .T. ) ;
#251328=ORIENTED_EDGE ( 'NONE', *, *, #30228, .T. ) ;
#251341=CARTESIAN_POINT ( 'NONE',  ( 5.900000000000060751, 64.75000000001119815, -22.12310748452479103 ) ) ;
#251511=EDGE_CURVE ( 'NONE', #53673, #230960, #85092, .T. ) ;
#251514=DIRECTION ( 'NONE',  ( 1.000000000000000000, 0.000000000000000000, 0.000000000000000000 ) ) ;
#251533=AXIS2_PLACEMENT_3D ( 'NONE', #232296, #15825, #118761 ) ;
#251592=CARTESIAN_POINT ( 'NONE',  ( -23.39999999999994529, 77.83551161375991967, -47.62760213295649692 ) ) ;
#251722=VECTOR ( 'NONE', #179702, 1000.000000000000000 ) ;
#251753=CARTESIAN_POINT ( 'NONE',  ( -21.04999999999994387, 65.19115966511134275, -30.12310748452479103 ) ) ;
#251790=AXIS2_PLACEMENT_3D ( 'NONE', #20063, #141277, #143829 ) ;
#251797=VERTEX_POINT ( 'NONE', #166853 ) ;
#251801=LINE ( 'NONE', #191865, #59401 ) ;
#251897=ORIENTED_EDGE ( 'NONE', *, *, #196253, .F. ) ;
#251948=VERTEX_POINT ( 'NONE', #64824 ) ;
#252133=EDGE_CURVE ( 'NONE', #187434, #77791, #239441, .T. ) ;
#252143=VERTEX_POINT ( 'NONE', #150788 ) ;
#252220=CARTESIAN_POINT ( 'NONE',  ( -21.14999999999994174, 76.00000000001119815, -31.97310748452479601 ) ) ;
#252227=VERTEX_POINT ( 'NONE', #197603 ) ;
#252236=AXIS2_PLACEMENT_3D ( 'NONE', #188086, #9439, #74594 ) ;
#252309=ORIENTED_EDGE ( 'NONE', *, *, #142662, .T. ) ;
#252352=EDGE_LOOP ( 'NONE', ( #95330, #199347, #194449, #92530 ) ) ;
#252357=CARTESIAN_POINT ( 'NONE',  ( 23.50000000000005684, 77.36076146337680370, -43.99645795275012006 ) ) ;
#252376=DIRECTION ( 'NONE',  ( 0.000000000000000000, 0.000000000000000000, -1.000000000000000000 ) ) ;
#252378=SPHERICAL_SURFACE ( 'NONE', #193545, 0.1000000000000000056 ) ;
#252454=DIRECTION ( 'NONE',  ( 0.000000000000000000, 1.000000000000000000, -8.673617379884043361E-16 ) ) ;
#252634=CARTESIAN_POINT ( 'NONE',  ( -21.14999999999994174, 77.16254490893143725, -43.82310748452479743 ) ) ;
#252647=CARTESIAN_POINT ( 'NONE',  ( -21.14999999999994174, 64.35000000001120668, -36.02310748452479316 ) ) ;
#252661=DIRECTION ( 'NONE',  ( -2.568025086422246928E-15, -0.1480365673253023762, 0.9889818879709281196 ) ) ;
#252769=ORIENTED_EDGE ( 'NONE', *, *, #80409, .F. ) ;
#252772=EDGE_CURVE ( 'NONE', #150150, #178868, #6566, .T. ) ;
#252815=CIRCLE ( 'NONE', #132029, 3.970710678118656300 ) ;
#252870=CYLINDRICAL_SURFACE ( 'NONE', #13543, 0.1000000000000028644 ) ;
#252872=EDGE_LOOP ( 'NONE', ( #47251, #188125, #134114, #106900 ) ) ;
#252904=CARTESIAN_POINT ( 'NONE',  ( 23.40000000000005542, 74.63923853664559260, -43.99645795275012006 ) ) ;
#252918=DIRECTION ( 'NONE',  ( -1.000000000000000000, 0.000000000000000000, 0.000000000000000000 ) ) ;
#252928=CIRCLE ( 'NONE', #148719, 0.09999999999999939493 ) ;
#253045=DIRECTION ( 'NONE',  ( 0.000000000000000000, 0.000000000000000000, -1.000000000000000000 ) ) ;
#253067=CIRCLE ( 'NONE', #149049, 0.1000000000000028644 ) ;
#253093=CARTESIAN_POINT ( 'NONE',  ( 11.60000000000006182, 67.75000000001118394, -18.42310748452479530 ) ) ;
#253119=EDGE_CURVE ( 'NONE', #128152, #75854, #48449, .T. ) ;
#253146=ORIENTED_EDGE ( 'NONE', *, *, #179227, .F. ) ;
#253157=DIRECTION ( 'NONE',  ( 1.000000000000000000, -0.000000000000000000, -0.000000000000000000 ) ) ;
#253164=EDGE_CURVE ( 'NONE', #224621, #8217, #159853, .T. ) ;
#253187=EDGE_CURVE ( 'NONE', #184662, #136469, #127566, .T. ) ;
#253219=CARTESIAN_POINT ( 'NONE',  ( 23.50000000000005684, 62.43959356634987046, -37.55748533175129467 ) ) ;
#253231=VECTOR ( 'NONE', #62574, 1000.000000000000000 ) ;
#253270=FACE_OUTER_BOUND ( 'NONE', #230483, .T. ) ;
#253317=CARTESIAN_POINT ( 'NONE',  ( -5.899999999999938183, 64.35000000001120668, -25.92310748452479174 ) ) ;
#253358=EDGE_CURVE ( 'NONE', #107651, #68335, #173008, .T. ) ;
#253379=VERTEX_POINT ( 'NONE', #222342 ) ;
#253381=CIRCLE ( 'NONE', #228453, 0.1000000000000021844 ) ;
#253421=ORIENTED_EDGE ( 'NONE', *, *, #234929, .F. ) ;
#253424=DIRECTION ( 'NONE',  ( 1.000000000000000000, -0.000000000000000000, 0.000000000000000000 ) ) ;
#253462=DIRECTION ( 'NONE',  ( 0.000000000000000000, 0.000000000000000000, 1.000000000000000000 ) ) ;
#253477=ORIENTED_EDGE ( 'NONE', *, *, #213005, .F. ) ;
#253484=EDGE_CURVE ( 'NONE', #12197, #97363, #89274, .T. ) ;
#253496=EDGE_CURVE ( 'NONE', #9346, #64966, #228811, .T. ) ;
#253625=CARTESIAN_POINT ( 'NONE',  ( 20.95000000000005613, 66.15000000001120384, -4.623107484524796362 ) ) ;
#253716=FACE_OUTER_BOUND ( 'NONE', #158929, .T. ) ;
#253788=AXIS2_PLACEMENT_3D ( 'NONE', #255444, #18170, #136826 ) ;
#253824=ORIENTED_EDGE ( 'NONE', *, *, #179917, .T. ) ;
#253828=VERTEX_POINT ( 'NONE', #30307 ) ;
#253833=CARTESIAN_POINT ( 'NONE',  ( -20.94999999999994600, 64.35000000001119247, -5.923107484524795296 ) ) ;
#253841=DIRECTION ( 'NONE',  ( 1.000000000000000000, 0.000000000000000000, 0.000000000000000000 ) ) ;
#253842=ORIENTED_EDGE ( 'NONE', *, *, #99439, .F. ) ;
#253920=EDGE_CURVE ( 'NONE', #201487, #99338, #114894, .T. ) ;
#253974=CIRCLE ( 'NONE', #125016, 0.09999999999999982514 ) ;
#253975=EDGE_CURVE ( 'NONE', #30313, #103754, #157988, .T. ) ;
#253991=ADVANCED_FACE ( 'NONE', ( #114964 ), #22308, .T. ) ;
#254007=CARTESIAN_POINT ( 'NONE',  ( 0.9000000000000547562, 64.35000000001120668, -12.62310748452478926 ) ) ;
#254042=ORIENTED_EDGE ( 'NONE', *, *, #132758, .F. ) ;
#254045=ORIENTED_EDGE ( 'NONE', *, *, #226367, .F. ) ;
#254058=CARTESIAN_POINT ( 'NONE',  ( -23.39999999999994529, 74.15089172278851493, -47.62873275725970501 ) ) ;
#254072=CIRCLE ( 'NONE', #158438, 0.09999999999999982514 ) ;
#254092=CIRCLE ( 'NONE', #95872, 0.09999999999999939493 ) ;
#254113=DIRECTION ( 'NONE',  ( -1.000000000000000000, 0.000000000000000000, 0.000000000000000000 ) ) ;
#254125=PLANE ( 'NONE',  #54028 ) ;
#254159=FACE_BOUND ( 'NONE', #137730, .T. ) ;
#254160=AXIS2_PLACEMENT_3D ( 'NONE', #78786, #94511, #38403 ) ;
#254228=EDGE_CURVE ( 'NONE', #130445, #172317, #69133, .T. ) ;
#254292=CARTESIAN_POINT ( 'NONE',  ( -20.94999999999994600, 61.72892516158560028, -36.56695479651062897 ) ) ;
#254311=EDGE_CURVE ( 'NONE', #135971, #21878, #64995, .T. ) ;
#254314=CARTESIAN_POINT ( 'NONE',  ( 23.40000000000005187, 74.94272479589878344, -3.023107484524792277 ) ) ;
#254360=LINE ( 'NONE', #196966, #82259 ) ;
#254481=DIRECTION ( 'NONE',  ( -0.000000000000000000, 1.000000000000000000, -0.000000000000000000 ) ) ;
#254527=DIRECTION ( 'NONE',  ( 0.000000000000000000, 0.000000000000000000, -1.000000000000000000 ) ) ;
#254554=FACE_OUTER_BOUND ( 'NONE', #158921, .T. ) ;
#254559=EDGE_CURVE ( 'NONE', #151679, #73109, #102749, .T. ) ;
#254600=ORIENTED_EDGE ( 'NONE', *, *, #236566, .T. ) ;
#254763=EDGE_LOOP ( 'NONE', ( #74742, #88056, #253421, #11717 ) ) ;
#254775=CYLINDRICAL_SURFACE ( 'NONE', #21481, 0.09999999999999939493 ) ;
#254800=CARTESIAN_POINT ( 'NONE',  ( -21.14999999999994174, 64.25000000001119815, -5.923107484524795296 ) ) ;
#254827=EDGE_LOOP ( 'NONE', ( #233555, #200459, #108845, #198636 ) ) ;
#254837=LINE ( 'NONE', #84887, #5487 ) ;
#254877=AXIS2_PLACEMENT_3D ( 'NONE', #145828, #186266, #188817 ) ;
#254898=FACE_OUTER_BOUND ( 'NONE', #92827, .T. ) ;
#254946=ORIENTED_EDGE ( 'NONE', *, *, #81032, .T. ) ;
#254976=AXIS2_PLACEMENT_3D ( 'NONE', #257742, #19190, #80404 ) ;
#254995=VECTOR ( 'NONE', #101387, 1000.000000000000000 ) ;
#255073=DIRECTION ( 'NONE',  ( 0.000000000000000000, -1.000000000000000000, 0.000000000000000000 ) ) ;
#255085=DIRECTION ( 'NONE',  ( -0.000000000000000000, 0.8164390028469706850, -0.5774316882803059992 ) ) ;
#255132=VERTEX_POINT ( 'NONE', #181421 ) ;
#255136=FACE_OUTER_BOUND ( 'NONE', #199379, .T. ) ;
#255183=AXIS2_PLACEMENT_3D ( 'NONE', #106353, #175073, #254527 ) ;
#255188=ORIENTED_EDGE ( 'NONE', *, *, #163016, .T. ) ;
#255235=ADVANCED_FACE ( 'NONE', ( #112157 ), #66200, .T. ) ;
#255241=TOROIDAL_SURFACE ( 'NONE', #92990, 0.2000000000000000111, 0.1000000000000000056 ) ;
#255245=ORIENTED_EDGE ( 'NONE', *, *, #138172, .F. ) ;
#255269=CARTESIAN_POINT ( 'NONE',  ( 21.15000000000005187, 76.00000000001119815, -40.07310748452479032 ) ) ;
#255279=ORIENTED_EDGE ( 'NONE', *, *, #26610, .T. ) ;
#255287=FACE_OUTER_BOUND ( 'NONE', #11987, .T. ) ;
#255313=DIRECTION ( 'NONE',  ( -0.000000000000000000, 0.1575546449569960317, 0.9875102702516440623 ) ) ;
#255324=DIRECTION ( 'NONE',  ( -0.000000000000000000, 1.000000000000000000, -0.000000000000000000 ) ) ;
#255326=CARTESIAN_POINT ( 'NONE',  ( -23.49999999999994316, 74.94272479589878344, -3.023107484524792277 ) ) ;
#255338=EDGE_CURVE ( 'NONE', #64966, #109860, #257671, .T. ) ;
#255391=DIRECTION ( 'NONE',  ( 0.000000000000000000, -0.1480365673253065117, 0.9889818879709273425 ) ) ;
#255444=CARTESIAN_POINT ( 'NONE',  ( -0.8999999999999430678, 63.75000000001118394, -10.02310748452479139 ) ) ;
#255450=VECTOR ( 'NONE', #203768, 1000.000000000000000 ) ;
#255504=SPHERICAL_SURFACE ( 'NONE', #158779, 0.1000000000000000056 ) ;
#255535=CARTESIAN_POINT ( 'NONE',  ( -5.899999999999938183, 64.25000000001119815, -22.12310748452479103 ) ) ;
#255555=VECTOR ( 'NONE', #175883, 1000.000000000000000 ) ;
#255632=EDGE_CURVE ( 'NONE', #210105, #148669, #101513, .T. ) ;
#255667=APPLICATION_CONTEXT ( 'automotive_design' ) ;
#255677=AXIS2_PLACEMENT_3D ( 'NONE', #150776, #214588, #92077 ) ;
#255685=CARTESIAN_POINT ( 'NONE',  ( 23.50000000000005684, 84.00000000001119815, -37.18565239344504647 ) ) ;
#255686=ORIENTED_EDGE ( 'NONE', *, *, #113563, .T. ) ;
#255703=VERTEX_POINT ( 'NONE', #166697 ) ;
#255754=CARTESIAN_POINT ( 'NONE',  ( -21.04999999999994387, 84.00000000001119815, -34.86056257560453986 ) ) ;
#255794=DIRECTION ( 'NONE',  ( 0.000000000000000000, -0.000000000000000000, 1.000000000000000000 ) ) ;
#255798=AXIS2_PLACEMENT_3D ( 'NONE', #253093, #54888, #111028 ) ;
#255813=DIRECTION ( 'NONE',  ( 1.000000000000000000, 0.000000000000000000, 0.000000000000000000 ) ) ;
#255839=DIRECTION ( 'NONE',  ( 0.000000000000000000, 0.1575546449569757979, 0.9875102702516471709 ) ) ;
#255869=CARTESIAN_POINT ( 'NONE',  ( -23.49999999999994316, 85.52235250936193722, -34.45408804175119144 ) ) ;
#255872=ORIENTED_EDGE ( 'NONE', *, *, #126501, .T. ) ;
#255878=CARTESIAN_POINT ( 'NONE',  ( 21.15000000000005187, 64.35000000001120668, -5.923107484524795296 ) ) ;
#255896=DIRECTION ( 'NONE',  ( -1.000000000000000000, 0.000000000000000000, 0.000000000000000000 ) ) ;
#255989=EDGE_CURVE ( 'NONE', #189995, #133767, #196972, .T. ) ;
#256024=FACE_OUTER_BOUND ( 'NONE', #210422, .T. ) ;
#256026=LINE ( 'NONE', #54030, #32827 ) ;
#256069=ORIENTED_EDGE ( 'NONE', *, *, #170782, .F. ) ;
#256076=DIRECTION ( 'NONE',  ( 0.000000000000000000, -1.000000000000000000, 0.000000000000000000 ) ) ;
#256079=EDGE_CURVE ( 'NONE', #168532, #211446, #138675, .T. ) ;
#256126=DIRECTION ( 'NONE',  ( -0.000000000000000000, -0.1332476588733589318, -0.9910827722268049644 ) ) ;
#256130=LINE ( 'NONE', #65703, #112980 ) ;
#256144=CARTESIAN_POINT ( 'NONE',  ( 5.900000000000059863, 64.65000000001120384, -26.02310748452479316 ) ) ;
#256151=AXIS2_PLACEMENT_3D ( 'NONE', #48011, #109262, #28507 ) ;
#256171=CARTESIAN_POINT ( 'NONE',  ( 20.95000000000005258, 64.35000000001119247, -6.023107484524794941 ) ) ;
#256293=DIRECTION ( 'NONE',  ( 0.000000000000000000, 0.000000000000000000, 1.000000000000000000 ) ) ;
#256310=FACE_BOUND ( 'NONE', #148154, .T. ) ;
#256367=DIRECTION ( 'NONE',  ( 0.000000000000000000, -0.1332476588733448597, -0.9910827722268067408 ) ) ;
#256410=CARTESIAN_POINT ( 'NONE',  ( -21.14999999999994174, 83.90000000001120384, -34.86056257560453986 ) ) ;
#256458=EDGE_CURVE ( 'NONE', #75854, #202553, #238861, .T. ) ;
#256478=CIRCLE ( 'NONE', #144092, 0.1999999999999987899 ) ;
#256484=AXIS2_PLACEMENT_3D ( 'NONE', #257584, #120736, #256293 ) ;
#256487=DIRECTION ( 'NONE',  ( 1.000000000000000000, -0.000000000000000000, -0.000000000000000000 ) ) ;
#256501=LINE ( 'NONE', #197868, #139606 ) ;
#256507=CIRCLE ( 'NONE', #248382, 0.09999999999999982514 ) ;
#256509=ORIENTED_EDGE ( 'NONE', *, *, #67024, .F. ) ;
#256542=VERTEX_POINT ( 'NONE', #97570 ) ;
#256582=FACE_OUTER_BOUND ( 'NONE', #97934, .T. ) ;
#256615=EDGE_CURVE ( 'NONE', #33086, #90057, #228143, .T. ) ;
#256617=ORIENTED_EDGE ( 'NONE', *, *, #193789, .T. ) ;
#256622=DIRECTION ( 'NONE',  ( 0.000000000000000000, 0.000000000000000000, -1.000000000000000000 ) ) ;
#256627=FACE_OUTER_BOUND ( 'NONE', #47931, .T. ) ;
#256632=DIRECTION ( 'NONE',  ( 0.000000000000000000, 0.000000000000000000, -1.000000000000000000 ) ) ;
#256722=DIRECTION ( 'NONE',  ( -0.000000000000000000, 1.000000000000000000, -0.000000000000000000 ) ) ;
#256729=ORIENTED_EDGE ( 'NONE', *, *, #50299, .T. ) ;
#256769=ORIENTED_EDGE ( 'NONE', *, *, #242076, .T. ) ;
#256776=AXIS2_PLACEMENT_3D ( 'NONE', #10936, #55150, #214264 ) ;
#256781=EDGE_CURVE ( 'NONE', #143932, #244869, #55882, .T. ) ;
#256813=ORIENTED_EDGE ( 'NONE', *, *, #99644, .F. ) ;
#256852=CARTESIAN_POINT ( 'NONE',  ( -11.59999999999994458, 64.25000000001119815, -18.32310748452479388 ) ) ;
#256961=LINE ( 'NONE', #181349, #67497 ) ;
#256974=DIRECTION ( 'NONE',  ( 3.469446951953515108E-14, 0.000000000000000000, 1.000000000000000000 ) ) ;
#257093=CARTESIAN_POINT ( 'NONE',  ( -23.39999999999994529, 83.80000000001119531, -34.77310748452479316 ) ) ;
#257183=VECTOR ( 'NONE', #50086, 1000.000000000000000 ) ;
#257189=AXIS2_PLACEMENT_3D ( 'NONE', #83830, #180417, #5596 ) ;
#257231=ORIENTED_EDGE ( 'NONE', *, *, #256079, .T. ) ;
#257250=ORIENTED_EDGE ( 'NONE', *, *, #56475, .F. ) ;
#257277=DIRECTION ( 'NONE',  ( 1.000000000000000000, 0.000000000000000000, 0.000000000000000000 ) ) ;
#257282=VERTEX_POINT ( 'NONE', #20353 ) ;
#257333=DIRECTION ( 'NONE',  ( 0.000000000000000000, 0.000000000000000000, -1.000000000000000000 ) ) ;
#257359=DIRECTION ( 'NONE',  ( 0.000000000000000000, 0.000000000000000000, -1.000000000000000000 ) ) ;
#257385=CARTESIAN_POINT ( 'NONE',  ( -20.94999999999994600, 66.15000000001120384, -4.623107484524796362 ) ) ;
#257425=DIRECTION ( 'NONE',  ( 0.000000000000000000, 0.000000000000000000, -1.000000000000000000 ) ) ;
#257441=ORIENTED_EDGE ( 'NONE', *, *, #113563, .F. ) ;
#257443=LINE ( 'NONE', #140105, #5887 ) ;
#257489=CIRCLE ( 'NONE', #232454, 0.1000000000000021844 ) ;
#257500=EDGE_CURVE ( 'NONE', #161732, #20544, #201800, .T. ) ;
#257584=CARTESIAN_POINT ( 'NONE',  ( 21.05000000000005400, 76.00000000001119815, -36.02310748452479316 ) ) ;
#257608=FACE_OUTER_BOUND ( 'NONE', #21305, .T. ) ;
#257671=CIRCLE ( 'NONE', #191133, 0.09999999999999939493 ) ;
#257680=ORIENTED_EDGE ( 'NONE', *, *, #719, .T. ) ;
#257682=LINE ( 'NONE', #3403, #142056 ) ;
#257709=ADVANCED_FACE ( 'NONE', ( #127800 ), #30001, .T. ) ;
#257733=EDGE_CURVE ( 'NONE', #111921, #69129, #52082, .T. ) ;
#257742=CARTESIAN_POINT ( 'NONE',  ( -23.39999999999994529, 84.00000000001119815, -34.86056257560453986 ) ) ;
#257753=CARTESIAN_POINT ( 'NONE',  ( -5.999999999999938716, 64.35000000001120668, -25.92310748452479174 ) ) ;
#257813=ORIENTED_EDGE ( 'NONE', *, *, #138665, .F. ) ;
#257821=DIRECTION ( 'NONE',  ( 0.000000000000000000, 0.000000000000000000, 1.000000000000000000 ) ) ;
#257856=CIRCLE ( 'NONE', #228715, 0.09999999999999939493 ) ;
#257915=ORIENTED_EDGE ( 'NONE', *, *, #144006, .T. ) ;
#257916=EDGE_CURVE ( 'NONE', #100189, #113855, #215023, .T. ) ;
#257949=ADVANCED_FACE ( 'NONE', ( #105304 ), #206276, .T. ) ;
#258012=FACE_OUTER_BOUND ( 'NONE', #141656, .T. ) ;
#258019=DIRECTION ( 'NONE',  ( -1.000000000000000000, 0.000000000000000000, 0.000000000000000000 ) ) ;
#258020=ADVANCED_FACE ( 'NONE', ( #24550 ), #162772, .F. ) ;
#258021=ADVANCED_FACE ( 'NONE', ( #140614 ), #104035, .T. ) ;
#258042=CARTESIAN_POINT ( 'NONE',  ( -21.14999999999994174, 77.16254490893143725, -44.02310748452479316 ) ) ;
#258073=ORIENTED_EDGE ( 'NONE', *, *, #254559, .T. ) ;
ENDSEC;
END-ISO-10303-21;
